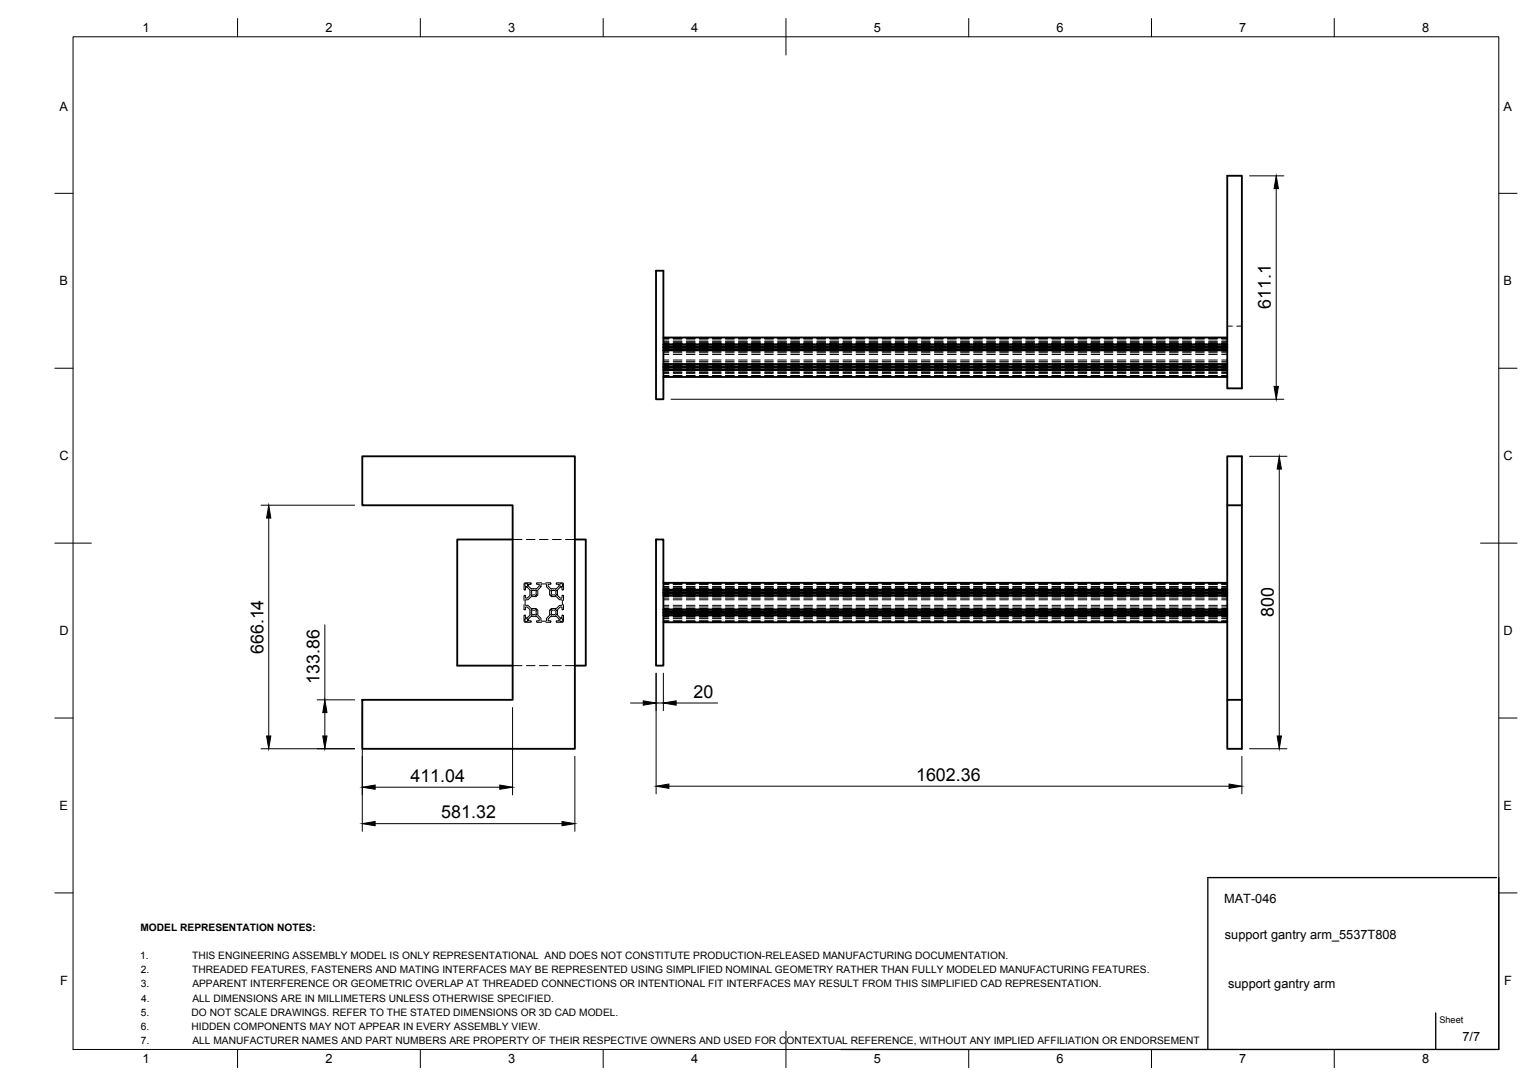
ISO-10303-21;
HEADER;
/* Generated by software containing ST-Developer
 * from STEP Tools, Inc. (www.steptools.com) 
 */

FILE_DESCRIPTION(
/* description */ ('STEP AP214'),
/* implementation_level */ '2;1');

FILE_NAME(
/* name */ 'support gantry arm.step',
/* time_stamp */ '2026-11-14T22:16:48-08:00',
/* author */ (''),
/* organization */ (''),
/* preprocessor_version */ 'ST-DEVELOPER v20.2',
/* originating_system */ 'Autodesk Translation Framework v15.17.0.0',
/* authorisation */ '');

FILE_SCHEMA (('AUTOMOTIVE_DESIGN { 1 0 10303 214 3 1 1 }'));
ENDSEC;

DATA;
#10=MECHANICAL_DESIGN_GEOMETRIC_PRESENTATION_REPRESENTATION('',(#5500),#276462);
#35=ORIENTED_CLOSED_SHELL('',*,#98725,.F.);
#36=ORIENTED_CLOSED_SHELL('',*,#98726,.F.);
#37=ORIENTED_CLOSED_SHELL('',*,#98727,.F.);
#38=ORIENTED_CLOSED_SHELL('',*,#98728,.F.);
#39=ORIENTED_CLOSED_SHELL('',*,#98729,.F.);
#40=ORIENTED_CLOSED_SHELL('',*,#98730,.F.);
#41=ORIENTED_CLOSED_SHELL('',*,#98731,.F.);
#42=ORIENTED_CLOSED_SHELL('',*,#98732,.F.);
#43=ORIENTED_CLOSED_SHELL('',*,#98733,.F.);
#44=BREP_WITH_VOIDS('Body1',#98734,(#35,#36,#37,#38,#39,#40,#41,#42,#43));
#5465=SHAPE_REPRESENTATION_RELATIONSHIP('SRR','None',#276493,#5471);
#5471=ADVANCED_BREP_SHAPE_REPRESENTATION('',(#44),#276461);
#5500=STYLED_ITEM('',(#276527),#44);
#6444=FACE_BOUND('',#19950,.T.);
#6445=FACE_BOUND('',#19956,.T.);
#7354=PLANE('',#110990);
#7355=PLANE('',#110998);
#7356=PLANE('',#110999);
#7357=PLANE('',#111002);
#7358=PLANE('',#111005);
#7359=PLANE('',#111008);
#7360=PLANE('',#111011);
#7361=PLANE('',#111014);
#7362=PLANE('',#111017);
#7363=PLANE('',#111020);
#7364=PLANE('',#111021);
#7365=PLANE('',#111026);
#7366=PLANE('',#111029);
#7367=PLANE('',#111032);
#7368=PLANE('',#111035);
#7369=PLANE('',#111038);
#7370=PLANE('',#111039);
#7371=PLANE('',#111064);
#7372=PLANE('',#111090);
#7373=PLANE('',#111092);
#7374=PLANE('',#111094);
#7375=PLANE('',#111095);
#7376=PLANE('',#111096);
#7377=PLANE('',#111098);
#7378=PLANE('',#111100);
#7379=PLANE('',#111102);
#7380=PLANE('',#111104);
#7381=PLANE('',#111106);
#7382=PLANE('',#111108);
#7383=PLANE('',#111109);
#7384=PLANE('',#111110);
#7385=PLANE('',#111112);
#7386=PLANE('',#111114);
#7387=PLANE('',#111116);
#7388=PLANE('',#111118);
#7389=PLANE('',#111120);
#7390=PLANE('',#111122);
#7391=PLANE('',#111123);
#7392=PLANE('',#111124);
#7393=PLANE('',#111126);
#7394=PLANE('',#111128);
#7395=PLANE('',#111130);
#7396=PLANE('',#111132);
#7397=PLANE('',#111134);
#7398=PLANE('',#111136);
#7399=PLANE('',#111137);
#7400=PLANE('',#111138);
#7401=PLANE('',#111140);
#7402=PLANE('',#111142);
#7403=PLANE('',#111144);
#7404=PLANE('',#111148);
#7405=PLANE('',#111156);
#7406=PLANE('',#111159);
#7407=PLANE('',#111162);
#7408=PLANE('',#111165);
#7409=PLANE('',#111168);
#7410=PLANE('',#111169);
#7411=PLANE('',#111172);
#7412=PLANE('',#111175);
#7413=PLANE('',#111178);
#7414=PLANE('',#111179);
#7415=PLANE('',#111184);
#7416=PLANE('',#111187);
#7417=PLANE('',#111190);
#7418=PLANE('',#111193);
#7419=PLANE('',#111196);
#7420=PLANE('',#111200);
#7421=PLANE('',#111208);
#7422=PLANE('',#111211);
#7423=PLANE('',#111214);
#7424=PLANE('',#111217);
#7425=PLANE('',#111220);
#7426=PLANE('',#111223);
#7427=PLANE('',#111226);
#7428=PLANE('',#111227);
#7429=PLANE('',#111230);
#7430=PLANE('',#111231);
#7431=PLANE('',#111236);
#7432=PLANE('',#111239);
#7433=PLANE('',#111242);
#7434=PLANE('',#111245);
#7435=PLANE('',#111248);
#7436=PLANE('',#111252);
#7437=PLANE('',#111260);
#7438=PLANE('',#111263);
#7439=PLANE('',#111266);
#7440=PLANE('',#111269);
#7441=PLANE('',#111272);
#7442=PLANE('',#111275);
#7443=PLANE('',#111278);
#7444=PLANE('',#111279);
#7445=PLANE('',#111282);
#7446=PLANE('',#111283);
#7447=PLANE('',#111288);
#7448=PLANE('',#111291);
#7449=PLANE('',#111294);
#7450=PLANE('',#111297);
#7451=PLANE('',#111300);
#7452=PLANE('',#111301);
#7453=PLANE('',#111302);
#7454=PLANE('',#111303);
#7455=PLANE('',#111304);
#7456=PLANE('',#111305);
#7457=PLANE('',#111309);
#7458=PLANE('',#111313);
#7459=PLANE('',#111317);
#7460=PLANE('',#111321);
#7461=PLANE('',#111322);
#7462=PLANE('',#111323);
#7463=PLANE('',#111324);
#7464=PLANE('',#111325);
#7465=PLANE('',#111326);
#7466=PLANE('',#111327);
#7467=PLANE('',#111328);
#7468=PLANE('',#111332);
#7469=PLANE('',#111336);
#7470=PLANE('',#111340);
#7471=PLANE('',#111344);
#7472=PLANE('',#111345);
#7473=PLANE('',#111346);
#7474=PLANE('',#111347);
#7475=PLANE('',#111351);
#7476=PLANE('',#111355);
#7477=PLANE('',#111359);
#7478=PLANE('',#111363);
#7479=PLANE('',#111364);
#7480=PLANE('',#111365);
#7481=PLANE('',#111366);
#7482=PLANE('',#111370);
#7483=PLANE('',#111371);
#7484=PLANE('',#111372);
#7485=PLANE('',#111373);
#7486=PLANE('',#111377);
#7487=PLANE('',#111381);
#7488=PLANE('',#111385);
#7489=PLANE('',#111389);
#7490=PLANE('',#111390);
#7491=PLANE('',#111391);
#7492=PLANE('',#111392);
#7493=PLANE('',#111396);
#7494=PLANE('',#111400);
#7495=PLANE('',#111404);
#7496=PLANE('',#111408);
#7497=PLANE('',#111409);
#7498=PLANE('',#111410);
#7499=PLANE('',#111411);
#7500=PLANE('',#111412);
#7501=PLANE('',#111413);
#7502=PLANE('',#111414);
#7503=PLANE('',#111418);
#7504=PLANE('',#111422);
#7505=PLANE('',#111426);
#7506=PLANE('',#111430);
#7507=PLANE('',#111431);
#7508=PLANE('',#111432);
#7509=PLANE('',#111433);
#7510=PLANE('',#111437);
#7511=PLANE('',#111441);
#7512=PLANE('',#111445);
#7513=PLANE('',#111449);
#7514=PLANE('',#111450);
#7515=PLANE('',#111451);
#7516=PLANE('',#111452);
#7517=PLANE('',#111456);
#7518=PLANE('',#111457);
#7519=PLANE('',#111458);
#7520=PLANE('',#111459);
#7521=PLANE('',#111463);
#7522=PLANE('',#111467);
#7523=PLANE('',#111471);
#7524=PLANE('',#111475);
#7525=PLANE('',#111476);
#7526=PLANE('',#111477);
#7527=PLANE('',#111478);
#7528=PLANE('',#111482);
#7529=PLANE('',#111486);
#7530=PLANE('',#111490);
#7531=PLANE('',#111494);
#7532=PLANE('',#111495);
#7533=PLANE('',#111496);
#7534=PLANE('',#111497);
#7535=PLANE('',#111498);
#7536=PLANE('',#111499);
#7537=PLANE('',#111500);
#7538=PLANE('',#111504);
#7539=PLANE('',#111508);
#7540=PLANE('',#111512);
#7541=PLANE('',#111516);
#7542=PLANE('',#111517);
#7543=PLANE('',#111518);
#7544=PLANE('',#111519);
#7545=PLANE('',#111523);
#7546=PLANE('',#111527);
#7547=PLANE('',#111531);
#7548=PLANE('',#111535);
#7549=PLANE('',#111536);
#7550=PLANE('',#111537);
#7551=PLANE('',#111538);
#7552=PLANE('',#111542);
#7553=PLANE('',#111543);
#7554=PLANE('',#111544);
#7555=PLANE('',#111545);
#7556=PLANE('',#111549);
#7557=PLANE('',#111553);
#7558=PLANE('',#111557);
#7559=PLANE('',#111561);
#7560=PLANE('',#111562);
#7561=PLANE('',#111563);
#7562=PLANE('',#111564);
#7563=PLANE('',#111568);
#7564=PLANE('',#111572);
#7565=PLANE('',#111576);
#7566=PLANE('',#111580);
#7567=PLANE('',#111581);
#7568=PLANE('',#111582);
#7569=PLANE('',#111583);
#7570=PLANE('',#111584);
#7571=PLANE('',#111585);
#7572=PLANE('',#111589);
#7573=PLANE('',#111593);
#7574=PLANE('',#111597);
#7575=PLANE('',#111601);
#7576=PLANE('',#111602);
#7577=PLANE('',#111603);
#7578=PLANE('',#111604);
#7579=PLANE('',#111608);
#7580=PLANE('',#111612);
#7581=PLANE('',#111616);
#7582=PLANE('',#111620);
#7583=PLANE('',#111621);
#7584=PLANE('',#111622);
#7585=PLANE('',#111623);
#7586=PLANE('',#111627);
#7587=PLANE('',#111628);
#7588=PLANE('',#111629);
#7589=PLANE('',#111630);
#7590=PLANE('',#111634);
#7591=PLANE('',#111638);
#7592=PLANE('',#111642);
#7593=PLANE('',#111646);
#7594=PLANE('',#111647);
#7595=PLANE('',#111648);
#7596=PLANE('',#111649);
#7597=PLANE('',#111650);
#7598=PLANE('',#111651);
#7599=PLANE('',#111652);
#7600=PLANE('',#111653);
#7601=PLANE('',#111654);
#7602=PLANE('',#111655);
#7603=PLANE('',#111656);
#7604=PLANE('',#111657);
#7605=PLANE('',#111658);
#7606=PLANE('',#111659);
#7607=PLANE('',#111660);
#7608=PLANE('',#111661);
#7609=PLANE('',#111662);
#7610=PLANE('',#111663);
#7611=PLANE('',#111664);
#7612=PLANE('',#111665);
#7613=PLANE('',#111666);
#13324=FACE_OUTER_BOUND('',#19556,.T.);
#13325=FACE_OUTER_BOUND('',#19557,.T.);
#13326=FACE_OUTER_BOUND('',#19558,.T.);
#13327=FACE_OUTER_BOUND('',#19559,.T.);
#13328=FACE_OUTER_BOUND('',#19560,.T.);
#13329=FACE_OUTER_BOUND('',#19561,.T.);
#13330=FACE_OUTER_BOUND('',#19562,.T.);
#13331=FACE_OUTER_BOUND('',#19563,.T.);
#13332=FACE_OUTER_BOUND('',#19564,.T.);
#13333=FACE_OUTER_BOUND('',#19565,.T.);
#13334=FACE_OUTER_BOUND('',#19566,.T.);
#13335=FACE_OUTER_BOUND('',#19567,.T.);
#13336=FACE_OUTER_BOUND('',#19568,.T.);
#13337=FACE_OUTER_BOUND('',#19569,.T.);
#13338=FACE_OUTER_BOUND('',#19570,.T.);
#13339=FACE_OUTER_BOUND('',#19571,.T.);
#13340=FACE_OUTER_BOUND('',#19572,.T.);
#13341=FACE_OUTER_BOUND('',#19573,.T.);
#13342=FACE_OUTER_BOUND('',#19574,.T.);
#13343=FACE_OUTER_BOUND('',#19575,.T.);
#13344=FACE_OUTER_BOUND('',#19576,.T.);
#13345=FACE_OUTER_BOUND('',#19577,.T.);
#13346=FACE_OUTER_BOUND('',#19578,.T.);
#13347=FACE_OUTER_BOUND('',#19579,.T.);
#13348=FACE_OUTER_BOUND('',#19580,.T.);
#13349=FACE_OUTER_BOUND('',#19581,.T.);
#13350=FACE_OUTER_BOUND('',#19582,.T.);
#13351=FACE_OUTER_BOUND('',#19583,.T.);
#13352=FACE_OUTER_BOUND('',#19584,.T.);
#13353=FACE_OUTER_BOUND('',#19585,.T.);
#13354=FACE_OUTER_BOUND('',#19586,.T.);
#13355=FACE_OUTER_BOUND('',#19587,.T.);
#13356=FACE_OUTER_BOUND('',#19588,.T.);
#13357=FACE_OUTER_BOUND('',#19589,.T.);
#13358=FACE_OUTER_BOUND('',#19590,.T.);
#13359=FACE_OUTER_BOUND('',#19591,.T.);
#13360=FACE_OUTER_BOUND('',#19592,.T.);
#13361=FACE_OUTER_BOUND('',#19593,.T.);
#13362=FACE_OUTER_BOUND('',#19594,.T.);
#13363=FACE_OUTER_BOUND('',#19595,.T.);
#13364=FACE_OUTER_BOUND('',#19596,.T.);
#13365=FACE_OUTER_BOUND('',#19597,.T.);
#13366=FACE_OUTER_BOUND('',#19598,.T.);
#13367=FACE_OUTER_BOUND('',#19599,.T.);
#13368=FACE_OUTER_BOUND('',#19600,.T.);
#13369=FACE_OUTER_BOUND('',#19601,.T.);
#13370=FACE_OUTER_BOUND('',#19602,.T.);
#13371=FACE_OUTER_BOUND('',#19603,.T.);
#13372=FACE_OUTER_BOUND('',#19604,.T.);
#13373=FACE_OUTER_BOUND('',#19605,.T.);
#13374=FACE_OUTER_BOUND('',#19606,.T.);
#13375=FACE_OUTER_BOUND('',#19607,.T.);
#13376=FACE_OUTER_BOUND('',#19608,.T.);
#13377=FACE_OUTER_BOUND('',#19609,.T.);
#13378=FACE_OUTER_BOUND('',#19610,.T.);
#13379=FACE_OUTER_BOUND('',#19611,.T.);
#13380=FACE_OUTER_BOUND('',#19612,.T.);
#13381=FACE_OUTER_BOUND('',#19613,.T.);
#13382=FACE_OUTER_BOUND('',#19614,.T.);
#13383=FACE_OUTER_BOUND('',#19615,.T.);
#13384=FACE_OUTER_BOUND('',#19616,.T.);
#13385=FACE_OUTER_BOUND('',#19617,.T.);
#13386=FACE_OUTER_BOUND('',#19618,.T.);
#13387=FACE_OUTER_BOUND('',#19619,.T.);
#13388=FACE_OUTER_BOUND('',#19620,.T.);
#13389=FACE_OUTER_BOUND('',#19621,.T.);
#13390=FACE_OUTER_BOUND('',#19622,.T.);
#13391=FACE_OUTER_BOUND('',#19623,.T.);
#13392=FACE_OUTER_BOUND('',#19624,.T.);
#13393=FACE_OUTER_BOUND('',#19625,.T.);
#13394=FACE_OUTER_BOUND('',#19626,.T.);
#13395=FACE_OUTER_BOUND('',#19627,.T.);
#13396=FACE_OUTER_BOUND('',#19628,.T.);
#13397=FACE_OUTER_BOUND('',#19629,.T.);
#13398=FACE_OUTER_BOUND('',#19630,.T.);
#13399=FACE_OUTER_BOUND('',#19631,.T.);
#13400=FACE_OUTER_BOUND('',#19632,.T.);
#13401=FACE_OUTER_BOUND('',#19633,.T.);
#13402=FACE_OUTER_BOUND('',#19634,.T.);
#13403=FACE_OUTER_BOUND('',#19635,.T.);
#13404=FACE_OUTER_BOUND('',#19636,.T.);
#13405=FACE_OUTER_BOUND('',#19637,.T.);
#13406=FACE_OUTER_BOUND('',#19638,.T.);
#13407=FACE_OUTER_BOUND('',#19639,.T.);
#13408=FACE_OUTER_BOUND('',#19640,.T.);
#13409=FACE_OUTER_BOUND('',#19641,.T.);
#13410=FACE_OUTER_BOUND('',#19642,.T.);
#13411=FACE_OUTER_BOUND('',#19643,.T.);
#13412=FACE_OUTER_BOUND('',#19644,.T.);
#13413=FACE_OUTER_BOUND('',#19645,.T.);
#13414=FACE_OUTER_BOUND('',#19646,.T.);
#13415=FACE_OUTER_BOUND('',#19647,.T.);
#13416=FACE_OUTER_BOUND('',#19648,.T.);
#13417=FACE_OUTER_BOUND('',#19649,.T.);
#13418=FACE_OUTER_BOUND('',#19650,.T.);
#13419=FACE_OUTER_BOUND('',#19651,.T.);
#13420=FACE_OUTER_BOUND('',#19652,.T.);
#13421=FACE_OUTER_BOUND('',#19653,.T.);
#13422=FACE_OUTER_BOUND('',#19654,.T.);
#13423=FACE_OUTER_BOUND('',#19655,.T.);
#13424=FACE_OUTER_BOUND('',#19656,.T.);
#13425=FACE_OUTER_BOUND('',#19657,.T.);
#13426=FACE_OUTER_BOUND('',#19658,.T.);
#13427=FACE_OUTER_BOUND('',#19659,.T.);
#13428=FACE_OUTER_BOUND('',#19660,.T.);
#13429=FACE_OUTER_BOUND('',#19661,.T.);
#13430=FACE_OUTER_BOUND('',#19662,.T.);
#13431=FACE_OUTER_BOUND('',#19663,.T.);
#13432=FACE_OUTER_BOUND('',#19664,.T.);
#13433=FACE_OUTER_BOUND('',#19665,.T.);
#13434=FACE_OUTER_BOUND('',#19666,.T.);
#13435=FACE_OUTER_BOUND('',#19667,.T.);
#13436=FACE_OUTER_BOUND('',#19668,.T.);
#13437=FACE_OUTER_BOUND('',#19669,.T.);
#13438=FACE_OUTER_BOUND('',#19670,.T.);
#13439=FACE_OUTER_BOUND('',#19671,.T.);
#13440=FACE_OUTER_BOUND('',#19672,.T.);
#13441=FACE_OUTER_BOUND('',#19673,.T.);
#13442=FACE_OUTER_BOUND('',#19674,.T.);
#13443=FACE_OUTER_BOUND('',#19675,.T.);
#13444=FACE_OUTER_BOUND('',#19676,.T.);
#13445=FACE_OUTER_BOUND('',#19677,.T.);
#13446=FACE_OUTER_BOUND('',#19678,.T.);
#13447=FACE_OUTER_BOUND('',#19679,.T.);
#13448=FACE_OUTER_BOUND('',#19680,.T.);
#13449=FACE_OUTER_BOUND('',#19681,.T.);
#13450=FACE_OUTER_BOUND('',#19682,.T.);
#13451=FACE_OUTER_BOUND('',#19683,.T.);
#13452=FACE_OUTER_BOUND('',#19684,.T.);
#13453=FACE_OUTER_BOUND('',#19685,.T.);
#13454=FACE_OUTER_BOUND('',#19686,.T.);
#13455=FACE_OUTER_BOUND('',#19687,.T.);
#13456=FACE_OUTER_BOUND('',#19688,.T.);
#13457=FACE_OUTER_BOUND('',#19689,.T.);
#13458=FACE_OUTER_BOUND('',#19690,.T.);
#13459=FACE_OUTER_BOUND('',#19691,.T.);
#13460=FACE_OUTER_BOUND('',#19692,.T.);
#13461=FACE_OUTER_BOUND('',#19693,.T.);
#13462=FACE_OUTER_BOUND('',#19694,.T.);
#13463=FACE_OUTER_BOUND('',#19695,.T.);
#13464=FACE_OUTER_BOUND('',#19696,.T.);
#13465=FACE_OUTER_BOUND('',#19697,.T.);
#13466=FACE_OUTER_BOUND('',#19698,.T.);
#13467=FACE_OUTER_BOUND('',#19699,.T.);
#13468=FACE_OUTER_BOUND('',#19700,.T.);
#13469=FACE_OUTER_BOUND('',#19701,.T.);
#13470=FACE_OUTER_BOUND('',#19702,.T.);
#13471=FACE_OUTER_BOUND('',#19703,.T.);
#13472=FACE_OUTER_BOUND('',#19704,.T.);
#13473=FACE_OUTER_BOUND('',#19705,.T.);
#13474=FACE_OUTER_BOUND('',#19706,.T.);
#13475=FACE_OUTER_BOUND('',#19707,.T.);
#13476=FACE_OUTER_BOUND('',#19708,.T.);
#13477=FACE_OUTER_BOUND('',#19709,.T.);
#13478=FACE_OUTER_BOUND('',#19710,.T.);
#13479=FACE_OUTER_BOUND('',#19711,.T.);
#13480=FACE_OUTER_BOUND('',#19712,.T.);
#13481=FACE_OUTER_BOUND('',#19713,.T.);
#13482=FACE_OUTER_BOUND('',#19714,.T.);
#13483=FACE_OUTER_BOUND('',#19715,.T.);
#13484=FACE_OUTER_BOUND('',#19716,.T.);
#13485=FACE_OUTER_BOUND('',#19717,.T.);
#13486=FACE_OUTER_BOUND('',#19718,.T.);
#13487=FACE_OUTER_BOUND('',#19719,.T.);
#13488=FACE_OUTER_BOUND('',#19720,.T.);
#13489=FACE_OUTER_BOUND('',#19721,.T.);
#13490=FACE_OUTER_BOUND('',#19722,.T.);
#13491=FACE_OUTER_BOUND('',#19723,.T.);
#13492=FACE_OUTER_BOUND('',#19724,.T.);
#13493=FACE_OUTER_BOUND('',#19725,.T.);
#13494=FACE_OUTER_BOUND('',#19726,.T.);
#13495=FACE_OUTER_BOUND('',#19727,.T.);
#13496=FACE_OUTER_BOUND('',#19728,.T.);
#13497=FACE_OUTER_BOUND('',#19729,.T.);
#13498=FACE_OUTER_BOUND('',#19730,.T.);
#13499=FACE_OUTER_BOUND('',#19731,.T.);
#13500=FACE_OUTER_BOUND('',#19732,.T.);
#13501=FACE_OUTER_BOUND('',#19733,.T.);
#13502=FACE_OUTER_BOUND('',#19734,.T.);
#13503=FACE_OUTER_BOUND('',#19735,.T.);
#13504=FACE_OUTER_BOUND('',#19736,.T.);
#13505=FACE_OUTER_BOUND('',#19737,.T.);
#13506=FACE_OUTER_BOUND('',#19738,.T.);
#13507=FACE_OUTER_BOUND('',#19739,.T.);
#13508=FACE_OUTER_BOUND('',#19740,.T.);
#13509=FACE_OUTER_BOUND('',#19741,.T.);
#13510=FACE_OUTER_BOUND('',#19742,.T.);
#13511=FACE_OUTER_BOUND('',#19743,.T.);
#13512=FACE_OUTER_BOUND('',#19744,.T.);
#13513=FACE_OUTER_BOUND('',#19745,.T.);
#13514=FACE_OUTER_BOUND('',#19746,.T.);
#13515=FACE_OUTER_BOUND('',#19747,.T.);
#13516=FACE_OUTER_BOUND('',#19748,.T.);
#13517=FACE_OUTER_BOUND('',#19749,.T.);
#13518=FACE_OUTER_BOUND('',#19750,.T.);
#13519=FACE_OUTER_BOUND('',#19751,.T.);
#13520=FACE_OUTER_BOUND('',#19752,.T.);
#13521=FACE_OUTER_BOUND('',#19753,.T.);
#13522=FACE_OUTER_BOUND('',#19754,.T.);
#13523=FACE_OUTER_BOUND('',#19755,.T.);
#13524=FACE_OUTER_BOUND('',#19756,.T.);
#13525=FACE_OUTER_BOUND('',#19757,.T.);
#13526=FACE_OUTER_BOUND('',#19758,.T.);
#13527=FACE_OUTER_BOUND('',#19759,.T.);
#13528=FACE_OUTER_BOUND('',#19760,.T.);
#13529=FACE_OUTER_BOUND('',#19761,.T.);
#13530=FACE_OUTER_BOUND('',#19762,.T.);
#13531=FACE_OUTER_BOUND('',#19763,.T.);
#13532=FACE_OUTER_BOUND('',#19764,.T.);
#13533=FACE_OUTER_BOUND('',#19765,.T.);
#13534=FACE_OUTER_BOUND('',#19766,.T.);
#13535=FACE_OUTER_BOUND('',#19767,.T.);
#13536=FACE_OUTER_BOUND('',#19768,.T.);
#13537=FACE_OUTER_BOUND('',#19769,.T.);
#13538=FACE_OUTER_BOUND('',#19770,.T.);
#13539=FACE_OUTER_BOUND('',#19771,.T.);
#13540=FACE_OUTER_BOUND('',#19772,.T.);
#13541=FACE_OUTER_BOUND('',#19773,.T.);
#13542=FACE_OUTER_BOUND('',#19774,.T.);
#13543=FACE_OUTER_BOUND('',#19775,.T.);
#13544=FACE_OUTER_BOUND('',#19776,.T.);
#13545=FACE_OUTER_BOUND('',#19777,.T.);
#13546=FACE_OUTER_BOUND('',#19778,.T.);
#13547=FACE_OUTER_BOUND('',#19779,.T.);
#13548=FACE_OUTER_BOUND('',#19780,.T.);
#13549=FACE_OUTER_BOUND('',#19781,.T.);
#13550=FACE_OUTER_BOUND('',#19782,.T.);
#13551=FACE_OUTER_BOUND('',#19783,.T.);
#13552=FACE_OUTER_BOUND('',#19784,.T.);
#13553=FACE_OUTER_BOUND('',#19785,.T.);
#13554=FACE_OUTER_BOUND('',#19786,.T.);
#13555=FACE_OUTER_BOUND('',#19787,.T.);
#13556=FACE_OUTER_BOUND('',#19788,.T.);
#13557=FACE_OUTER_BOUND('',#19789,.T.);
#13558=FACE_OUTER_BOUND('',#19790,.T.);
#13559=FACE_OUTER_BOUND('',#19791,.T.);
#13560=FACE_OUTER_BOUND('',#19792,.T.);
#13561=FACE_OUTER_BOUND('',#19793,.T.);
#13562=FACE_OUTER_BOUND('',#19794,.T.);
#13563=FACE_OUTER_BOUND('',#19795,.T.);
#13564=FACE_OUTER_BOUND('',#19796,.T.);
#13565=FACE_OUTER_BOUND('',#19797,.T.);
#13566=FACE_OUTER_BOUND('',#19798,.T.);
#13567=FACE_OUTER_BOUND('',#19799,.T.);
#13568=FACE_OUTER_BOUND('',#19800,.T.);
#13569=FACE_OUTER_BOUND('',#19801,.T.);
#13570=FACE_OUTER_BOUND('',#19802,.T.);
#13571=FACE_OUTER_BOUND('',#19803,.T.);
#13572=FACE_OUTER_BOUND('',#19804,.T.);
#13573=FACE_OUTER_BOUND('',#19805,.T.);
#13574=FACE_OUTER_BOUND('',#19806,.T.);
#13575=FACE_OUTER_BOUND('',#19807,.T.);
#13576=FACE_OUTER_BOUND('',#19808,.T.);
#13577=FACE_OUTER_BOUND('',#19809,.T.);
#13578=FACE_OUTER_BOUND('',#19810,.T.);
#13579=FACE_OUTER_BOUND('',#19811,.T.);
#13580=FACE_OUTER_BOUND('',#19812,.T.);
#13581=FACE_OUTER_BOUND('',#19813,.T.);
#13582=FACE_OUTER_BOUND('',#19814,.T.);
#13583=FACE_OUTER_BOUND('',#19815,.T.);
#13584=FACE_OUTER_BOUND('',#19816,.T.);
#13585=FACE_OUTER_BOUND('',#19817,.T.);
#13586=FACE_OUTER_BOUND('',#19818,.T.);
#13587=FACE_OUTER_BOUND('',#19819,.T.);
#13588=FACE_OUTER_BOUND('',#19820,.T.);
#13589=FACE_OUTER_BOUND('',#19821,.T.);
#13590=FACE_OUTER_BOUND('',#19822,.T.);
#13591=FACE_OUTER_BOUND('',#19823,.T.);
#13592=FACE_OUTER_BOUND('',#19824,.T.);
#13593=FACE_OUTER_BOUND('',#19825,.T.);
#13594=FACE_OUTER_BOUND('',#19826,.T.);
#13595=FACE_OUTER_BOUND('',#19827,.T.);
#13596=FACE_OUTER_BOUND('',#19828,.T.);
#13597=FACE_OUTER_BOUND('',#19829,.T.);
#13598=FACE_OUTER_BOUND('',#19830,.T.);
#13599=FACE_OUTER_BOUND('',#19831,.T.);
#13600=FACE_OUTER_BOUND('',#19832,.T.);
#13601=FACE_OUTER_BOUND('',#19833,.T.);
#13602=FACE_OUTER_BOUND('',#19834,.T.);
#13603=FACE_OUTER_BOUND('',#19835,.T.);
#13604=FACE_OUTER_BOUND('',#19836,.T.);
#13605=FACE_OUTER_BOUND('',#19837,.T.);
#13606=FACE_OUTER_BOUND('',#19838,.T.);
#13607=FACE_OUTER_BOUND('',#19839,.T.);
#13608=FACE_OUTER_BOUND('',#19840,.T.);
#13609=FACE_OUTER_BOUND('',#19841,.T.);
#13610=FACE_OUTER_BOUND('',#19842,.T.);
#13611=FACE_OUTER_BOUND('',#19843,.T.);
#13612=FACE_OUTER_BOUND('',#19844,.T.);
#13613=FACE_OUTER_BOUND('',#19845,.T.);
#13614=FACE_OUTER_BOUND('',#19846,.T.);
#13615=FACE_OUTER_BOUND('',#19847,.T.);
#13616=FACE_OUTER_BOUND('',#19848,.T.);
#13617=FACE_OUTER_BOUND('',#19849,.T.);
#13618=FACE_OUTER_BOUND('',#19850,.T.);
#13619=FACE_OUTER_BOUND('',#19851,.T.);
#13620=FACE_OUTER_BOUND('',#19852,.T.);
#13621=FACE_OUTER_BOUND('',#19853,.T.);
#13622=FACE_OUTER_BOUND('',#19854,.T.);
#13623=FACE_OUTER_BOUND('',#19855,.T.);
#13624=FACE_OUTER_BOUND('',#19856,.T.);
#13625=FACE_OUTER_BOUND('',#19857,.T.);
#13626=FACE_OUTER_BOUND('',#19858,.T.);
#13627=FACE_OUTER_BOUND('',#19859,.T.);
#13628=FACE_OUTER_BOUND('',#19860,.T.);
#13629=FACE_OUTER_BOUND('',#19861,.T.);
#13630=FACE_OUTER_BOUND('',#19862,.T.);
#13631=FACE_OUTER_BOUND('',#19863,.T.);
#13632=FACE_OUTER_BOUND('',#19864,.T.);
#13633=FACE_OUTER_BOUND('',#19865,.T.);
#13634=FACE_OUTER_BOUND('',#19866,.T.);
#13635=FACE_OUTER_BOUND('',#19867,.T.);
#13636=FACE_OUTER_BOUND('',#19868,.T.);
#13637=FACE_OUTER_BOUND('',#19869,.T.);
#13638=FACE_OUTER_BOUND('',#19870,.T.);
#13639=FACE_OUTER_BOUND('',#19871,.T.);
#13640=FACE_OUTER_BOUND('',#19872,.T.);
#13641=FACE_OUTER_BOUND('',#19873,.T.);
#13642=FACE_OUTER_BOUND('',#19874,.T.);
#13643=FACE_OUTER_BOUND('',#19875,.T.);
#13644=FACE_OUTER_BOUND('',#19876,.T.);
#13645=FACE_OUTER_BOUND('',#19877,.T.);
#13646=FACE_OUTER_BOUND('',#19878,.T.);
#13647=FACE_OUTER_BOUND('',#19879,.T.);
#13648=FACE_OUTER_BOUND('',#19880,.T.);
#13649=FACE_OUTER_BOUND('',#19881,.T.);
#13650=FACE_OUTER_BOUND('',#19882,.T.);
#13651=FACE_OUTER_BOUND('',#19883,.T.);
#13652=FACE_OUTER_BOUND('',#19884,.T.);
#13653=FACE_OUTER_BOUND('',#19885,.T.);
#13654=FACE_OUTER_BOUND('',#19886,.T.);
#13655=FACE_OUTER_BOUND('',#19887,.T.);
#13656=FACE_OUTER_BOUND('',#19888,.T.);
#13657=FACE_OUTER_BOUND('',#19889,.T.);
#13658=FACE_OUTER_BOUND('',#19890,.T.);
#13659=FACE_OUTER_BOUND('',#19891,.T.);
#13660=FACE_OUTER_BOUND('',#19892,.T.);
#13661=FACE_OUTER_BOUND('',#19893,.T.);
#13662=FACE_OUTER_BOUND('',#19894,.T.);
#13663=FACE_OUTER_BOUND('',#19895,.T.);
#13664=FACE_OUTER_BOUND('',#19896,.T.);
#13665=FACE_OUTER_BOUND('',#19897,.T.);
#13666=FACE_OUTER_BOUND('',#19898,.T.);
#13667=FACE_OUTER_BOUND('',#19899,.T.);
#13668=FACE_OUTER_BOUND('',#19900,.T.);
#13669=FACE_OUTER_BOUND('',#19901,.T.);
#13670=FACE_OUTER_BOUND('',#19902,.T.);
#13671=FACE_OUTER_BOUND('',#19903,.T.);
#13672=FACE_OUTER_BOUND('',#19904,.T.);
#13673=FACE_OUTER_BOUND('',#19905,.T.);
#13674=FACE_OUTER_BOUND('',#19906,.T.);
#13675=FACE_OUTER_BOUND('',#19907,.T.);
#13676=FACE_OUTER_BOUND('',#19908,.T.);
#13677=FACE_OUTER_BOUND('',#19909,.T.);
#13678=FACE_OUTER_BOUND('',#19910,.T.);
#13679=FACE_OUTER_BOUND('',#19911,.T.);
#13680=FACE_OUTER_BOUND('',#19912,.T.);
#13681=FACE_OUTER_BOUND('',#19913,.T.);
#13682=FACE_OUTER_BOUND('',#19914,.T.);
#13683=FACE_OUTER_BOUND('',#19915,.T.);
#13684=FACE_OUTER_BOUND('',#19916,.T.);
#13685=FACE_OUTER_BOUND('',#19917,.T.);
#13686=FACE_OUTER_BOUND('',#19918,.T.);
#13687=FACE_OUTER_BOUND('',#19919,.T.);
#13688=FACE_OUTER_BOUND('',#19920,.T.);
#13689=FACE_OUTER_BOUND('',#19921,.T.);
#13690=FACE_OUTER_BOUND('',#19922,.T.);
#13691=FACE_OUTER_BOUND('',#19923,.T.);
#13692=FACE_OUTER_BOUND('',#19924,.T.);
#13693=FACE_OUTER_BOUND('',#19925,.T.);
#13694=FACE_OUTER_BOUND('',#19926,.T.);
#13695=FACE_OUTER_BOUND('',#19927,.T.);
#13696=FACE_OUTER_BOUND('',#19928,.T.);
#13697=FACE_OUTER_BOUND('',#19929,.T.);
#13698=FACE_OUTER_BOUND('',#19930,.T.);
#13699=FACE_OUTER_BOUND('',#19931,.T.);
#13700=FACE_OUTER_BOUND('',#19932,.T.);
#13701=FACE_OUTER_BOUND('',#19933,.T.);
#13702=FACE_OUTER_BOUND('',#19934,.T.);
#13703=FACE_OUTER_BOUND('',#19935,.T.);
#13704=FACE_OUTER_BOUND('',#19936,.T.);
#13705=FACE_OUTER_BOUND('',#19937,.T.);
#13706=FACE_OUTER_BOUND('',#19938,.T.);
#13707=FACE_OUTER_BOUND('',#19939,.T.);
#13708=FACE_OUTER_BOUND('',#19940,.T.);
#13709=FACE_OUTER_BOUND('',#19941,.T.);
#13710=FACE_OUTER_BOUND('',#19942,.T.);
#13711=FACE_OUTER_BOUND('',#19943,.T.);
#13712=FACE_OUTER_BOUND('',#19944,.T.);
#13713=FACE_OUTER_BOUND('',#19945,.T.);
#13714=FACE_OUTER_BOUND('',#19946,.T.);
#13715=FACE_OUTER_BOUND('',#19947,.T.);
#13716=FACE_OUTER_BOUND('',#19948,.T.);
#13717=FACE_OUTER_BOUND('',#19949,.T.);
#13718=FACE_OUTER_BOUND('',#19951,.T.);
#13719=FACE_OUTER_BOUND('',#19952,.T.);
#13720=FACE_OUTER_BOUND('',#19953,.T.);
#13721=FACE_OUTER_BOUND('',#19954,.T.);
#13722=FACE_OUTER_BOUND('',#19955,.T.);
#13723=FACE_OUTER_BOUND('',#19957,.T.);
#19556=EDGE_LOOP('',(#88025,#88026,#88027,#88028));
#19557=EDGE_LOOP('',(#88029,#88030,#88031,#88032,#88033,#88034,#88035,#88036,
#88037,#88038,#88039,#88040,#88041,#88042,#88043,#88044));
#19558=EDGE_LOOP('',(#88045,#88046,#88047,#88048));
#19559=EDGE_LOOP('',(#88049,#88050,#88051,#88052));
#19560=EDGE_LOOP('',(#88053,#88054,#88055,#88056));
#19561=EDGE_LOOP('',(#88057,#88058,#88059,#88060));
#19562=EDGE_LOOP('',(#88061,#88062,#88063,#88064));
#19563=EDGE_LOOP('',(#88065,#88066,#88067,#88068));
#19564=EDGE_LOOP('',(#88069,#88070,#88071,#88072));
#19565=EDGE_LOOP('',(#88073,#88074,#88075,#88076));
#19566=EDGE_LOOP('',(#88077,#88078,#88079,#88080));
#19567=EDGE_LOOP('',(#88081,#88082,#88083,#88084));
#19568=EDGE_LOOP('',(#88085,#88086,#88087,#88088));
#19569=EDGE_LOOP('',(#88089,#88090,#88091,#88092));
#19570=EDGE_LOOP('',(#88093,#88094,#88095,#88096));
#19571=EDGE_LOOP('',(#88097,#88098,#88099,#88100));
#19572=EDGE_LOOP('',(#88101,#88102,#88103,#88104));
#19573=EDGE_LOOP('',(#88105,#88106,#88107,#88108,#88109,#88110,#88111,#88112,
#88113,#88114,#88115,#88116,#88117,#88118,#88119,#88120));
#19574=EDGE_LOOP('',(#88121,#88122,#88123,#88124,#88125,#88126,#88127,#88128));
#19575=EDGE_LOOP('',(#88129,#88130,#88131,#88132));
#19576=EDGE_LOOP('',(#88133,#88134,#88135,#88136));
#19577=EDGE_LOOP('',(#88137,#88138,#88139,#88140));
#19578=EDGE_LOOP('',(#88141,#88142,#88143,#88144));
#19579=EDGE_LOOP('',(#88145,#88146,#88147,#88148));
#19580=EDGE_LOOP('',(#88149,#88150,#88151,#88152));
#19581=EDGE_LOOP('',(#88153,#88154,#88155,#88156));
#19582=EDGE_LOOP('',(#88157,#88158,#88159,#88160));
#19583=EDGE_LOOP('',(#88161,#88162,#88163,#88164,#88165,#88166,#88167,#88168));
#19584=EDGE_LOOP('',(#88169,#88170,#88171,#88172,#88173,#88174,#88175,#88176,
#88177,#88178,#88179,#88180,#88181,#88182,#88183,#88184,#88185,#88186,#88187,
#88188,#88189,#88190,#88191,#88192,#88193,#88194,#88195,#88196,#88197,#88198,
#88199,#88200,#88201,#88202,#88203,#88204,#88205,#88206,#88207,#88208,#88209,
#88210,#88211,#88212,#88213,#88214,#88215,#88216,#88217,#88218,#88219,#88220,
#88221,#88222,#88223,#88224));
#19585=EDGE_LOOP('',(#88225,#88226,#88227,#88228,#88229,#88230,#88231,#88232,
#88233,#88234,#88235,#88236,#88237,#88238,#88239,#88240,#88241,#88242,#88243,
#88244,#88245,#88246,#88247,#88248,#88249,#88250,#88251,#88252,#88253,#88254,
#88255,#88256,#88257,#88258,#88259,#88260,#88261,#88262,#88263,#88264,#88265,
#88266,#88267,#88268,#88269,#88270,#88271,#88272,#88273,#88274,#88275,#88276,
#88277,#88278,#88279,#88280));
#19586=EDGE_LOOP('',(#88281,#88282,#88283,#88284));
#19587=EDGE_LOOP('',(#88285,#88286,#88287,#88288));
#19588=EDGE_LOOP('',(#88289,#88290,#88291,#88292));
#19589=EDGE_LOOP('',(#88293,#88294,#88295,#88296));
#19590=EDGE_LOOP('',(#88297,#88298,#88299,#88300));
#19591=EDGE_LOOP('',(#88301,#88302,#88303,#88304));
#19592=EDGE_LOOP('',(#88305,#88306,#88307,#88308));
#19593=EDGE_LOOP('',(#88309,#88310,#88311,#88312));
#19594=EDGE_LOOP('',(#88313,#88314,#88315,#88316));
#19595=EDGE_LOOP('',(#88317,#88318,#88319,#88320));
#19596=EDGE_LOOP('',(#88321,#88322,#88323,#88324));
#19597=EDGE_LOOP('',(#88325,#88326,#88327,#88328));
#19598=EDGE_LOOP('',(#88329,#88330,#88331,#88332));
#19599=EDGE_LOOP('',(#88333,#88334,#88335,#88336));
#19600=EDGE_LOOP('',(#88337,#88338,#88339,#88340));
#19601=EDGE_LOOP('',(#88341,#88342,#88343,#88344));
#19602=EDGE_LOOP('',(#88345,#88346,#88347,#88348));
#19603=EDGE_LOOP('',(#88349,#88350,#88351,#88352));
#19604=EDGE_LOOP('',(#88353,#88354,#88355,#88356));
#19605=EDGE_LOOP('',(#88357,#88358,#88359,#88360));
#19606=EDGE_LOOP('',(#88361,#88362,#88363,#88364));
#19607=EDGE_LOOP('',(#88365,#88366,#88367,#88368));
#19608=EDGE_LOOP('',(#88369,#88370,#88371,#88372));
#19609=EDGE_LOOP('',(#88373,#88374,#88375,#88376));
#19610=EDGE_LOOP('',(#88377,#88378,#88379,#88380));
#19611=EDGE_LOOP('',(#88381,#88382,#88383,#88384));
#19612=EDGE_LOOP('',(#88385,#88386,#88387,#88388));
#19613=EDGE_LOOP('',(#88389,#88390,#88391,#88392));
#19614=EDGE_LOOP('',(#88393,#88394,#88395,#88396));
#19615=EDGE_LOOP('',(#88397,#88398,#88399,#88400));
#19616=EDGE_LOOP('',(#88401,#88402,#88403,#88404));
#19617=EDGE_LOOP('',(#88405,#88406,#88407,#88408));
#19618=EDGE_LOOP('',(#88409,#88410,#88411,#88412));
#19619=EDGE_LOOP('',(#88413,#88414,#88415,#88416));
#19620=EDGE_LOOP('',(#88417,#88418,#88419,#88420));
#19621=EDGE_LOOP('',(#88421,#88422,#88423,#88424));
#19622=EDGE_LOOP('',(#88425,#88426,#88427,#88428));
#19623=EDGE_LOOP('',(#88429,#88430,#88431,#88432));
#19624=EDGE_LOOP('',(#88433,#88434,#88435,#88436));
#19625=EDGE_LOOP('',(#88437,#88438,#88439,#88440));
#19626=EDGE_LOOP('',(#88441,#88442,#88443,#88444));
#19627=EDGE_LOOP('',(#88445,#88446,#88447,#88448));
#19628=EDGE_LOOP('',(#88449,#88450,#88451,#88452));
#19629=EDGE_LOOP('',(#88453,#88454,#88455,#88456));
#19630=EDGE_LOOP('',(#88457,#88458,#88459,#88460));
#19631=EDGE_LOOP('',(#88461,#88462,#88463,#88464));
#19632=EDGE_LOOP('',(#88465,#88466,#88467,#88468));
#19633=EDGE_LOOP('',(#88469,#88470,#88471,#88472));
#19634=EDGE_LOOP('',(#88473,#88474,#88475,#88476));
#19635=EDGE_LOOP('',(#88477,#88478,#88479,#88480));
#19636=EDGE_LOOP('',(#88481,#88482,#88483,#88484));
#19637=EDGE_LOOP('',(#88485,#88486,#88487,#88488));
#19638=EDGE_LOOP('',(#88489,#88490,#88491,#88492));
#19639=EDGE_LOOP('',(#88493,#88494,#88495,#88496));
#19640=EDGE_LOOP('',(#88497,#88498,#88499,#88500));
#19641=EDGE_LOOP('',(#88501,#88502,#88503,#88504));
#19642=EDGE_LOOP('',(#88505,#88506,#88507,#88508));
#19643=EDGE_LOOP('',(#88509,#88510,#88511,#88512,#88513,#88514,#88515,#88516,
#88517,#88518,#88519,#88520,#88521,#88522,#88523,#88524));
#19644=EDGE_LOOP('',(#88525,#88526,#88527,#88528));
#19645=EDGE_LOOP('',(#88529,#88530,#88531,#88532));
#19646=EDGE_LOOP('',(#88533,#88534,#88535,#88536));
#19647=EDGE_LOOP('',(#88537,#88538,#88539,#88540));
#19648=EDGE_LOOP('',(#88541,#88542,#88543,#88544));
#19649=EDGE_LOOP('',(#88545,#88546,#88547,#88548));
#19650=EDGE_LOOP('',(#88549,#88550,#88551,#88552));
#19651=EDGE_LOOP('',(#88553,#88554,#88555,#88556));
#19652=EDGE_LOOP('',(#88557,#88558,#88559,#88560));
#19653=EDGE_LOOP('',(#88561,#88562,#88563,#88564));
#19654=EDGE_LOOP('',(#88565,#88566,#88567,#88568));
#19655=EDGE_LOOP('',(#88569,#88570,#88571,#88572));
#19656=EDGE_LOOP('',(#88573,#88574,#88575,#88576));
#19657=EDGE_LOOP('',(#88577,#88578,#88579,#88580));
#19658=EDGE_LOOP('',(#88581,#88582,#88583,#88584));
#19659=EDGE_LOOP('',(#88585,#88586,#88587,#88588,#88589,#88590,#88591,#88592,
#88593,#88594,#88595,#88596,#88597,#88598,#88599,#88600));
#19660=EDGE_LOOP('',(#88601,#88602,#88603,#88604,#88605,#88606,#88607,#88608));
#19661=EDGE_LOOP('',(#88609,#88610,#88611,#88612));
#19662=EDGE_LOOP('',(#88613,#88614,#88615,#88616));
#19663=EDGE_LOOP('',(#88617,#88618,#88619,#88620));
#19664=EDGE_LOOP('',(#88621,#88622,#88623,#88624));
#19665=EDGE_LOOP('',(#88625,#88626,#88627,#88628));
#19666=EDGE_LOOP('',(#88629,#88630,#88631,#88632));
#19667=EDGE_LOOP('',(#88633,#88634,#88635,#88636));
#19668=EDGE_LOOP('',(#88637,#88638,#88639,#88640));
#19669=EDGE_LOOP('',(#88641,#88642,#88643,#88644,#88645,#88646,#88647,#88648));
#19670=EDGE_LOOP('',(#88649,#88650,#88651,#88652));
#19671=EDGE_LOOP('',(#88653,#88654,#88655,#88656,#88657,#88658,#88659,#88660,
#88661,#88662,#88663,#88664,#88665,#88666,#88667,#88668));
#19672=EDGE_LOOP('',(#88669,#88670,#88671,#88672));
#19673=EDGE_LOOP('',(#88673,#88674,#88675,#88676));
#19674=EDGE_LOOP('',(#88677,#88678,#88679,#88680));
#19675=EDGE_LOOP('',(#88681,#88682,#88683,#88684));
#19676=EDGE_LOOP('',(#88685,#88686,#88687,#88688));
#19677=EDGE_LOOP('',(#88689,#88690,#88691,#88692));
#19678=EDGE_LOOP('',(#88693,#88694,#88695,#88696));
#19679=EDGE_LOOP('',(#88697,#88698,#88699,#88700));
#19680=EDGE_LOOP('',(#88701,#88702,#88703,#88704));
#19681=EDGE_LOOP('',(#88705,#88706,#88707,#88708));
#19682=EDGE_LOOP('',(#88709,#88710,#88711,#88712));
#19683=EDGE_LOOP('',(#88713,#88714,#88715,#88716));
#19684=EDGE_LOOP('',(#88717,#88718,#88719,#88720));
#19685=EDGE_LOOP('',(#88721,#88722,#88723,#88724));
#19686=EDGE_LOOP('',(#88725,#88726,#88727,#88728));
#19687=EDGE_LOOP('',(#88729,#88730,#88731,#88732,#88733,#88734,#88735,#88736,
#88737,#88738,#88739,#88740,#88741,#88742,#88743,#88744));
#19688=EDGE_LOOP('',(#88745,#88746,#88747,#88748,#88749,#88750,#88751,#88752));
#19689=EDGE_LOOP('',(#88753,#88754,#88755,#88756));
#19690=EDGE_LOOP('',(#88757,#88758,#88759,#88760));
#19691=EDGE_LOOP('',(#88761,#88762,#88763,#88764));
#19692=EDGE_LOOP('',(#88765,#88766,#88767,#88768));
#19693=EDGE_LOOP('',(#88769,#88770,#88771,#88772));
#19694=EDGE_LOOP('',(#88773,#88774,#88775,#88776));
#19695=EDGE_LOOP('',(#88777,#88778,#88779,#88780));
#19696=EDGE_LOOP('',(#88781,#88782,#88783,#88784));
#19697=EDGE_LOOP('',(#88785,#88786,#88787,#88788,#88789,#88790,#88791,#88792));
#19698=EDGE_LOOP('',(#88793,#88794,#88795,#88796));
#19699=EDGE_LOOP('',(#88797,#88798,#88799,#88800,#88801,#88802,#88803,#88804,
#88805,#88806,#88807,#88808,#88809,#88810,#88811,#88812));
#19700=EDGE_LOOP('',(#88813,#88814,#88815,#88816));
#19701=EDGE_LOOP('',(#88817,#88818,#88819,#88820));
#19702=EDGE_LOOP('',(#88821,#88822,#88823,#88824));
#19703=EDGE_LOOP('',(#88825,#88826,#88827,#88828));
#19704=EDGE_LOOP('',(#88829,#88830,#88831,#88832));
#19705=EDGE_LOOP('',(#88833,#88834,#88835,#88836));
#19706=EDGE_LOOP('',(#88837,#88838,#88839,#88840));
#19707=EDGE_LOOP('',(#88841,#88842,#88843,#88844));
#19708=EDGE_LOOP('',(#88845,#88846,#88847,#88848));
#19709=EDGE_LOOP('',(#88849,#88850,#88851,#88852));
#19710=EDGE_LOOP('',(#88853,#88854,#88855,#88856));
#19711=EDGE_LOOP('',(#88857,#88858,#88859,#88860));
#19712=EDGE_LOOP('',(#88861,#88862,#88863,#88864));
#19713=EDGE_LOOP('',(#88865,#88866,#88867,#88868));
#19714=EDGE_LOOP('',(#88869,#88870,#88871,#88872));
#19715=EDGE_LOOP('',(#88873,#88874,#88875,#88876,#88877,#88878,#88879,#88880,
#88881,#88882,#88883,#88884,#88885,#88886,#88887,#88888));
#19716=EDGE_LOOP('',(#88889,#88890,#88891,#88892,#88893,#88894,#88895,#88896));
#19717=EDGE_LOOP('',(#88897,#88898,#88899,#88900));
#19718=EDGE_LOOP('',(#88901,#88902,#88903,#88904));
#19719=EDGE_LOOP('',(#88905,#88906,#88907,#88908));
#19720=EDGE_LOOP('',(#88909,#88910,#88911,#88912));
#19721=EDGE_LOOP('',(#88913,#88914,#88915,#88916));
#19722=EDGE_LOOP('',(#88917,#88918,#88919,#88920));
#19723=EDGE_LOOP('',(#88921,#88922,#88923,#88924));
#19724=EDGE_LOOP('',(#88925,#88926,#88927,#88928));
#19725=EDGE_LOOP('',(#88929,#88930,#88931,#88932,#88933,#88934,#88935,#88936));
#19726=EDGE_LOOP('',(#88937,#88938,#88939,#88940));
#19727=EDGE_LOOP('',(#88941,#88942,#88943,#88944));
#19728=EDGE_LOOP('',(#88945,#88946,#88947,#88948));
#19729=EDGE_LOOP('',(#88949,#88950,#88951,#88952));
#19730=EDGE_LOOP('',(#88953,#88954,#88955,#88956));
#19731=EDGE_LOOP('',(#88957,#88958,#88959,#88960));
#19732=EDGE_LOOP('',(#88961,#88962,#88963,#88964));
#19733=EDGE_LOOP('',(#88965,#88966,#88967,#88968));
#19734=EDGE_LOOP('',(#88969,#88970,#88971,#88972));
#19735=EDGE_LOOP('',(#88973,#88974,#88975,#88976));
#19736=EDGE_LOOP('',(#88977,#88978,#88979,#88980));
#19737=EDGE_LOOP('',(#88981,#88982,#88983,#88984));
#19738=EDGE_LOOP('',(#88985,#88986,#88987,#88988));
#19739=EDGE_LOOP('',(#88989,#88990,#88991,#88992));
#19740=EDGE_LOOP('',(#88993,#88994,#88995,#88996));
#19741=EDGE_LOOP('',(#88997,#88998,#88999,#89000));
#19742=EDGE_LOOP('',(#89001,#89002,#89003,#89004));
#19743=EDGE_LOOP('',(#89005,#89006,#89007,#89008));
#19744=EDGE_LOOP('',(#89009,#89010,#89011,#89012));
#19745=EDGE_LOOP('',(#89013,#89014,#89015,#89016));
#19746=EDGE_LOOP('',(#89017,#89018,#89019,#89020));
#19747=EDGE_LOOP('',(#89021,#89022,#89023,#89024));
#19748=EDGE_LOOP('',(#89025,#89026,#89027,#89028));
#19749=EDGE_LOOP('',(#89029,#89030,#89031,#89032));
#19750=EDGE_LOOP('',(#89033,#89034,#89035,#89036));
#19751=EDGE_LOOP('',(#89037,#89038,#89039,#89040));
#19752=EDGE_LOOP('',(#89041,#89042,#89043,#89044));
#19753=EDGE_LOOP('',(#89045,#89046,#89047,#89048));
#19754=EDGE_LOOP('',(#89049,#89050,#89051,#89052));
#19755=EDGE_LOOP('',(#89053,#89054,#89055,#89056));
#19756=EDGE_LOOP('',(#89057,#89058,#89059,#89060));
#19757=EDGE_LOOP('',(#89061,#89062,#89063,#89064));
#19758=EDGE_LOOP('',(#89065,#89066,#89067,#89068));
#19759=EDGE_LOOP('',(#89069,#89070,#89071,#89072));
#19760=EDGE_LOOP('',(#89073,#89074,#89075,#89076));
#19761=EDGE_LOOP('',(#89077,#89078,#89079,#89080));
#19762=EDGE_LOOP('',(#89081,#89082,#89083,#89084));
#19763=EDGE_LOOP('',(#89085,#89086,#89087,#89088));
#19764=EDGE_LOOP('',(#89089,#89090,#89091,#89092));
#19765=EDGE_LOOP('',(#89093,#89094,#89095,#89096));
#19766=EDGE_LOOP('',(#89097,#89098,#89099,#89100));
#19767=EDGE_LOOP('',(#89101,#89102,#89103,#89104));
#19768=EDGE_LOOP('',(#89105,#89106,#89107,#89108));
#19769=EDGE_LOOP('',(#89109,#89110,#89111,#89112));
#19770=EDGE_LOOP('',(#89113,#89114,#89115,#89116));
#19771=EDGE_LOOP('',(#89117,#89118,#89119,#89120));
#19772=EDGE_LOOP('',(#89121,#89122,#89123,#89124));
#19773=EDGE_LOOP('',(#89125,#89126,#89127,#89128));
#19774=EDGE_LOOP('',(#89129,#89130,#89131,#89132));
#19775=EDGE_LOOP('',(#89133,#89134,#89135,#89136));
#19776=EDGE_LOOP('',(#89137,#89138,#89139,#89140));
#19777=EDGE_LOOP('',(#89141,#89142,#89143,#89144));
#19778=EDGE_LOOP('',(#89145,#89146,#89147,#89148));
#19779=EDGE_LOOP('',(#89149,#89150,#89151,#89152));
#19780=EDGE_LOOP('',(#89153,#89154,#89155,#89156));
#19781=EDGE_LOOP('',(#89157,#89158,#89159,#89160));
#19782=EDGE_LOOP('',(#89161,#89162,#89163,#89164));
#19783=EDGE_LOOP('',(#89165,#89166,#89167,#89168));
#19784=EDGE_LOOP('',(#89169,#89170,#89171,#89172));
#19785=EDGE_LOOP('',(#89173,#89174,#89175,#89176));
#19786=EDGE_LOOP('',(#89177,#89178,#89179,#89180));
#19787=EDGE_LOOP('',(#89181,#89182,#89183,#89184));
#19788=EDGE_LOOP('',(#89185,#89186,#89187,#89188));
#19789=EDGE_LOOP('',(#89189,#89190,#89191,#89192));
#19790=EDGE_LOOP('',(#89193,#89194,#89195,#89196));
#19791=EDGE_LOOP('',(#89197,#89198,#89199,#89200));
#19792=EDGE_LOOP('',(#89201,#89202,#89203,#89204));
#19793=EDGE_LOOP('',(#89205,#89206,#89207,#89208));
#19794=EDGE_LOOP('',(#89209,#89210,#89211,#89212));
#19795=EDGE_LOOP('',(#89213,#89214,#89215,#89216));
#19796=EDGE_LOOP('',(#89217,#89218,#89219,#89220));
#19797=EDGE_LOOP('',(#89221,#89222,#89223,#89224));
#19798=EDGE_LOOP('',(#89225,#89226,#89227,#89228));
#19799=EDGE_LOOP('',(#89229,#89230,#89231,#89232));
#19800=EDGE_LOOP('',(#89233,#89234,#89235,#89236));
#19801=EDGE_LOOP('',(#89237,#89238,#89239,#89240));
#19802=EDGE_LOOP('',(#89241,#89242,#89243,#89244));
#19803=EDGE_LOOP('',(#89245,#89246,#89247,#89248));
#19804=EDGE_LOOP('',(#89249,#89250,#89251,#89252));
#19805=EDGE_LOOP('',(#89253,#89254,#89255,#89256));
#19806=EDGE_LOOP('',(#89257,#89258,#89259,#89260));
#19807=EDGE_LOOP('',(#89261,#89262,#89263,#89264));
#19808=EDGE_LOOP('',(#89265,#89266,#89267,#89268));
#19809=EDGE_LOOP('',(#89269,#89270,#89271,#89272));
#19810=EDGE_LOOP('',(#89273,#89274,#89275,#89276));
#19811=EDGE_LOOP('',(#89277,#89278,#89279,#89280));
#19812=EDGE_LOOP('',(#89281,#89282,#89283,#89284));
#19813=EDGE_LOOP('',(#89285,#89286,#89287,#89288));
#19814=EDGE_LOOP('',(#89289,#89290,#89291,#89292));
#19815=EDGE_LOOP('',(#89293,#89294,#89295,#89296));
#19816=EDGE_LOOP('',(#89297,#89298,#89299,#89300));
#19817=EDGE_LOOP('',(#89301,#89302,#89303,#89304));
#19818=EDGE_LOOP('',(#89305,#89306,#89307,#89308));
#19819=EDGE_LOOP('',(#89309,#89310,#89311,#89312));
#19820=EDGE_LOOP('',(#89313,#89314,#89315,#89316));
#19821=EDGE_LOOP('',(#89317,#89318,#89319,#89320));
#19822=EDGE_LOOP('',(#89321,#89322,#89323,#89324));
#19823=EDGE_LOOP('',(#89325,#89326,#89327,#89328));
#19824=EDGE_LOOP('',(#89329,#89330,#89331,#89332));
#19825=EDGE_LOOP('',(#89333,#89334,#89335,#89336));
#19826=EDGE_LOOP('',(#89337,#89338,#89339,#89340));
#19827=EDGE_LOOP('',(#89341,#89342,#89343,#89344));
#19828=EDGE_LOOP('',(#89345,#89346,#89347,#89348));
#19829=EDGE_LOOP('',(#89349,#89350,#89351,#89352));
#19830=EDGE_LOOP('',(#89353,#89354,#89355,#89356));
#19831=EDGE_LOOP('',(#89357,#89358,#89359,#89360));
#19832=EDGE_LOOP('',(#89361,#89362,#89363,#89364));
#19833=EDGE_LOOP('',(#89365,#89366,#89367,#89368));
#19834=EDGE_LOOP('',(#89369,#89370,#89371,#89372));
#19835=EDGE_LOOP('',(#89373,#89374,#89375,#89376));
#19836=EDGE_LOOP('',(#89377,#89378,#89379,#89380));
#19837=EDGE_LOOP('',(#89381,#89382,#89383,#89384));
#19838=EDGE_LOOP('',(#89385,#89386,#89387,#89388));
#19839=EDGE_LOOP('',(#89389,#89390,#89391,#89392));
#19840=EDGE_LOOP('',(#89393,#89394,#89395,#89396));
#19841=EDGE_LOOP('',(#89397,#89398,#89399,#89400));
#19842=EDGE_LOOP('',(#89401,#89402,#89403,#89404));
#19843=EDGE_LOOP('',(#89405,#89406,#89407,#89408));
#19844=EDGE_LOOP('',(#89409,#89410,#89411,#89412));
#19845=EDGE_LOOP('',(#89413,#89414,#89415,#89416));
#19846=EDGE_LOOP('',(#89417,#89418,#89419,#89420));
#19847=EDGE_LOOP('',(#89421,#89422,#89423,#89424));
#19848=EDGE_LOOP('',(#89425,#89426,#89427,#89428));
#19849=EDGE_LOOP('',(#89429,#89430,#89431,#89432));
#19850=EDGE_LOOP('',(#89433,#89434,#89435,#89436));
#19851=EDGE_LOOP('',(#89437,#89438,#89439,#89440));
#19852=EDGE_LOOP('',(#89441,#89442,#89443,#89444));
#19853=EDGE_LOOP('',(#89445,#89446,#89447,#89448));
#19854=EDGE_LOOP('',(#89449,#89450,#89451,#89452));
#19855=EDGE_LOOP('',(#89453,#89454,#89455,#89456));
#19856=EDGE_LOOP('',(#89457,#89458,#89459,#89460));
#19857=EDGE_LOOP('',(#89461,#89462,#89463,#89464));
#19858=EDGE_LOOP('',(#89465,#89466,#89467,#89468));
#19859=EDGE_LOOP('',(#89469,#89470,#89471,#89472));
#19860=EDGE_LOOP('',(#89473,#89474,#89475,#89476));
#19861=EDGE_LOOP('',(#89477,#89478,#89479,#89480));
#19862=EDGE_LOOP('',(#89481,#89482,#89483,#89484));
#19863=EDGE_LOOP('',(#89485,#89486,#89487,#89488));
#19864=EDGE_LOOP('',(#89489,#89490,#89491,#89492));
#19865=EDGE_LOOP('',(#89493,#89494,#89495,#89496));
#19866=EDGE_LOOP('',(#89497,#89498,#89499,#89500));
#19867=EDGE_LOOP('',(#89501,#89502,#89503,#89504));
#19868=EDGE_LOOP('',(#89505,#89506,#89507,#89508));
#19869=EDGE_LOOP('',(#89509,#89510,#89511,#89512));
#19870=EDGE_LOOP('',(#89513,#89514,#89515,#89516));
#19871=EDGE_LOOP('',(#89517,#89518,#89519,#89520));
#19872=EDGE_LOOP('',(#89521,#89522,#89523,#89524));
#19873=EDGE_LOOP('',(#89525,#89526,#89527,#89528));
#19874=EDGE_LOOP('',(#89529,#89530,#89531,#89532));
#19875=EDGE_LOOP('',(#89533,#89534,#89535,#89536));
#19876=EDGE_LOOP('',(#89537,#89538,#89539,#89540));
#19877=EDGE_LOOP('',(#89541,#89542,#89543,#89544));
#19878=EDGE_LOOP('',(#89545,#89546,#89547,#89548));
#19879=EDGE_LOOP('',(#89549,#89550,#89551,#89552));
#19880=EDGE_LOOP('',(#89553,#89554,#89555,#89556));
#19881=EDGE_LOOP('',(#89557,#89558,#89559,#89560));
#19882=EDGE_LOOP('',(#89561,#89562,#89563,#89564));
#19883=EDGE_LOOP('',(#89565,#89566,#89567,#89568));
#19884=EDGE_LOOP('',(#89569,#89570,#89571,#89572));
#19885=EDGE_LOOP('',(#89573,#89574,#89575,#89576));
#19886=EDGE_LOOP('',(#89577,#89578,#89579,#89580));
#19887=EDGE_LOOP('',(#89581,#89582,#89583,#89584));
#19888=EDGE_LOOP('',(#89585,#89586,#89587,#89588));
#19889=EDGE_LOOP('',(#89589,#89590,#89591,#89592));
#19890=EDGE_LOOP('',(#89593,#89594,#89595,#89596));
#19891=EDGE_LOOP('',(#89597,#89598,#89599,#89600));
#19892=EDGE_LOOP('',(#89601,#89602,#89603,#89604));
#19893=EDGE_LOOP('',(#89605,#89606,#89607,#89608));
#19894=EDGE_LOOP('',(#89609,#89610,#89611,#89612));
#19895=EDGE_LOOP('',(#89613,#89614,#89615,#89616));
#19896=EDGE_LOOP('',(#89617,#89618,#89619,#89620));
#19897=EDGE_LOOP('',(#89621,#89622,#89623,#89624));
#19898=EDGE_LOOP('',(#89625,#89626,#89627,#89628));
#19899=EDGE_LOOP('',(#89629,#89630,#89631,#89632));
#19900=EDGE_LOOP('',(#89633,#89634,#89635,#89636));
#19901=EDGE_LOOP('',(#89637,#89638,#89639,#89640));
#19902=EDGE_LOOP('',(#89641,#89642,#89643,#89644));
#19903=EDGE_LOOP('',(#89645,#89646,#89647,#89648));
#19904=EDGE_LOOP('',(#89649,#89650,#89651,#89652));
#19905=EDGE_LOOP('',(#89653,#89654,#89655,#89656));
#19906=EDGE_LOOP('',(#89657,#89658,#89659,#89660));
#19907=EDGE_LOOP('',(#89661,#89662,#89663,#89664));
#19908=EDGE_LOOP('',(#89665,#89666,#89667,#89668));
#19909=EDGE_LOOP('',(#89669,#89670,#89671,#89672));
#19910=EDGE_LOOP('',(#89673,#89674,#89675,#89676));
#19911=EDGE_LOOP('',(#89677,#89678,#89679,#89680));
#19912=EDGE_LOOP('',(#89681,#89682,#89683,#89684));
#19913=EDGE_LOOP('',(#89685,#89686,#89687,#89688));
#19914=EDGE_LOOP('',(#89689,#89690,#89691,#89692));
#19915=EDGE_LOOP('',(#89693,#89694,#89695,#89696));
#19916=EDGE_LOOP('',(#89697,#89698,#89699,#89700));
#19917=EDGE_LOOP('',(#89701,#89702,#89703,#89704));
#19918=EDGE_LOOP('',(#89705,#89706,#89707,#89708));
#19919=EDGE_LOOP('',(#89709,#89710,#89711,#89712));
#19920=EDGE_LOOP('',(#89713,#89714,#89715,#89716));
#19921=EDGE_LOOP('',(#89717,#89718,#89719,#89720));
#19922=EDGE_LOOP('',(#89721,#89722,#89723,#89724));
#19923=EDGE_LOOP('',(#89725,#89726,#89727,#89728));
#19924=EDGE_LOOP('',(#89729,#89730,#89731,#89732));
#19925=EDGE_LOOP('',(#89733,#89734,#89735,#89736));
#19926=EDGE_LOOP('',(#89737,#89738,#89739,#89740));
#19927=EDGE_LOOP('',(#89741,#89742,#89743,#89744));
#19928=EDGE_LOOP('',(#89745,#89746,#89747,#89748));
#19929=EDGE_LOOP('',(#89749,#89750,#89751,#89752));
#19930=EDGE_LOOP('',(#89753,#89754,#89755,#89756));
#19931=EDGE_LOOP('',(#89757,#89758,#89759,#89760));
#19932=EDGE_LOOP('',(#89761,#89762,#89763,#89764));
#19933=EDGE_LOOP('',(#89765,#89766,#89767,#89768));
#19934=EDGE_LOOP('',(#89769,#89770,#89771,#89772));
#19935=EDGE_LOOP('',(#89773,#89774,#89775,#89776));
#19936=EDGE_LOOP('',(#89777,#89778,#89779,#89780));
#19937=EDGE_LOOP('',(#89781,#89782,#89783,#89784));
#19938=EDGE_LOOP('',(#89785,#89786,#89787,#89788));
#19939=EDGE_LOOP('',(#89789,#89790,#89791,#89792));
#19940=EDGE_LOOP('',(#89793,#89794,#89795,#89796,#89797,#89798,#89799,#89800));
#19941=EDGE_LOOP('',(#89801,#89802,#89803,#89804));
#19942=EDGE_LOOP('',(#89805,#89806,#89807,#89808));
#19943=EDGE_LOOP('',(#89809,#89810,#89811,#89812));
#19944=EDGE_LOOP('',(#89813,#89814,#89815,#89816));
#19945=EDGE_LOOP('',(#89817,#89818,#89819,#89820));
#19946=EDGE_LOOP('',(#89821,#89822,#89823,#89824));
#19947=EDGE_LOOP('',(#89825,#89826,#89827,#89828));
#19948=EDGE_LOOP('',(#89829,#89830,#89831,#89832));
#19949=EDGE_LOOP('',(#89833,#89834,#89835,#89836,#89837,#89838,#89839,#89840));
#19950=EDGE_LOOP('',(#89841,#89842,#89843,#89844,#89845,#89846,#89847,#89848,
#89849,#89850,#89851,#89852,#89853,#89854,#89855,#89856,#89857,#89858,#89859,
#89860,#89861,#89862,#89863,#89864,#89865,#89866,#89867,#89868,#89869,#89870,
#89871,#89872,#89873,#89874,#89875,#89876,#89877,#89878,#89879,#89880,#89881,
#89882,#89883,#89884,#89885,#89886,#89887,#89888,#89889,#89890,#89891,#89892,
#89893,#89894,#89895,#89896,#89897,#89898,#89899,#89900,#89901,#89902,#89903,
#89904,#89905,#89906,#89907,#89908,#89909,#89910,#89911,#89912,#89913,#89914,
#89915,#89916,#89917,#89918,#89919,#89920,#89921,#89922,#89923,#89924,#89925,
#89926,#89927,#89928,#89929,#89930,#89931,#89932,#89933,#89934,#89935,#89936,
#89937,#89938,#89939,#89940,#89941,#89942,#89943,#89944,#89945,#89946,#89947,
#89948,#89949,#89950,#89951,#89952,#89953,#89954,#89955,#89956,#89957,#89958,
#89959,#89960,#89961,#89962,#89963,#89964,#89965,#89966,#89967,#89968,#89969,
#89970,#89971,#89972,#89973,#89974,#89975,#89976,#89977,#89978,#89979,#89980,
#89981,#89982,#89983,#89984,#89985,#89986,#89987,#89988,#89989,#89990,#89991,
#89992,#89993,#89994,#89995,#89996,#89997,#89998,#89999,#90000,#90001,#90002,
#90003,#90004,#90005,#90006,#90007,#90008,#90009,#90010,#90011,#90012,#90013,
#90014,#90015,#90016,#90017,#90018,#90019,#90020,#90021,#90022,#90023,#90024,
#90025,#90026,#90027,#90028,#90029,#90030,#90031,#90032,#90033,#90034,#90035,
#90036,#90037,#90038,#90039,#90040,#90041,#90042,#90043,#90044,#90045,#90046,
#90047,#90048,#90049,#90050,#90051,#90052,#90053,#90054));
#19951=EDGE_LOOP('',(#90055,#90056,#90057,#90058));
#19952=EDGE_LOOP('',(#90059,#90060,#90061,#90062));
#19953=EDGE_LOOP('',(#90063,#90064,#90065,#90066));
#19954=EDGE_LOOP('',(#90067,#90068,#90069,#90070));
#19955=EDGE_LOOP('',(#90071,#90072,#90073,#90074));
#19956=EDGE_LOOP('',(#90075,#90076,#90077,#90078,#90079,#90080,#90081,#90082,
#90083,#90084,#90085,#90086,#90087,#90088,#90089,#90090,#90091,#90092,#90093,
#90094,#90095,#90096,#90097,#90098,#90099,#90100,#90101,#90102,#90103,#90104,
#90105,#90106,#90107,#90108,#90109,#90110,#90111,#90112,#90113,#90114,#90115,
#90116,#90117,#90118,#90119,#90120,#90121,#90122,#90123,#90124,#90125,#90126,
#90127,#90128,#90129,#90130,#90131,#90132,#90133,#90134,#90135,#90136,#90137,
#90138,#90139,#90140,#90141,#90142,#90143,#90144,#90145,#90146,#90147,#90148,
#90149,#90150,#90151,#90152,#90153,#90154,#90155,#90156,#90157,#90158,#90159,
#90160,#90161,#90162,#90163,#90164,#90165,#90166,#90167,#90168,#90169,#90170,
#90171,#90172,#90173,#90174,#90175,#90176,#90177,#90178,#90179,#90180,#90181,
#90182,#90183,#90184,#90185,#90186,#90187,#90188,#90189,#90190,#90191,#90192,
#90193,#90194,#90195,#90196,#90197,#90198,#90199,#90200,#90201,#90202,#90203,
#90204,#90205,#90206,#90207,#90208,#90209,#90210,#90211,#90212,#90213,#90214,
#90215,#90216,#90217,#90218,#90219,#90220,#90221,#90222,#90223,#90224,#90225,
#90226,#90227,#90228,#90229,#90230,#90231,#90232,#90233,#90234,#90235,#90236,
#90237,#90238,#90239,#90240,#90241,#90242,#90243,#90244,#90245,#90246,#90247,
#90248,#90249,#90250,#90251,#90252,#90253,#90254,#90255,#90256,#90257,#90258,
#90259,#90260,#90261,#90262,#90263,#90264,#90265,#90266,#90267,#90268,#90269,
#90270,#90271,#90272,#90273,#90274,#90275,#90276,#90277,#90278,#90279,#90280,
#90281,#90282,#90283,#90284,#90285,#90286,#90287,#90288));
#19957=EDGE_LOOP('',(#90289,#90290,#90291,#90292));
#24331=LINE('',#274156,#29558);
#24332=LINE('',#274159,#29559);
#24333=LINE('',#274165,#29560);
#24334=LINE('',#274169,#29561);
#24335=LINE('',#274173,#29562);
#24336=LINE('',#274177,#29563);
#24337=LINE('',#274181,#29564);
#24338=LINE('',#274185,#29565);
#24339=LINE('',#274188,#29566);
#24340=LINE('',#274189,#29567);
#24341=LINE('',#274192,#29568);
#24342=LINE('',#274193,#29569);
#24343=LINE('',#274196,#29570);
#24344=LINE('',#274197,#29571);
#24345=LINE('',#274200,#29572);
#24346=LINE('',#274204,#29573);
#24347=LINE('',#274205,#29574);
#24348=LINE('',#274208,#29575);
#24349=LINE('',#274212,#29576);
#24350=LINE('',#274213,#29577);
#24351=LINE('',#274216,#29578);
#24352=LINE('',#274220,#29579);
#24353=LINE('',#274221,#29580);
#24354=LINE('',#274224,#29581);
#24355=LINE('',#274228,#29582);
#24356=LINE('',#274229,#29583);
#24357=LINE('',#274232,#29584);
#24358=LINE('',#274236,#29585);
#24359=LINE('',#274237,#29586);
#24360=LINE('',#274240,#29587);
#24361=LINE('',#274244,#29588);
#24362=LINE('',#274245,#29589);
#24363=LINE('',#274254,#29590);
#24364=LINE('',#274258,#29591);
#24365=LINE('',#274262,#29592);
#24366=LINE('',#274265,#29593);
#24367=LINE('',#274268,#29594);
#24368=LINE('',#274270,#29595);
#24369=LINE('',#274271,#29596);
#24370=LINE('',#274274,#29597);
#24371=LINE('',#274278,#29598);
#24372=LINE('',#274279,#29599);
#24373=LINE('',#274282,#29600);
#24374=LINE('',#274286,#29601);
#24375=LINE('',#274287,#29602);
#24376=LINE('',#274290,#29603);
#24377=LINE('',#274294,#29604);
#24378=LINE('',#274295,#29605);
#24379=LINE('',#274304,#29606);
#24380=LINE('',#274308,#29607);
#24381=LINE('',#274312,#29608);
#24382=LINE('',#274316,#29609);
#24383=LINE('',#274318,#29610);
#24384=LINE('',#274320,#29611);
#24385=LINE('',#274324,#29612);
#24386=LINE('',#274328,#29613);
#24387=LINE('',#274332,#29614);
#24388=LINE('',#274336,#29615);
#24389=LINE('',#274340,#29616);
#24390=LINE('',#274344,#29617);
#24391=LINE('',#274346,#29618);
#24392=LINE('',#274348,#29619);
#24393=LINE('',#274352,#29620);
#24394=LINE('',#274356,#29621);
#24395=LINE('',#274360,#29622);
#24396=LINE('',#274364,#29623);
#24397=LINE('',#274368,#29624);
#24398=LINE('',#274372,#29625);
#24399=LINE('',#274374,#29626);
#24400=LINE('',#274376,#29627);
#24401=LINE('',#274380,#29628);
#24402=LINE('',#274384,#29629);
#24403=LINE('',#274388,#29630);
#24404=LINE('',#274392,#29631);
#24405=LINE('',#274396,#29632);
#24406=LINE('',#274400,#29633);
#24407=LINE('',#274402,#29634);
#24408=LINE('',#274404,#29635);
#24409=LINE('',#274408,#29636);
#24410=LINE('',#274411,#29637);
#24411=LINE('',#274417,#29638);
#24412=LINE('',#274421,#29639);
#24413=LINE('',#274425,#29640);
#24414=LINE('',#274429,#29641);
#24415=LINE('',#274431,#29642);
#24416=LINE('',#274433,#29643);
#24417=LINE('',#274437,#29644);
#24418=LINE('',#274441,#29645);
#24419=LINE('',#274445,#29646);
#24420=LINE('',#274449,#29647);
#24421=LINE('',#274453,#29648);
#24422=LINE('',#274457,#29649);
#24423=LINE('',#274459,#29650);
#24424=LINE('',#274461,#29651);
#24425=LINE('',#274465,#29652);
#24426=LINE('',#274469,#29653);
#24427=LINE('',#274473,#29654);
#24428=LINE('',#274477,#29655);
#24429=LINE('',#274481,#29656);
#24430=LINE('',#274485,#29657);
#24431=LINE('',#274487,#29658);
#24432=LINE('',#274489,#29659);
#24433=LINE('',#274493,#29660);
#24434=LINE('',#274497,#29661);
#24435=LINE('',#274501,#29662);
#24436=LINE('',#274505,#29663);
#24437=LINE('',#274509,#29664);
#24438=LINE('',#274513,#29665);
#24439=LINE('',#274515,#29666);
#24440=LINE('',#274517,#29667);
#24441=LINE('',#274521,#29668);
#24442=LINE('',#274524,#29669);
#24443=LINE('',#274526,#29670);
#24444=LINE('',#274527,#29671);
#24445=LINE('',#274529,#29672);
#24446=LINE('',#274531,#29673);
#24447=LINE('',#274533,#29674);
#24448=LINE('',#274535,#29675);
#24449=LINE('',#274537,#29676);
#24450=LINE('',#274539,#29677);
#24451=LINE('',#274541,#29678);
#24452=LINE('',#274543,#29679);
#24453=LINE('',#274545,#29680);
#24454=LINE('',#274547,#29681);
#24455=LINE('',#274549,#29682);
#24456=LINE('',#274551,#29683);
#24457=LINE('',#274553,#29684);
#24458=LINE('',#274555,#29685);
#24459=LINE('',#274557,#29686);
#24460=LINE('',#274559,#29687);
#24461=LINE('',#274561,#29688);
#24462=LINE('',#274563,#29689);
#24463=LINE('',#274565,#29690);
#24464=LINE('',#274567,#29691);
#24465=LINE('',#274569,#29692);
#24466=LINE('',#274571,#29693);
#24467=LINE('',#274573,#29694);
#24468=LINE('',#274575,#29695);
#24469=LINE('',#274577,#29696);
#24470=LINE('',#274579,#29697);
#24471=LINE('',#274581,#29698);
#24472=LINE('',#274583,#29699);
#24473=LINE('',#274585,#29700);
#24474=LINE('',#274587,#29701);
#24475=LINE('',#274589,#29702);
#24476=LINE('',#274591,#29703);
#24477=LINE('',#274593,#29704);
#24478=LINE('',#274595,#29705);
#24479=LINE('',#274597,#29706);
#24480=LINE('',#274599,#29707);
#24481=LINE('',#274601,#29708);
#24482=LINE('',#274603,#29709);
#24483=LINE('',#274605,#29710);
#24484=LINE('',#274607,#29711);
#24485=LINE('',#274609,#29712);
#24486=LINE('',#274611,#29713);
#24487=LINE('',#274613,#29714);
#24488=LINE('',#274615,#29715);
#24489=LINE('',#274617,#29716);
#24490=LINE('',#274619,#29717);
#24491=LINE('',#274621,#29718);
#24492=LINE('',#274623,#29719);
#24493=LINE('',#274625,#29720);
#24494=LINE('',#274627,#29721);
#24495=LINE('',#274629,#29722);
#24496=LINE('',#274631,#29723);
#24497=LINE('',#274633,#29724);
#24498=LINE('',#274635,#29725);
#24499=LINE('',#274642,#29726);
#24500=LINE('',#274645,#29727);
#24501=LINE('',#274651,#29728);
#24502=LINE('',#274655,#29729);
#24503=LINE('',#274658,#29730);
#24504=LINE('',#274660,#29731);
#24505=LINE('',#274664,#29732);
#24506=LINE('',#274668,#29733);
#24507=LINE('',#274672,#29734);
#24508=LINE('',#274675,#29735);
#24509=LINE('',#274678,#29736);
#24510=LINE('',#274680,#29737);
#24511=LINE('',#274681,#29738);
#24512=LINE('',#274684,#29739);
#24513=LINE('',#274688,#29740);
#24514=LINE('',#274689,#29741);
#24515=LINE('',#274692,#29742);
#24516=LINE('',#274696,#29743);
#24517=LINE('',#274697,#29744);
#24518=LINE('',#274700,#29745);
#24519=LINE('',#274704,#29746);
#24520=LINE('',#274705,#29747);
#24521=LINE('',#274708,#29748);
#24522=LINE('',#274711,#29749);
#24523=LINE('',#274714,#29750);
#24524=LINE('',#274715,#29751);
#24525=LINE('',#274718,#29752);
#24526=LINE('',#274722,#29753);
#24527=LINE('',#274723,#29754);
#24528=LINE('',#274726,#29755);
#24529=LINE('',#274730,#29756);
#24530=LINE('',#274731,#29757);
#24531=LINE('',#274740,#29758);
#24532=LINE('',#274744,#29759);
#24533=LINE('',#274748,#29760);
#24534=LINE('',#274751,#29761);
#24535=LINE('',#274754,#29762);
#24536=LINE('',#274756,#29763);
#24537=LINE('',#274757,#29764);
#24538=LINE('',#274760,#29765);
#24539=LINE('',#274764,#29766);
#24540=LINE('',#274765,#29767);
#24541=LINE('',#274768,#29768);
#24542=LINE('',#274772,#29769);
#24543=LINE('',#274773,#29770);
#24544=LINE('',#274776,#29771);
#24545=LINE('',#274780,#29772);
#24546=LINE('',#274781,#29773);
#24547=LINE('',#274790,#29774);
#24548=LINE('',#274793,#29775);
#24549=LINE('',#274798,#29776);
#24550=LINE('',#274800,#29777);
#24551=LINE('',#274804,#29778);
#24552=LINE('',#274808,#29779);
#24553=LINE('',#274812,#29780);
#24554=LINE('',#274816,#29781);
#24555=LINE('',#274820,#29782);
#24556=LINE('',#274823,#29783);
#24557=LINE('',#274826,#29784);
#24558=LINE('',#274828,#29785);
#24559=LINE('',#274829,#29786);
#24560=LINE('',#274832,#29787);
#24561=LINE('',#274836,#29788);
#24562=LINE('',#274837,#29789);
#24563=LINE('',#274840,#29790);
#24564=LINE('',#274844,#29791);
#24565=LINE('',#274845,#29792);
#24566=LINE('',#274848,#29793);
#24567=LINE('',#274852,#29794);
#24568=LINE('',#274853,#29795);
#24569=LINE('',#274856,#29796);
#24570=LINE('',#274860,#29797);
#24571=LINE('',#274861,#29798);
#24572=LINE('',#274864,#29799);
#24573=LINE('',#274868,#29800);
#24574=LINE('',#274869,#29801);
#24575=LINE('',#274872,#29802);
#24576=LINE('',#274875,#29803);
#24577=LINE('',#274878,#29804);
#24578=LINE('',#274879,#29805);
#24579=LINE('',#274888,#29806);
#24580=LINE('',#274892,#29807);
#24581=LINE('',#274896,#29808);
#24582=LINE('',#274899,#29809);
#24583=LINE('',#274902,#29810);
#24584=LINE('',#274904,#29811);
#24585=LINE('',#274905,#29812);
#24586=LINE('',#274908,#29813);
#24587=LINE('',#274912,#29814);
#24588=LINE('',#274913,#29815);
#24589=LINE('',#274916,#29816);
#24590=LINE('',#274920,#29817);
#24591=LINE('',#274921,#29818);
#24592=LINE('',#274924,#29819);
#24593=LINE('',#274928,#29820);
#24594=LINE('',#274929,#29821);
#24595=LINE('',#274938,#29822);
#24596=LINE('',#274941,#29823);
#24597=LINE('',#274946,#29824);
#24598=LINE('',#274948,#29825);
#24599=LINE('',#274952,#29826);
#24600=LINE('',#274956,#29827);
#24601=LINE('',#274960,#29828);
#24602=LINE('',#274964,#29829);
#24603=LINE('',#274968,#29830);
#24604=LINE('',#274971,#29831);
#24605=LINE('',#274974,#29832);
#24606=LINE('',#274976,#29833);
#24607=LINE('',#274977,#29834);
#24608=LINE('',#274980,#29835);
#24609=LINE('',#274984,#29836);
#24610=LINE('',#274985,#29837);
#24611=LINE('',#274988,#29838);
#24612=LINE('',#274992,#29839);
#24613=LINE('',#274993,#29840);
#24614=LINE('',#274996,#29841);
#24615=LINE('',#275000,#29842);
#24616=LINE('',#275001,#29843);
#24617=LINE('',#275004,#29844);
#24618=LINE('',#275008,#29845);
#24619=LINE('',#275009,#29846);
#24620=LINE('',#275012,#29847);
#24621=LINE('',#275016,#29848);
#24622=LINE('',#275017,#29849);
#24623=LINE('',#275020,#29850);
#24624=LINE('',#275023,#29851);
#24625=LINE('',#275026,#29852);
#24626=LINE('',#275027,#29853);
#24627=LINE('',#275036,#29854);
#24628=LINE('',#275040,#29855);
#24629=LINE('',#275044,#29856);
#24630=LINE('',#275047,#29857);
#24631=LINE('',#275050,#29858);
#24632=LINE('',#275052,#29859);
#24633=LINE('',#275053,#29860);
#24634=LINE('',#275056,#29861);
#24635=LINE('',#275060,#29862);
#24636=LINE('',#275061,#29863);
#24637=LINE('',#275064,#29864);
#24638=LINE('',#275068,#29865);
#24639=LINE('',#275069,#29866);
#24640=LINE('',#275072,#29867);
#24641=LINE('',#275076,#29868);
#24642=LINE('',#275077,#29869);
#24643=LINE('',#275084,#29870);
#24644=LINE('',#275086,#29871);
#24645=LINE('',#275088,#29872);
#24646=LINE('',#275089,#29873);
#24647=LINE('',#275093,#29874);
#24648=LINE('',#275095,#29875);
#24649=LINE('',#275097,#29876);
#24650=LINE('',#275098,#29877);
#24651=LINE('',#275102,#29878);
#24652=LINE('',#275104,#29879);
#24653=LINE('',#275106,#29880);
#24654=LINE('',#275107,#29881);
#24655=LINE('',#275110,#29882);
#24656=LINE('',#275112,#29883);
#24657=LINE('',#275113,#29884);
#24658=LINE('',#275116,#29885);
#24659=LINE('',#275118,#29886);
#24660=LINE('',#275119,#29887);
#24661=LINE('',#275125,#29888);
#24662=LINE('',#275128,#29889);
#24663=LINE('',#275130,#29890);
#24664=LINE('',#275131,#29891);
#24665=LINE('',#275137,#29892);
#24666=LINE('',#275140,#29893);
#24667=LINE('',#275142,#29894);
#24668=LINE('',#275143,#29895);
#24669=LINE('',#275149,#29896);
#24670=LINE('',#275152,#29897);
#24671=LINE('',#275154,#29898);
#24672=LINE('',#275155,#29899);
#24673=LINE('',#275161,#29900);
#24674=LINE('',#275164,#29901);
#24675=LINE('',#275166,#29902);
#24676=LINE('',#275167,#29903);
#24677=LINE('',#275170,#29904);
#24678=LINE('',#275172,#29905);
#24679=LINE('',#275173,#29906);
#24680=LINE('',#275176,#29907);
#24681=LINE('',#275178,#29908);
#24682=LINE('',#275179,#29909);
#24683=LINE('',#275182,#29910);
#24684=LINE('',#275184,#29911);
#24685=LINE('',#275185,#29912);
#24686=LINE('',#275189,#29913);
#24687=LINE('',#275191,#29914);
#24688=LINE('',#275193,#29915);
#24689=LINE('',#275194,#29916);
#24690=LINE('',#275197,#29917);
#24691=LINE('',#275199,#29918);
#24692=LINE('',#275200,#29919);
#24693=LINE('',#275203,#29920);
#24694=LINE('',#275205,#29921);
#24695=LINE('',#275206,#29922);
#24696=LINE('',#275209,#29923);
#24697=LINE('',#275211,#29924);
#24698=LINE('',#275212,#29925);
#24699=LINE('',#275218,#29926);
#24700=LINE('',#275221,#29927);
#24701=LINE('',#275223,#29928);
#24702=LINE('',#275224,#29929);
#24703=LINE('',#275230,#29930);
#24704=LINE('',#275233,#29931);
#24705=LINE('',#275235,#29932);
#24706=LINE('',#275236,#29933);
#24707=LINE('',#275242,#29934);
#24708=LINE('',#275245,#29935);
#24709=LINE('',#275247,#29936);
#24710=LINE('',#275248,#29937);
#24711=LINE('',#275254,#29938);
#24712=LINE('',#275257,#29939);
#24713=LINE('',#275259,#29940);
#24714=LINE('',#275260,#29941);
#24715=LINE('',#275263,#29942);
#24716=LINE('',#275265,#29943);
#24717=LINE('',#275266,#29944);
#24718=LINE('',#275269,#29945);
#24719=LINE('',#275271,#29946);
#24720=LINE('',#275272,#29947);
#24721=LINE('',#275275,#29948);
#24722=LINE('',#275277,#29949);
#24723=LINE('',#275278,#29950);
#24724=LINE('',#275284,#29951);
#24725=LINE('',#275287,#29952);
#24726=LINE('',#275289,#29953);
#24727=LINE('',#275290,#29954);
#24728=LINE('',#275296,#29955);
#24729=LINE('',#275299,#29956);
#24730=LINE('',#275301,#29957);
#24731=LINE('',#275302,#29958);
#24732=LINE('',#275309,#29959);
#24733=LINE('',#275311,#29960);
#24734=LINE('',#275313,#29961);
#24735=LINE('',#275314,#29962);
#24736=LINE('',#275320,#29963);
#24737=LINE('',#275323,#29964);
#24738=LINE('',#275325,#29965);
#24739=LINE('',#275326,#29966);
#24740=LINE('',#275329,#29967);
#24741=LINE('',#275331,#29968);
#24742=LINE('',#275332,#29969);
#24743=LINE('',#275335,#29970);
#24744=LINE('',#275337,#29971);
#24745=LINE('',#275338,#29972);
#24746=LINE('',#275341,#29973);
#24747=LINE('',#275343,#29974);
#24748=LINE('',#275344,#29975);
#24749=LINE('',#275350,#29976);
#24750=LINE('',#275353,#29977);
#24751=LINE('',#275355,#29978);
#24752=LINE('',#275356,#29979);
#24753=LINE('',#275359,#29980);
#24754=LINE('',#275361,#29981);
#24755=LINE('',#275362,#29982);
#24756=LINE('',#275365,#29983);
#24757=LINE('',#275367,#29984);
#24758=LINE('',#275368,#29985);
#24759=LINE('',#275371,#29986);
#24760=LINE('',#275373,#29987);
#24761=LINE('',#275374,#29988);
#24762=LINE('',#275380,#29989);
#24763=LINE('',#275383,#29990);
#24764=LINE('',#275385,#29991);
#24765=LINE('',#275386,#29992);
#24766=LINE('',#275392,#29993);
#24767=LINE('',#275395,#29994);
#24768=LINE('',#275397,#29995);
#24769=LINE('',#275398,#29996);
#24770=LINE('',#275404,#29997);
#24771=LINE('',#275407,#29998);
#24772=LINE('',#275409,#29999);
#24773=LINE('',#275410,#30000);
#24774=LINE('',#275416,#30001);
#24775=LINE('',#275418,#30002);
#24776=LINE('',#275419,#30003);
#24777=LINE('',#275423,#30004);
#24778=LINE('',#275425,#30005);
#24779=LINE('',#275427,#30006);
#24780=LINE('',#275428,#30007);
#24781=LINE('',#275431,#30008);
#24782=LINE('',#275433,#30009);
#24783=LINE('',#275434,#30010);
#24784=LINE('',#275437,#30011);
#24785=LINE('',#275439,#30012);
#24786=LINE('',#275440,#30013);
#24787=LINE('',#275446,#30014);
#24788=LINE('',#275449,#30015);
#24789=LINE('',#275451,#30016);
#24790=LINE('',#275452,#30017);
#24791=LINE('',#275458,#30018);
#24792=LINE('',#275461,#30019);
#24793=LINE('',#275463,#30020);
#24794=LINE('',#275464,#30021);
#24795=LINE('',#275470,#30022);
#24796=LINE('',#275473,#30023);
#24797=LINE('',#275475,#30024);
#24798=LINE('',#275476,#30025);
#24799=LINE('',#275482,#30026);
#24800=LINE('',#275485,#30027);
#24801=LINE('',#275487,#30028);
#24802=LINE('',#275488,#30029);
#24803=LINE('',#275491,#30030);
#24804=LINE('',#275493,#30031);
#24805=LINE('',#275494,#30032);
#24806=LINE('',#275496,#30033);
#24807=LINE('',#275497,#30034);
#24808=LINE('',#275501,#30035);
#24809=LINE('',#275503,#30036);
#24810=LINE('',#275505,#30037);
#24811=LINE('',#275506,#30038);
#24812=LINE('',#275509,#30039);
#24813=LINE('',#275511,#30040);
#24814=LINE('',#275512,#30041);
#24815=LINE('',#275515,#30042);
#24816=LINE('',#275517,#30043);
#24817=LINE('',#275518,#30044);
#24818=LINE('',#275521,#30045);
#24819=LINE('',#275523,#30046);
#24820=LINE('',#275524,#30047);
#24821=LINE('',#275530,#30048);
#24822=LINE('',#275533,#30049);
#24823=LINE('',#275535,#30050);
#24824=LINE('',#275536,#30051);
#24825=LINE('',#275542,#30052);
#24826=LINE('',#275545,#30053);
#24827=LINE('',#275547,#30054);
#24828=LINE('',#275548,#30055);
#24829=LINE('',#275554,#30056);
#24830=LINE('',#275557,#30057);
#24831=LINE('',#275559,#30058);
#24832=LINE('',#275560,#30059);
#24833=LINE('',#275566,#30060);
#24834=LINE('',#275569,#30061);
#24835=LINE('',#275571,#30062);
#24836=LINE('',#275572,#30063);
#24837=LINE('',#275575,#30064);
#24838=LINE('',#275577,#30065);
#24839=LINE('',#275578,#30066);
#24840=LINE('',#275581,#30067);
#24841=LINE('',#275583,#30068);
#24842=LINE('',#275584,#30069);
#24843=LINE('',#275587,#30070);
#24844=LINE('',#275589,#30071);
#24845=LINE('',#275590,#30072);
#24846=LINE('',#275596,#30073);
#24847=LINE('',#275599,#30074);
#24848=LINE('',#275601,#30075);
#24849=LINE('',#275602,#30076);
#24850=LINE('',#275608,#30077);
#24851=LINE('',#275611,#30078);
#24852=LINE('',#275613,#30079);
#24853=LINE('',#275614,#30080);
#24854=LINE('',#275620,#30081);
#24855=LINE('',#275623,#30082);
#24856=LINE('',#275625,#30083);
#24857=LINE('',#275626,#30084);
#24858=LINE('',#275632,#30085);
#24859=LINE('',#275635,#30086);
#24860=LINE('',#275637,#30087);
#24861=LINE('',#275638,#30088);
#24862=LINE('',#275641,#30089);
#24863=LINE('',#275643,#30090);
#24864=LINE('',#275644,#30091);
#24865=LINE('',#275647,#30092);
#24866=LINE('',#275649,#30093);
#24867=LINE('',#275650,#30094);
#24868=LINE('',#275653,#30095);
#24869=LINE('',#275655,#30096);
#24870=LINE('',#275656,#30097);
#24871=LINE('',#275662,#30098);
#24872=LINE('',#275665,#30099);
#24873=LINE('',#275667,#30100);
#24874=LINE('',#275668,#30101);
#24875=LINE('',#275671,#30102);
#24876=LINE('',#275673,#30103);
#24877=LINE('',#275674,#30104);
#24878=LINE('',#275677,#30105);
#24879=LINE('',#275679,#30106);
#24880=LINE('',#275680,#30107);
#24881=LINE('',#275683,#30108);
#24882=LINE('',#275685,#30109);
#24883=LINE('',#275686,#30110);
#24884=LINE('',#275692,#30111);
#24885=LINE('',#275695,#30112);
#24886=LINE('',#275697,#30113);
#24887=LINE('',#275698,#30114);
#24888=LINE('',#275704,#30115);
#24889=LINE('',#275707,#30116);
#24890=LINE('',#275709,#30117);
#24891=LINE('',#275710,#30118);
#24892=LINE('',#275716,#30119);
#24893=LINE('',#275719,#30120);
#24894=LINE('',#275721,#30121);
#24895=LINE('',#275722,#30122);
#24896=LINE('',#275728,#30123);
#24897=LINE('',#275730,#30124);
#24898=LINE('',#275731,#30125);
#24899=LINE('',#275735,#30126);
#24900=LINE('',#275737,#30127);
#24901=LINE('',#275739,#30128);
#24902=LINE('',#275740,#30129);
#24903=LINE('',#275743,#30130);
#24904=LINE('',#275745,#30131);
#24905=LINE('',#275746,#30132);
#24906=LINE('',#275749,#30133);
#24907=LINE('',#275751,#30134);
#24908=LINE('',#275752,#30135);
#24909=LINE('',#275758,#30136);
#24910=LINE('',#275761,#30137);
#24911=LINE('',#275763,#30138);
#24912=LINE('',#275764,#30139);
#24913=LINE('',#275770,#30140);
#24914=LINE('',#275773,#30141);
#24915=LINE('',#275775,#30142);
#24916=LINE('',#275776,#30143);
#24917=LINE('',#275782,#30144);
#24918=LINE('',#275785,#30145);
#24919=LINE('',#275787,#30146);
#24920=LINE('',#275788,#30147);
#24921=LINE('',#275794,#30148);
#24922=LINE('',#275797,#30149);
#24923=LINE('',#275799,#30150);
#24924=LINE('',#275800,#30151);
#24925=LINE('',#275803,#30152);
#24926=LINE('',#275805,#30153);
#24927=LINE('',#275806,#30154);
#24928=LINE('',#275808,#30155);
#24929=LINE('',#275809,#30156);
#24930=LINE('',#275813,#30157);
#24931=LINE('',#275815,#30158);
#24932=LINE('',#275817,#30159);
#24933=LINE('',#275818,#30160);
#24934=LINE('',#275821,#30161);
#24935=LINE('',#275823,#30162);
#24936=LINE('',#275824,#30163);
#24937=LINE('',#275827,#30164);
#24938=LINE('',#275829,#30165);
#24939=LINE('',#275830,#30166);
#24940=LINE('',#275833,#30167);
#24941=LINE('',#275835,#30168);
#24942=LINE('',#275836,#30169);
#24943=LINE('',#275842,#30170);
#24944=LINE('',#275845,#30171);
#24945=LINE('',#275847,#30172);
#24946=LINE('',#275848,#30173);
#24947=LINE('',#275854,#30174);
#24948=LINE('',#275857,#30175);
#24949=LINE('',#275859,#30176);
#24950=LINE('',#275860,#30177);
#24951=LINE('',#275866,#30178);
#24952=LINE('',#275869,#30179);
#24953=LINE('',#275871,#30180);
#24954=LINE('',#275872,#30181);
#24955=LINE('',#275878,#30182);
#24956=LINE('',#275881,#30183);
#24957=LINE('',#275883,#30184);
#24958=LINE('',#275884,#30185);
#24959=LINE('',#275887,#30186);
#24960=LINE('',#275889,#30187);
#24961=LINE('',#275890,#30188);
#24962=LINE('',#275893,#30189);
#24963=LINE('',#275895,#30190);
#24964=LINE('',#275896,#30191);
#24965=LINE('',#275899,#30192);
#24966=LINE('',#275901,#30193);
#24967=LINE('',#275902,#30194);
#24968=LINE('',#275908,#30195);
#24969=LINE('',#275911,#30196);
#24970=LINE('',#275913,#30197);
#24971=LINE('',#275914,#30198);
#24972=LINE('',#275920,#30199);
#24973=LINE('',#275923,#30200);
#24974=LINE('',#275925,#30201);
#24975=LINE('',#275926,#30202);
#24976=LINE('',#275932,#30203);
#24977=LINE('',#275935,#30204);
#24978=LINE('',#275937,#30205);
#24979=LINE('',#275938,#30206);
#24980=LINE('',#275944,#30207);
#24981=LINE('',#275947,#30208);
#24982=LINE('',#275949,#30209);
#24983=LINE('',#275950,#30210);
#24984=LINE('',#275953,#30211);
#24985=LINE('',#275955,#30212);
#24986=LINE('',#275956,#30213);
#24987=LINE('',#275959,#30214);
#24988=LINE('',#275961,#30215);
#24989=LINE('',#275962,#30216);
#24990=LINE('',#275965,#30217);
#24991=LINE('',#275967,#30218);
#24992=LINE('',#275968,#30219);
#24993=LINE('',#275974,#30220);
#24994=LINE('',#275977,#30221);
#24995=LINE('',#275979,#30222);
#24996=LINE('',#275980,#30223);
#24997=LINE('',#275983,#30224);
#24998=LINE('',#275985,#30225);
#24999=LINE('',#275986,#30226);
#25000=LINE('',#275989,#30227);
#25001=LINE('',#275991,#30228);
#25002=LINE('',#275992,#30229);
#25003=LINE('',#275995,#30230);
#25004=LINE('',#275997,#30231);
#25005=LINE('',#275998,#30232);
#25006=LINE('',#276004,#30233);
#25007=LINE('',#276007,#30234);
#25008=LINE('',#276009,#30235);
#25009=LINE('',#276010,#30236);
#25010=LINE('',#276016,#30237);
#25011=LINE('',#276019,#30238);
#25012=LINE('',#276021,#30239);
#25013=LINE('',#276022,#30240);
#25014=LINE('',#276028,#30241);
#25015=LINE('',#276031,#30242);
#25016=LINE('',#276033,#30243);
#25017=LINE('',#276034,#30244);
#25018=LINE('',#276040,#30245);
#25019=LINE('',#276042,#30246);
#25020=LINE('',#276043,#30247);
#25021=LINE('',#276047,#30248);
#25022=LINE('',#276049,#30249);
#25023=LINE('',#276051,#30250);
#25024=LINE('',#276052,#30251);
#25025=LINE('',#276055,#30252);
#25026=LINE('',#276057,#30253);
#25027=LINE('',#276058,#30254);
#25028=LINE('',#276061,#30255);
#25029=LINE('',#276063,#30256);
#25030=LINE('',#276064,#30257);
#25031=LINE('',#276070,#30258);
#25032=LINE('',#276073,#30259);
#25033=LINE('',#276075,#30260);
#25034=LINE('',#276076,#30261);
#25035=LINE('',#276082,#30262);
#25036=LINE('',#276085,#30263);
#25037=LINE('',#276087,#30264);
#25038=LINE('',#276088,#30265);
#25039=LINE('',#276094,#30266);
#25040=LINE('',#276097,#30267);
#25041=LINE('',#276099,#30268);
#25042=LINE('',#276100,#30269);
#25043=LINE('',#276106,#30270);
#25044=LINE('',#276109,#30271);
#25045=LINE('',#276111,#30272);
#25046=LINE('',#276112,#30273);
#25047=LINE('',#276115,#30274);
#25048=LINE('',#276117,#30275);
#25049=LINE('',#276118,#30276);
#25050=LINE('',#276120,#30277);
#25051=LINE('',#276121,#30278);
#25052=LINE('',#276124,#30279);
#25053=LINE('',#276126,#30280);
#25054=LINE('',#276127,#30281);
#25055=LINE('',#276130,#30282);
#25056=LINE('',#276132,#30283);
#25057=LINE('',#276133,#30284);
#25058=LINE('',#276136,#30285);
#25059=LINE('',#276138,#30286);
#25060=LINE('',#276139,#30287);
#25061=LINE('',#276145,#30288);
#25062=LINE('',#276148,#30289);
#25063=LINE('',#276150,#30290);
#25064=LINE('',#276151,#30291);
#25065=LINE('',#276157,#30292);
#25066=LINE('',#276160,#30293);
#25067=LINE('',#276162,#30294);
#25068=LINE('',#276163,#30295);
#25069=LINE('',#276169,#30296);
#25070=LINE('',#276172,#30297);
#25071=LINE('',#276174,#30298);
#25072=LINE('',#276175,#30299);
#25073=LINE('',#276181,#30300);
#25074=LINE('',#276184,#30301);
#25075=LINE('',#276186,#30302);
#25076=LINE('',#276187,#30303);
#25077=LINE('',#276190,#30304);
#25078=LINE('',#276192,#30305);
#25079=LINE('',#276193,#30306);
#25080=LINE('',#276196,#30307);
#25081=LINE('',#276198,#30308);
#25082=LINE('',#276199,#30309);
#25083=LINE('',#276202,#30310);
#25084=LINE('',#276204,#30311);
#25085=LINE('',#276205,#30312);
#25086=LINE('',#276211,#30313);
#25087=LINE('',#276214,#30314);
#25088=LINE('',#276216,#30315);
#25089=LINE('',#276217,#30316);
#25090=LINE('',#276223,#30317);
#25091=LINE('',#276226,#30318);
#25092=LINE('',#276228,#30319);
#25093=LINE('',#276229,#30320);
#25094=LINE('',#276235,#30321);
#25095=LINE('',#276238,#30322);
#25096=LINE('',#276240,#30323);
#25097=LINE('',#276241,#30324);
#25098=LINE('',#276247,#30325);
#25099=LINE('',#276250,#30326);
#25100=LINE('',#276252,#30327);
#25101=LINE('',#276253,#30328);
#25102=LINE('',#276256,#30329);
#25103=LINE('',#276258,#30330);
#25104=LINE('',#276259,#30331);
#25105=LINE('',#276262,#30332);
#25106=LINE('',#276264,#30333);
#25107=LINE('',#276265,#30334);
#25108=LINE('',#276268,#30335);
#25109=LINE('',#276270,#30336);
#25110=LINE('',#276271,#30337);
#25111=LINE('',#276277,#30338);
#25112=LINE('',#276280,#30339);
#25113=LINE('',#276282,#30340);
#25114=LINE('',#276283,#30341);
#25115=LINE('',#276286,#30342);
#25116=LINE('',#276288,#30343);
#25117=LINE('',#276289,#30344);
#25118=LINE('',#276292,#30345);
#25119=LINE('',#276294,#30346);
#25120=LINE('',#276295,#30347);
#25121=LINE('',#276298,#30348);
#25122=LINE('',#276300,#30349);
#25123=LINE('',#276301,#30350);
#25124=LINE('',#276307,#30351);
#25125=LINE('',#276310,#30352);
#25126=LINE('',#276312,#30353);
#25127=LINE('',#276313,#30354);
#25128=LINE('',#276319,#30355);
#25129=LINE('',#276322,#30356);
#25130=LINE('',#276324,#30357);
#25131=LINE('',#276325,#30358);
#25132=LINE('',#276331,#30359);
#25133=LINE('',#276334,#30360);
#25134=LINE('',#276336,#30361);
#25135=LINE('',#276337,#30362);
#25136=LINE('',#276343,#30363);
#25137=LINE('',#276345,#30364);
#25138=LINE('',#276346,#30365);
#25139=LINE('',#276349,#30366);
#25140=LINE('',#276351,#30367);
#25141=LINE('',#276352,#30368);
#25142=LINE('',#276354,#30369);
#25143=LINE('',#276355,#30370);
#25144=LINE('',#276358,#30371);
#25145=LINE('',#276360,#30372);
#25146=LINE('',#276361,#30373);
#25147=LINE('',#276363,#30374);
#25148=LINE('',#276364,#30375);
#25149=LINE('',#276368,#30376);
#25150=LINE('',#276370,#30377);
#25151=LINE('',#276372,#30378);
#25152=LINE('',#276374,#30379);
#25153=LINE('',#276376,#30380);
#25154=LINE('',#276378,#30381);
#25155=LINE('',#276380,#30382);
#25156=LINE('',#276381,#30383);
#25157=LINE('',#276385,#30384);
#25158=LINE('',#276386,#30385);
#25159=LINE('',#276387,#30386);
#25160=LINE('',#276390,#30387);
#25161=LINE('',#276391,#30388);
#25162=LINE('',#276394,#30389);
#25163=LINE('',#276395,#30390);
#25164=LINE('',#276398,#30391);
#25165=LINE('',#276399,#30392);
#25166=LINE('',#276402,#30393);
#25167=LINE('',#276403,#30394);
#25168=LINE('',#276406,#30395);
#25169=LINE('',#276407,#30396);
#25170=LINE('',#276410,#30397);
#25171=LINE('',#276411,#30398);
#25172=LINE('',#276413,#30399);
#25173=LINE('',#276418,#30400);
#25174=LINE('',#276420,#30401);
#25175=LINE('',#276422,#30402);
#25176=LINE('',#276423,#30403);
#25177=LINE('',#276426,#30404);
#25178=LINE('',#276428,#30405);
#25179=LINE('',#276429,#30406);
#25180=LINE('',#276432,#30407);
#25181=LINE('',#276434,#30408);
#25182=LINE('',#276435,#30409);
#25183=LINE('',#276437,#30410);
#25184=LINE('',#276438,#30411);
#29558=VECTOR('',#140420,1000.);
#29559=VECTOR('',#140423,1000.);
#29560=VECTOR('',#140428,1000.);
#29561=VECTOR('',#140431,1000.);
#29562=VECTOR('',#140434,1000.);
#29563=VECTOR('',#140437,1000.);
#29564=VECTOR('',#140440,1000.);
#29565=VECTOR('',#140443,1000.);
#29566=VECTOR('',#140446,1000.);
#29567=VECTOR('',#140447,1000.);
#29568=VECTOR('',#140450,1000.);
#29569=VECTOR('',#140451,1000.);
#29570=VECTOR('',#140454,1000.);
#29571=VECTOR('',#140455,1000.);
#29572=VECTOR('',#140458,1000.);
#29573=VECTOR('',#140463,1000.);
#29574=VECTOR('',#140464,1000.);
#29575=VECTOR('',#140467,1000.);
#29576=VECTOR('',#140472,1000.);
#29577=VECTOR('',#140473,1000.);
#29578=VECTOR('',#140476,1000.);
#29579=VECTOR('',#140481,1000.);
#29580=VECTOR('',#140482,1000.);
#29581=VECTOR('',#140485,1000.);
#29582=VECTOR('',#140490,1000.);
#29583=VECTOR('',#140491,1000.);
#29584=VECTOR('',#140494,1000.);
#29585=VECTOR('',#140499,1000.);
#29586=VECTOR('',#140500,1000.);
#29587=VECTOR('',#140503,1000.);
#29588=VECTOR('',#140508,1000.);
#29589=VECTOR('',#140509,1000.);
#29590=VECTOR('',#140520,1000.);
#29591=VECTOR('',#140523,1000.);
#29592=VECTOR('',#140526,1000.);
#29593=VECTOR('',#140529,1000.);
#29594=VECTOR('',#140532,1000.);
#29595=VECTOR('',#140533,1000.);
#29596=VECTOR('',#140534,1000.);
#29597=VECTOR('',#140537,1000.);
#29598=VECTOR('',#140542,1000.);
#29599=VECTOR('',#140543,1000.);
#29600=VECTOR('',#140546,1000.);
#29601=VECTOR('',#140551,1000.);
#29602=VECTOR('',#140552,1000.);
#29603=VECTOR('',#140555,1000.);
#29604=VECTOR('',#140560,1000.);
#29605=VECTOR('',#140561,1000.);
#29606=VECTOR('',#140572,1000.);
#29607=VECTOR('',#140575,1000.);
#29608=VECTOR('',#140578,1000.);
#29609=VECTOR('',#140581,1000.);
#29610=VECTOR('',#140582,1000.);
#29611=VECTOR('',#140583,1000.);
#29612=VECTOR('',#140586,1000.);
#29613=VECTOR('',#140589,1000.);
#29614=VECTOR('',#140592,1000.);
#29615=VECTOR('',#140595,1000.);
#29616=VECTOR('',#140598,1000.);
#29617=VECTOR('',#140601,1000.);
#29618=VECTOR('',#140602,1000.);
#29619=VECTOR('',#140603,1000.);
#29620=VECTOR('',#140606,1000.);
#29621=VECTOR('',#140609,1000.);
#29622=VECTOR('',#140612,1000.);
#29623=VECTOR('',#140615,1000.);
#29624=VECTOR('',#140618,1000.);
#29625=VECTOR('',#140621,1000.);
#29626=VECTOR('',#140622,1000.);
#29627=VECTOR('',#140623,1000.);
#29628=VECTOR('',#140626,1000.);
#29629=VECTOR('',#140629,1000.);
#29630=VECTOR('',#140632,1000.);
#29631=VECTOR('',#140635,1000.);
#29632=VECTOR('',#140638,1000.);
#29633=VECTOR('',#140641,1000.);
#29634=VECTOR('',#140642,1000.);
#29635=VECTOR('',#140643,1000.);
#29636=VECTOR('',#140646,1000.);
#29637=VECTOR('',#140649,1000.);
#29638=VECTOR('',#140654,1000.);
#29639=VECTOR('',#140657,1000.);
#29640=VECTOR('',#140660,1000.);
#29641=VECTOR('',#140663,1000.);
#29642=VECTOR('',#140664,1000.);
#29643=VECTOR('',#140665,1000.);
#29644=VECTOR('',#140668,1000.);
#29645=VECTOR('',#140671,1000.);
#29646=VECTOR('',#140674,1000.);
#29647=VECTOR('',#140677,1000.);
#29648=VECTOR('',#140680,1000.);
#29649=VECTOR('',#140683,1000.);
#29650=VECTOR('',#140684,1000.);
#29651=VECTOR('',#140685,1000.);
#29652=VECTOR('',#140688,1000.);
#29653=VECTOR('',#140691,1000.);
#29654=VECTOR('',#140694,1000.);
#29655=VECTOR('',#140697,1000.);
#29656=VECTOR('',#140700,1000.);
#29657=VECTOR('',#140703,1000.);
#29658=VECTOR('',#140704,1000.);
#29659=VECTOR('',#140705,1000.);
#29660=VECTOR('',#140708,1000.);
#29661=VECTOR('',#140711,1000.);
#29662=VECTOR('',#140714,1000.);
#29663=VECTOR('',#140717,1000.);
#29664=VECTOR('',#140720,1000.);
#29665=VECTOR('',#140723,1000.);
#29666=VECTOR('',#140724,1000.);
#29667=VECTOR('',#140725,1000.);
#29668=VECTOR('',#140728,1000.);
#29669=VECTOR('',#140731,1000.);
#29670=VECTOR('',#140734,1000.);
#29671=VECTOR('',#140735,1000.);
#29672=VECTOR('',#140738,1000.);
#29673=VECTOR('',#140741,1000.);
#29674=VECTOR('',#140744,1000.);
#29675=VECTOR('',#140747,1000.);
#29676=VECTOR('',#140750,1000.);
#29677=VECTOR('',#140753,1000.);
#29678=VECTOR('',#140756,1000.);
#29679=VECTOR('',#140759,1000.);
#29680=VECTOR('',#140762,1000.);
#29681=VECTOR('',#140765,1000.);
#29682=VECTOR('',#140768,1000.);
#29683=VECTOR('',#140771,1000.);
#29684=VECTOR('',#140774,1000.);
#29685=VECTOR('',#140777,1000.);
#29686=VECTOR('',#140780,1000.);
#29687=VECTOR('',#140783,1000.);
#29688=VECTOR('',#140786,1000.);
#29689=VECTOR('',#140789,1000.);
#29690=VECTOR('',#140792,1000.);
#29691=VECTOR('',#140795,1000.);
#29692=VECTOR('',#140798,1000.);
#29693=VECTOR('',#140801,1000.);
#29694=VECTOR('',#140804,1000.);
#29695=VECTOR('',#140807,1000.);
#29696=VECTOR('',#140810,1000.);
#29697=VECTOR('',#140813,1000.);
#29698=VECTOR('',#140816,1000.);
#29699=VECTOR('',#140819,1000.);
#29700=VECTOR('',#140822,1000.);
#29701=VECTOR('',#140825,1000.);
#29702=VECTOR('',#140828,1000.);
#29703=VECTOR('',#140831,1000.);
#29704=VECTOR('',#140834,1000.);
#29705=VECTOR('',#140837,1000.);
#29706=VECTOR('',#140840,1000.);
#29707=VECTOR('',#140843,1000.);
#29708=VECTOR('',#140846,1000.);
#29709=VECTOR('',#140849,1000.);
#29710=VECTOR('',#140852,1000.);
#29711=VECTOR('',#140855,1000.);
#29712=VECTOR('',#140858,1000.);
#29713=VECTOR('',#140861,1000.);
#29714=VECTOR('',#140864,1000.);
#29715=VECTOR('',#140867,1000.);
#29716=VECTOR('',#140870,1000.);
#29717=VECTOR('',#140873,1000.);
#29718=VECTOR('',#140876,1000.);
#29719=VECTOR('',#140879,1000.);
#29720=VECTOR('',#140882,1000.);
#29721=VECTOR('',#140885,1000.);
#29722=VECTOR('',#140888,1000.);
#29723=VECTOR('',#140891,1000.);
#29724=VECTOR('',#140894,1000.);
#29725=VECTOR('',#140897,1000.);
#29726=VECTOR('',#140904,1000.);
#29727=VECTOR('',#140907,1000.);
#29728=VECTOR('',#140912,1000.);
#29729=VECTOR('',#140915,1000.);
#29730=VECTOR('',#140918,1000.);
#29731=VECTOR('',#140919,1000.);
#29732=VECTOR('',#140922,1000.);
#29733=VECTOR('',#140925,1000.);
#29734=VECTOR('',#140928,1000.);
#29735=VECTOR('',#140931,1000.);
#29736=VECTOR('',#140934,1000.);
#29737=VECTOR('',#140935,1000.);
#29738=VECTOR('',#140936,1000.);
#29739=VECTOR('',#140939,1000.);
#29740=VECTOR('',#140944,1000.);
#29741=VECTOR('',#140945,1000.);
#29742=VECTOR('',#140948,1000.);
#29743=VECTOR('',#140953,1000.);
#29744=VECTOR('',#140954,1000.);
#29745=VECTOR('',#140957,1000.);
#29746=VECTOR('',#140962,1000.);
#29747=VECTOR('',#140963,1000.);
#29748=VECTOR('',#140966,1000.);
#29749=VECTOR('',#140971,1000.);
#29750=VECTOR('',#140974,1000.);
#29751=VECTOR('',#140975,1000.);
#29752=VECTOR('',#140978,1000.);
#29753=VECTOR('',#140983,1000.);
#29754=VECTOR('',#140984,1000.);
#29755=VECTOR('',#140987,1000.);
#29756=VECTOR('',#140992,1000.);
#29757=VECTOR('',#140993,1000.);
#29758=VECTOR('',#141004,1000.);
#29759=VECTOR('',#141007,1000.);
#29760=VECTOR('',#141010,1000.);
#29761=VECTOR('',#141013,1000.);
#29762=VECTOR('',#141016,1000.);
#29763=VECTOR('',#141017,1000.);
#29764=VECTOR('',#141018,1000.);
#29765=VECTOR('',#141021,1000.);
#29766=VECTOR('',#141026,1000.);
#29767=VECTOR('',#141027,1000.);
#29768=VECTOR('',#141030,1000.);
#29769=VECTOR('',#141035,1000.);
#29770=VECTOR('',#141036,1000.);
#29771=VECTOR('',#141039,1000.);
#29772=VECTOR('',#141044,1000.);
#29773=VECTOR('',#141045,1000.);
#29774=VECTOR('',#141056,1000.);
#29775=VECTOR('',#141059,1000.);
#29776=VECTOR('',#141064,1000.);
#29777=VECTOR('',#141065,1000.);
#29778=VECTOR('',#141068,1000.);
#29779=VECTOR('',#141071,1000.);
#29780=VECTOR('',#141074,1000.);
#29781=VECTOR('',#141077,1000.);
#29782=VECTOR('',#141080,1000.);
#29783=VECTOR('',#141083,1000.);
#29784=VECTOR('',#141086,1000.);
#29785=VECTOR('',#141087,1000.);
#29786=VECTOR('',#141088,1000.);
#29787=VECTOR('',#141091,1000.);
#29788=VECTOR('',#141096,1000.);
#29789=VECTOR('',#141097,1000.);
#29790=VECTOR('',#141100,1000.);
#29791=VECTOR('',#141105,1000.);
#29792=VECTOR('',#141106,1000.);
#29793=VECTOR('',#141109,1000.);
#29794=VECTOR('',#141114,1000.);
#29795=VECTOR('',#141115,1000.);
#29796=VECTOR('',#141118,1000.);
#29797=VECTOR('',#141123,1000.);
#29798=VECTOR('',#141124,1000.);
#29799=VECTOR('',#141127,1000.);
#29800=VECTOR('',#141132,1000.);
#29801=VECTOR('',#141133,1000.);
#29802=VECTOR('',#141136,1000.);
#29803=VECTOR('',#141141,1000.);
#29804=VECTOR('',#141144,1000.);
#29805=VECTOR('',#141145,1000.);
#29806=VECTOR('',#141156,1000.);
#29807=VECTOR('',#141159,1000.);
#29808=VECTOR('',#141162,1000.);
#29809=VECTOR('',#141165,1000.);
#29810=VECTOR('',#141168,1000.);
#29811=VECTOR('',#141169,1000.);
#29812=VECTOR('',#141170,1000.);
#29813=VECTOR('',#141173,1000.);
#29814=VECTOR('',#141178,1000.);
#29815=VECTOR('',#141179,1000.);
#29816=VECTOR('',#141182,1000.);
#29817=VECTOR('',#141187,1000.);
#29818=VECTOR('',#141188,1000.);
#29819=VECTOR('',#141191,1000.);
#29820=VECTOR('',#141196,1000.);
#29821=VECTOR('',#141197,1000.);
#29822=VECTOR('',#141208,1000.);
#29823=VECTOR('',#141211,1000.);
#29824=VECTOR('',#141216,1000.);
#29825=VECTOR('',#141217,1000.);
#29826=VECTOR('',#141220,1000.);
#29827=VECTOR('',#141223,1000.);
#29828=VECTOR('',#141226,1000.);
#29829=VECTOR('',#141229,1000.);
#29830=VECTOR('',#141232,1000.);
#29831=VECTOR('',#141235,1000.);
#29832=VECTOR('',#141238,1000.);
#29833=VECTOR('',#141239,1000.);
#29834=VECTOR('',#141240,1000.);
#29835=VECTOR('',#141243,1000.);
#29836=VECTOR('',#141248,1000.);
#29837=VECTOR('',#141249,1000.);
#29838=VECTOR('',#141252,1000.);
#29839=VECTOR('',#141257,1000.);
#29840=VECTOR('',#141258,1000.);
#29841=VECTOR('',#141261,1000.);
#29842=VECTOR('',#141266,1000.);
#29843=VECTOR('',#141267,1000.);
#29844=VECTOR('',#141270,1000.);
#29845=VECTOR('',#141275,1000.);
#29846=VECTOR('',#141276,1000.);
#29847=VECTOR('',#141279,1000.);
#29848=VECTOR('',#141284,1000.);
#29849=VECTOR('',#141285,1000.);
#29850=VECTOR('',#141288,1000.);
#29851=VECTOR('',#141293,1000.);
#29852=VECTOR('',#141296,1000.);
#29853=VECTOR('',#141297,1000.);
#29854=VECTOR('',#141308,1000.);
#29855=VECTOR('',#141311,1000.);
#29856=VECTOR('',#141314,1000.);
#29857=VECTOR('',#141317,1000.);
#29858=VECTOR('',#141320,1000.);
#29859=VECTOR('',#141321,1000.);
#29860=VECTOR('',#141322,1000.);
#29861=VECTOR('',#141325,1000.);
#29862=VECTOR('',#141330,1000.);
#29863=VECTOR('',#141331,1000.);
#29864=VECTOR('',#141334,1000.);
#29865=VECTOR('',#141339,1000.);
#29866=VECTOR('',#141340,1000.);
#29867=VECTOR('',#141343,1000.);
#29868=VECTOR('',#141348,1000.);
#29869=VECTOR('',#141349,1000.);
#29870=VECTOR('',#141358,1000.);
#29871=VECTOR('',#141359,1000.);
#29872=VECTOR('',#141360,1000.);
#29873=VECTOR('',#141361,1000.);
#29874=VECTOR('',#141364,1000.);
#29875=VECTOR('',#141365,1000.);
#29876=VECTOR('',#141366,1000.);
#29877=VECTOR('',#141367,1000.);
#29878=VECTOR('',#141370,1000.);
#29879=VECTOR('',#141371,1000.);
#29880=VECTOR('',#141372,1000.);
#29881=VECTOR('',#141373,1000.);
#29882=VECTOR('',#141376,1000.);
#29883=VECTOR('',#141377,1000.);
#29884=VECTOR('',#141378,1000.);
#29885=VECTOR('',#141381,1000.);
#29886=VECTOR('',#141382,1000.);
#29887=VECTOR('',#141383,1000.);
#29888=VECTOR('',#141390,1000.);
#29889=VECTOR('',#141393,1000.);
#29890=VECTOR('',#141394,1000.);
#29891=VECTOR('',#141395,1000.);
#29892=VECTOR('',#141402,1000.);
#29893=VECTOR('',#141405,1000.);
#29894=VECTOR('',#141406,1000.);
#29895=VECTOR('',#141407,1000.);
#29896=VECTOR('',#141414,1000.);
#29897=VECTOR('',#141417,1000.);
#29898=VECTOR('',#141418,1000.);
#29899=VECTOR('',#141419,1000.);
#29900=VECTOR('',#141426,1000.);
#29901=VECTOR('',#141429,1000.);
#29902=VECTOR('',#141430,1000.);
#29903=VECTOR('',#141431,1000.);
#29904=VECTOR('',#141434,1000.);
#29905=VECTOR('',#141435,1000.);
#29906=VECTOR('',#141436,1000.);
#29907=VECTOR('',#141439,1000.);
#29908=VECTOR('',#141440,1000.);
#29909=VECTOR('',#141441,1000.);
#29910=VECTOR('',#141444,1000.);
#29911=VECTOR('',#141445,1000.);
#29912=VECTOR('',#141446,1000.);
#29913=VECTOR('',#141449,1000.);
#29914=VECTOR('',#141450,1000.);
#29915=VECTOR('',#141451,1000.);
#29916=VECTOR('',#141452,1000.);
#29917=VECTOR('',#141455,1000.);
#29918=VECTOR('',#141456,1000.);
#29919=VECTOR('',#141457,1000.);
#29920=VECTOR('',#141460,1000.);
#29921=VECTOR('',#141461,1000.);
#29922=VECTOR('',#141462,1000.);
#29923=VECTOR('',#141465,1000.);
#29924=VECTOR('',#141466,1000.);
#29925=VECTOR('',#141467,1000.);
#29926=VECTOR('',#141474,1000.);
#29927=VECTOR('',#141477,1000.);
#29928=VECTOR('',#141478,1000.);
#29929=VECTOR('',#141479,1000.);
#29930=VECTOR('',#141486,1000.);
#29931=VECTOR('',#141489,1000.);
#29932=VECTOR('',#141490,1000.);
#29933=VECTOR('',#141491,1000.);
#29934=VECTOR('',#141498,1000.);
#29935=VECTOR('',#141501,1000.);
#29936=VECTOR('',#141502,1000.);
#29937=VECTOR('',#141503,1000.);
#29938=VECTOR('',#141510,1000.);
#29939=VECTOR('',#141513,1000.);
#29940=VECTOR('',#141514,1000.);
#29941=VECTOR('',#141515,1000.);
#29942=VECTOR('',#141518,1000.);
#29943=VECTOR('',#141519,1000.);
#29944=VECTOR('',#141520,1000.);
#29945=VECTOR('',#141523,1000.);
#29946=VECTOR('',#141524,1000.);
#29947=VECTOR('',#141525,1000.);
#29948=VECTOR('',#141528,1000.);
#29949=VECTOR('',#141529,1000.);
#29950=VECTOR('',#141530,1000.);
#29951=VECTOR('',#141537,1000.);
#29952=VECTOR('',#141540,1000.);
#29953=VECTOR('',#141541,1000.);
#29954=VECTOR('',#141542,1000.);
#29955=VECTOR('',#141549,1000.);
#29956=VECTOR('',#141552,1000.);
#29957=VECTOR('',#141553,1000.);
#29958=VECTOR('',#141554,1000.);
#29959=VECTOR('',#141563,1000.);
#29960=VECTOR('',#141564,1000.);
#29961=VECTOR('',#141565,1000.);
#29962=VECTOR('',#141566,1000.);
#29963=VECTOR('',#141573,1000.);
#29964=VECTOR('',#141576,1000.);
#29965=VECTOR('',#141577,1000.);
#29966=VECTOR('',#141578,1000.);
#29967=VECTOR('',#141581,1000.);
#29968=VECTOR('',#141582,1000.);
#29969=VECTOR('',#141583,1000.);
#29970=VECTOR('',#141586,1000.);
#29971=VECTOR('',#141587,1000.);
#29972=VECTOR('',#141588,1000.);
#29973=VECTOR('',#141591,1000.);
#29974=VECTOR('',#141592,1000.);
#29975=VECTOR('',#141593,1000.);
#29976=VECTOR('',#141600,1000.);
#29977=VECTOR('',#141603,1000.);
#29978=VECTOR('',#141604,1000.);
#29979=VECTOR('',#141605,1000.);
#29980=VECTOR('',#141608,1000.);
#29981=VECTOR('',#141609,1000.);
#29982=VECTOR('',#141610,1000.);
#29983=VECTOR('',#141613,1000.);
#29984=VECTOR('',#141614,1000.);
#29985=VECTOR('',#141615,1000.);
#29986=VECTOR('',#141618,1000.);
#29987=VECTOR('',#141619,1000.);
#29988=VECTOR('',#141620,1000.);
#29989=VECTOR('',#141627,1000.);
#29990=VECTOR('',#141630,1000.);
#29991=VECTOR('',#141631,1000.);
#29992=VECTOR('',#141632,1000.);
#29993=VECTOR('',#141639,1000.);
#29994=VECTOR('',#141642,1000.);
#29995=VECTOR('',#141643,1000.);
#29996=VECTOR('',#141644,1000.);
#29997=VECTOR('',#141651,1000.);
#29998=VECTOR('',#141654,1000.);
#29999=VECTOR('',#141655,1000.);
#30000=VECTOR('',#141656,1000.);
#30001=VECTOR('',#141663,1000.);
#30002=VECTOR('',#141666,1000.);
#30003=VECTOR('',#141667,1000.);
#30004=VECTOR('',#141670,1000.);
#30005=VECTOR('',#141671,1000.);
#30006=VECTOR('',#141672,1000.);
#30007=VECTOR('',#141673,1000.);
#30008=VECTOR('',#141676,1000.);
#30009=VECTOR('',#141677,1000.);
#30010=VECTOR('',#141678,1000.);
#30011=VECTOR('',#141681,1000.);
#30012=VECTOR('',#141682,1000.);
#30013=VECTOR('',#141683,1000.);
#30014=VECTOR('',#141690,1000.);
#30015=VECTOR('',#141693,1000.);
#30016=VECTOR('',#141694,1000.);
#30017=VECTOR('',#141695,1000.);
#30018=VECTOR('',#141702,1000.);
#30019=VECTOR('',#141705,1000.);
#30020=VECTOR('',#141706,1000.);
#30021=VECTOR('',#141707,1000.);
#30022=VECTOR('',#141714,1000.);
#30023=VECTOR('',#141717,1000.);
#30024=VECTOR('',#141718,1000.);
#30025=VECTOR('',#141719,1000.);
#30026=VECTOR('',#141726,1000.);
#30027=VECTOR('',#141729,1000.);
#30028=VECTOR('',#141730,1000.);
#30029=VECTOR('',#141731,1000.);
#30030=VECTOR('',#141734,1000.);
#30031=VECTOR('',#141735,1000.);
#30032=VECTOR('',#141736,1000.);
#30033=VECTOR('',#141739,1000.);
#30034=VECTOR('',#141740,1000.);
#30035=VECTOR('',#141743,1000.);
#30036=VECTOR('',#141744,1000.);
#30037=VECTOR('',#141745,1000.);
#30038=VECTOR('',#141746,1000.);
#30039=VECTOR('',#141749,1000.);
#30040=VECTOR('',#141750,1000.);
#30041=VECTOR('',#141751,1000.);
#30042=VECTOR('',#141754,1000.);
#30043=VECTOR('',#141755,1000.);
#30044=VECTOR('',#141756,1000.);
#30045=VECTOR('',#141759,1000.);
#30046=VECTOR('',#141760,1000.);
#30047=VECTOR('',#141761,1000.);
#30048=VECTOR('',#141768,1000.);
#30049=VECTOR('',#141771,1000.);
#30050=VECTOR('',#141772,1000.);
#30051=VECTOR('',#141773,1000.);
#30052=VECTOR('',#141780,1000.);
#30053=VECTOR('',#141783,1000.);
#30054=VECTOR('',#141784,1000.);
#30055=VECTOR('',#141785,1000.);
#30056=VECTOR('',#141792,1000.);
#30057=VECTOR('',#141795,1000.);
#30058=VECTOR('',#141796,1000.);
#30059=VECTOR('',#141797,1000.);
#30060=VECTOR('',#141804,1000.);
#30061=VECTOR('',#141807,1000.);
#30062=VECTOR('',#141808,1000.);
#30063=VECTOR('',#141809,1000.);
#30064=VECTOR('',#141812,1000.);
#30065=VECTOR('',#141813,1000.);
#30066=VECTOR('',#141814,1000.);
#30067=VECTOR('',#141817,1000.);
#30068=VECTOR('',#141818,1000.);
#30069=VECTOR('',#141819,1000.);
#30070=VECTOR('',#141822,1000.);
#30071=VECTOR('',#141823,1000.);
#30072=VECTOR('',#141824,1000.);
#30073=VECTOR('',#141831,1000.);
#30074=VECTOR('',#141834,1000.);
#30075=VECTOR('',#141835,1000.);
#30076=VECTOR('',#141836,1000.);
#30077=VECTOR('',#141843,1000.);
#30078=VECTOR('',#141846,1000.);
#30079=VECTOR('',#141847,1000.);
#30080=VECTOR('',#141848,1000.);
#30081=VECTOR('',#141855,1000.);
#30082=VECTOR('',#141858,1000.);
#30083=VECTOR('',#141859,1000.);
#30084=VECTOR('',#141860,1000.);
#30085=VECTOR('',#141867,1000.);
#30086=VECTOR('',#141870,1000.);
#30087=VECTOR('',#141871,1000.);
#30088=VECTOR('',#141872,1000.);
#30089=VECTOR('',#141875,1000.);
#30090=VECTOR('',#141876,1000.);
#30091=VECTOR('',#141877,1000.);
#30092=VECTOR('',#141880,1000.);
#30093=VECTOR('',#141881,1000.);
#30094=VECTOR('',#141882,1000.);
#30095=VECTOR('',#141885,1000.);
#30096=VECTOR('',#141886,1000.);
#30097=VECTOR('',#141887,1000.);
#30098=VECTOR('',#141894,1000.);
#30099=VECTOR('',#141897,1000.);
#30100=VECTOR('',#141898,1000.);
#30101=VECTOR('',#141899,1000.);
#30102=VECTOR('',#141902,1000.);
#30103=VECTOR('',#141903,1000.);
#30104=VECTOR('',#141904,1000.);
#30105=VECTOR('',#141907,1000.);
#30106=VECTOR('',#141908,1000.);
#30107=VECTOR('',#141909,1000.);
#30108=VECTOR('',#141912,1000.);
#30109=VECTOR('',#141913,1000.);
#30110=VECTOR('',#141914,1000.);
#30111=VECTOR('',#141921,1000.);
#30112=VECTOR('',#141924,1000.);
#30113=VECTOR('',#141925,1000.);
#30114=VECTOR('',#141926,1000.);
#30115=VECTOR('',#141933,1000.);
#30116=VECTOR('',#141936,1000.);
#30117=VECTOR('',#141937,1000.);
#30118=VECTOR('',#141938,1000.);
#30119=VECTOR('',#141945,1000.);
#30120=VECTOR('',#141948,1000.);
#30121=VECTOR('',#141949,1000.);
#30122=VECTOR('',#141950,1000.);
#30123=VECTOR('',#141957,1000.);
#30124=VECTOR('',#141960,1000.);
#30125=VECTOR('',#141961,1000.);
#30126=VECTOR('',#141964,1000.);
#30127=VECTOR('',#141965,1000.);
#30128=VECTOR('',#141966,1000.);
#30129=VECTOR('',#141967,1000.);
#30130=VECTOR('',#141970,1000.);
#30131=VECTOR('',#141971,1000.);
#30132=VECTOR('',#141972,1000.);
#30133=VECTOR('',#141975,1000.);
#30134=VECTOR('',#141976,1000.);
#30135=VECTOR('',#141977,1000.);
#30136=VECTOR('',#141984,1000.);
#30137=VECTOR('',#141987,1000.);
#30138=VECTOR('',#141988,1000.);
#30139=VECTOR('',#141989,1000.);
#30140=VECTOR('',#141996,1000.);
#30141=VECTOR('',#141999,1000.);
#30142=VECTOR('',#142000,1000.);
#30143=VECTOR('',#142001,1000.);
#30144=VECTOR('',#142008,1000.);
#30145=VECTOR('',#142011,1000.);
#30146=VECTOR('',#142012,1000.);
#30147=VECTOR('',#142013,1000.);
#30148=VECTOR('',#142020,1000.);
#30149=VECTOR('',#142023,1000.);
#30150=VECTOR('',#142024,1000.);
#30151=VECTOR('',#142025,1000.);
#30152=VECTOR('',#142028,1000.);
#30153=VECTOR('',#142029,1000.);
#30154=VECTOR('',#142030,1000.);
#30155=VECTOR('',#142033,1000.);
#30156=VECTOR('',#142034,1000.);
#30157=VECTOR('',#142037,1000.);
#30158=VECTOR('',#142038,1000.);
#30159=VECTOR('',#142039,1000.);
#30160=VECTOR('',#142040,1000.);
#30161=VECTOR('',#142043,1000.);
#30162=VECTOR('',#142044,1000.);
#30163=VECTOR('',#142045,1000.);
#30164=VECTOR('',#142048,1000.);
#30165=VECTOR('',#142049,1000.);
#30166=VECTOR('',#142050,1000.);
#30167=VECTOR('',#142053,1000.);
#30168=VECTOR('',#142054,1000.);
#30169=VECTOR('',#142055,1000.);
#30170=VECTOR('',#142062,1000.);
#30171=VECTOR('',#142065,1000.);
#30172=VECTOR('',#142066,1000.);
#30173=VECTOR('',#142067,1000.);
#30174=VECTOR('',#142074,1000.);
#30175=VECTOR('',#142077,1000.);
#30176=VECTOR('',#142078,1000.);
#30177=VECTOR('',#142079,1000.);
#30178=VECTOR('',#142086,1000.);
#30179=VECTOR('',#142089,1000.);
#30180=VECTOR('',#142090,1000.);
#30181=VECTOR('',#142091,1000.);
#30182=VECTOR('',#142098,1000.);
#30183=VECTOR('',#142101,1000.);
#30184=VECTOR('',#142102,1000.);
#30185=VECTOR('',#142103,1000.);
#30186=VECTOR('',#142106,1000.);
#30187=VECTOR('',#142107,1000.);
#30188=VECTOR('',#142108,1000.);
#30189=VECTOR('',#142111,1000.);
#30190=VECTOR('',#142112,1000.);
#30191=VECTOR('',#142113,1000.);
#30192=VECTOR('',#142116,1000.);
#30193=VECTOR('',#142117,1000.);
#30194=VECTOR('',#142118,1000.);
#30195=VECTOR('',#142125,1000.);
#30196=VECTOR('',#142128,1000.);
#30197=VECTOR('',#142129,1000.);
#30198=VECTOR('',#142130,1000.);
#30199=VECTOR('',#142137,1000.);
#30200=VECTOR('',#142140,1000.);
#30201=VECTOR('',#142141,1000.);
#30202=VECTOR('',#142142,1000.);
#30203=VECTOR('',#142149,1000.);
#30204=VECTOR('',#142152,1000.);
#30205=VECTOR('',#142153,1000.);
#30206=VECTOR('',#142154,1000.);
#30207=VECTOR('',#142161,1000.);
#30208=VECTOR('',#142164,1000.);
#30209=VECTOR('',#142165,1000.);
#30210=VECTOR('',#142166,1000.);
#30211=VECTOR('',#142169,1000.);
#30212=VECTOR('',#142170,1000.);
#30213=VECTOR('',#142171,1000.);
#30214=VECTOR('',#142174,1000.);
#30215=VECTOR('',#142175,1000.);
#30216=VECTOR('',#142176,1000.);
#30217=VECTOR('',#142179,1000.);
#30218=VECTOR('',#142180,1000.);
#30219=VECTOR('',#142181,1000.);
#30220=VECTOR('',#142188,1000.);
#30221=VECTOR('',#142191,1000.);
#30222=VECTOR('',#142192,1000.);
#30223=VECTOR('',#142193,1000.);
#30224=VECTOR('',#142196,1000.);
#30225=VECTOR('',#142197,1000.);
#30226=VECTOR('',#142198,1000.);
#30227=VECTOR('',#142201,1000.);
#30228=VECTOR('',#142202,1000.);
#30229=VECTOR('',#142203,1000.);
#30230=VECTOR('',#142206,1000.);
#30231=VECTOR('',#142207,1000.);
#30232=VECTOR('',#142208,1000.);
#30233=VECTOR('',#142215,1000.);
#30234=VECTOR('',#142218,1000.);
#30235=VECTOR('',#142219,1000.);
#30236=VECTOR('',#142220,1000.);
#30237=VECTOR('',#142227,1000.);
#30238=VECTOR('',#142230,1000.);
#30239=VECTOR('',#142231,1000.);
#30240=VECTOR('',#142232,1000.);
#30241=VECTOR('',#142239,1000.);
#30242=VECTOR('',#142242,1000.);
#30243=VECTOR('',#142243,1000.);
#30244=VECTOR('',#142244,1000.);
#30245=VECTOR('',#142251,1000.);
#30246=VECTOR('',#142254,1000.);
#30247=VECTOR('',#142255,1000.);
#30248=VECTOR('',#142258,1000.);
#30249=VECTOR('',#142259,1000.);
#30250=VECTOR('',#142260,1000.);
#30251=VECTOR('',#142261,1000.);
#30252=VECTOR('',#142264,1000.);
#30253=VECTOR('',#142265,1000.);
#30254=VECTOR('',#142266,1000.);
#30255=VECTOR('',#142269,1000.);
#30256=VECTOR('',#142270,1000.);
#30257=VECTOR('',#142271,1000.);
#30258=VECTOR('',#142278,1000.);
#30259=VECTOR('',#142281,1000.);
#30260=VECTOR('',#142282,1000.);
#30261=VECTOR('',#142283,1000.);
#30262=VECTOR('',#142290,1000.);
#30263=VECTOR('',#142293,1000.);
#30264=VECTOR('',#142294,1000.);
#30265=VECTOR('',#142295,1000.);
#30266=VECTOR('',#142302,1000.);
#30267=VECTOR('',#142305,1000.);
#30268=VECTOR('',#142306,1000.);
#30269=VECTOR('',#142307,1000.);
#30270=VECTOR('',#142314,1000.);
#30271=VECTOR('',#142317,1000.);
#30272=VECTOR('',#142318,1000.);
#30273=VECTOR('',#142319,1000.);
#30274=VECTOR('',#142322,1000.);
#30275=VECTOR('',#142323,1000.);
#30276=VECTOR('',#142324,1000.);
#30277=VECTOR('',#142327,1000.);
#30278=VECTOR('',#142328,1000.);
#30279=VECTOR('',#142331,1000.);
#30280=VECTOR('',#142332,1000.);
#30281=VECTOR('',#142333,1000.);
#30282=VECTOR('',#142336,1000.);
#30283=VECTOR('',#142337,1000.);
#30284=VECTOR('',#142338,1000.);
#30285=VECTOR('',#142341,1000.);
#30286=VECTOR('',#142342,1000.);
#30287=VECTOR('',#142343,1000.);
#30288=VECTOR('',#142350,1000.);
#30289=VECTOR('',#142353,1000.);
#30290=VECTOR('',#142354,1000.);
#30291=VECTOR('',#142355,1000.);
#30292=VECTOR('',#142362,1000.);
#30293=VECTOR('',#142365,1000.);
#30294=VECTOR('',#142366,1000.);
#30295=VECTOR('',#142367,1000.);
#30296=VECTOR('',#142374,1000.);
#30297=VECTOR('',#142377,1000.);
#30298=VECTOR('',#142378,1000.);
#30299=VECTOR('',#142379,1000.);
#30300=VECTOR('',#142386,1000.);
#30301=VECTOR('',#142389,1000.);
#30302=VECTOR('',#142390,1000.);
#30303=VECTOR('',#142391,1000.);
#30304=VECTOR('',#142394,1000.);
#30305=VECTOR('',#142395,1000.);
#30306=VECTOR('',#142396,1000.);
#30307=VECTOR('',#142399,1000.);
#30308=VECTOR('',#142400,1000.);
#30309=VECTOR('',#142401,1000.);
#30310=VECTOR('',#142404,1000.);
#30311=VECTOR('',#142405,1000.);
#30312=VECTOR('',#142406,1000.);
#30313=VECTOR('',#142413,1000.);
#30314=VECTOR('',#142416,1000.);
#30315=VECTOR('',#142417,1000.);
#30316=VECTOR('',#142418,1000.);
#30317=VECTOR('',#142425,1000.);
#30318=VECTOR('',#142428,1000.);
#30319=VECTOR('',#142429,1000.);
#30320=VECTOR('',#142430,1000.);
#30321=VECTOR('',#142437,1000.);
#30322=VECTOR('',#142440,1000.);
#30323=VECTOR('',#142441,1000.);
#30324=VECTOR('',#142442,1000.);
#30325=VECTOR('',#142449,1000.);
#30326=VECTOR('',#142452,1000.);
#30327=VECTOR('',#142453,1000.);
#30328=VECTOR('',#142454,1000.);
#30329=VECTOR('',#142457,1000.);
#30330=VECTOR('',#142458,1000.);
#30331=VECTOR('',#142459,1000.);
#30332=VECTOR('',#142462,1000.);
#30333=VECTOR('',#142463,1000.);
#30334=VECTOR('',#142464,1000.);
#30335=VECTOR('',#142467,1000.);
#30336=VECTOR('',#142468,1000.);
#30337=VECTOR('',#142469,1000.);
#30338=VECTOR('',#142476,1000.);
#30339=VECTOR('',#142479,1000.);
#30340=VECTOR('',#142480,1000.);
#30341=VECTOR('',#142481,1000.);
#30342=VECTOR('',#142484,1000.);
#30343=VECTOR('',#142485,1000.);
#30344=VECTOR('',#142486,1000.);
#30345=VECTOR('',#142489,1000.);
#30346=VECTOR('',#142490,1000.);
#30347=VECTOR('',#142491,1000.);
#30348=VECTOR('',#142494,1000.);
#30349=VECTOR('',#142495,1000.);
#30350=VECTOR('',#142496,1000.);
#30351=VECTOR('',#142503,1000.);
#30352=VECTOR('',#142506,1000.);
#30353=VECTOR('',#142507,1000.);
#30354=VECTOR('',#142508,1000.);
#30355=VECTOR('',#142515,1000.);
#30356=VECTOR('',#142518,1000.);
#30357=VECTOR('',#142519,1000.);
#30358=VECTOR('',#142520,1000.);
#30359=VECTOR('',#142527,1000.);
#30360=VECTOR('',#142530,1000.);
#30361=VECTOR('',#142531,1000.);
#30362=VECTOR('',#142532,1000.);
#30363=VECTOR('',#142539,1000.);
#30364=VECTOR('',#142542,1000.);
#30365=VECTOR('',#142543,1000.);
#30366=VECTOR('',#142546,1000.);
#30367=VECTOR('',#142547,1000.);
#30368=VECTOR('',#142548,1000.);
#30369=VECTOR('',#142551,1000.);
#30370=VECTOR('',#142552,1000.);
#30371=VECTOR('',#142555,1000.);
#30372=VECTOR('',#142556,1000.);
#30373=VECTOR('',#142557,1000.);
#30374=VECTOR('',#142560,1000.);
#30375=VECTOR('',#142561,1000.);
#30376=VECTOR('',#142564,1000.);
#30377=VECTOR('',#142565,1000.);
#30378=VECTOR('',#142566,1000.);
#30379=VECTOR('',#142567,1000.);
#30380=VECTOR('',#142568,1000.);
#30381=VECTOR('',#142569,1000.);
#30382=VECTOR('',#142570,1000.);
#30383=VECTOR('',#142571,1000.);
#30384=VECTOR('',#142574,1000.);
#30385=VECTOR('',#142575,1000.);
#30386=VECTOR('',#142576,1000.);
#30387=VECTOR('',#142579,1000.);
#30388=VECTOR('',#142580,1000.);
#30389=VECTOR('',#142583,1000.);
#30390=VECTOR('',#142584,1000.);
#30391=VECTOR('',#142587,1000.);
#30392=VECTOR('',#142588,1000.);
#30393=VECTOR('',#142591,1000.);
#30394=VECTOR('',#142592,1000.);
#30395=VECTOR('',#142595,1000.);
#30396=VECTOR('',#142596,1000.);
#30397=VECTOR('',#142599,1000.);
#30398=VECTOR('',#142600,1000.);
#30399=VECTOR('',#142603,1000.);
#30400=VECTOR('',#142608,1000.);
#30401=VECTOR('',#142609,1000.);
#30402=VECTOR('',#142610,1000.);
#30403=VECTOR('',#142611,1000.);
#30404=VECTOR('',#142614,1000.);
#30405=VECTOR('',#142615,1000.);
#30406=VECTOR('',#142616,1000.);
#30407=VECTOR('',#142619,1000.);
#30408=VECTOR('',#142620,1000.);
#30409=VECTOR('',#142621,1000.);
#30410=VECTOR('',#142624,1000.);
#30411=VECTOR('',#142625,1000.);
#36279=CIRCLE('',#110988,6.3);
#36280=CIRCLE('',#110989,6.3);
#36281=CIRCLE('',#110991,9.9216);
#36282=CIRCLE('',#110992,6.29999999999999);
#36283=CIRCLE('',#110993,9.92159999999999);
#36284=CIRCLE('',#110994,6.29999999999999);
#36285=CIRCLE('',#110995,9.92159999999999);
#36286=CIRCLE('',#110996,6.3);
#36287=CIRCLE('',#110997,9.92159999999999);
#36288=CIRCLE('',#111001,9.92159999999999);
#36289=CIRCLE('',#111004,6.3);
#36290=CIRCLE('',#111007,9.92159999999999);
#36291=CIRCLE('',#111010,6.29999999999999);
#36292=CIRCLE('',#111013,9.92159999999999);
#36293=CIRCLE('',#111016,6.29999999999999);
#36294=CIRCLE('',#111019,9.9216);
#36295=CIRCLE('',#111022,1.8);
#36296=CIRCLE('',#111023,1.8);
#36297=CIRCLE('',#111024,1.8);
#36298=CIRCLE('',#111025,1.8);
#36299=CIRCLE('',#111028,1.8);
#36300=CIRCLE('',#111031,1.8);
#36301=CIRCLE('',#111034,1.8);
#36302=CIRCLE('',#111037,1.8);
#36303=CIRCLE('',#111040,2.7);
#36304=CIRCLE('',#111041,2.7);
#36305=CIRCLE('',#111042,2.7);
#36306=CIRCLE('',#111043,2.69999999999999);
#36307=CIRCLE('',#111044,2.69999999999999);
#36308=CIRCLE('',#111045,2.7);
#36309=CIRCLE('',#111046,2.7);
#36310=CIRCLE('',#111047,2.7);
#36311=CIRCLE('',#111048,2.7);
#36312=CIRCLE('',#111049,2.7);
#36313=CIRCLE('',#111050,2.69999999999999);
#36314=CIRCLE('',#111051,2.69999999999999);
#36315=CIRCLE('',#111052,2.7);
#36316=CIRCLE('',#111053,2.7);
#36317=CIRCLE('',#111054,2.7);
#36318=CIRCLE('',#111055,2.69999999999999);
#36319=CIRCLE('',#111056,2.7);
#36320=CIRCLE('',#111057,2.69999999999999);
#36321=CIRCLE('',#111058,2.7);
#36322=CIRCLE('',#111059,2.7);
#36323=CIRCLE('',#111060,2.7);
#36324=CIRCLE('',#111061,2.7);
#36325=CIRCLE('',#111062,2.69999999999999);
#36326=CIRCLE('',#111063,2.69999999999999);
#36327=CIRCLE('',#111065,2.7);
#36328=CIRCLE('',#111066,2.7);
#36329=CIRCLE('',#111067,2.69999999999999);
#36330=CIRCLE('',#111068,2.69999999999999);
#36331=CIRCLE('',#111069,2.69999999999999);
#36332=CIRCLE('',#111070,2.7);
#36333=CIRCLE('',#111071,2.7);
#36334=CIRCLE('',#111072,2.7);
#36335=CIRCLE('',#111073,2.69999999999999);
#36336=CIRCLE('',#111074,2.69999999999999);
#36337=CIRCLE('',#111075,2.69999999999999);
#36338=CIRCLE('',#111076,2.7);
#36339=CIRCLE('',#111077,2.7);
#36340=CIRCLE('',#111078,2.7);
#36341=CIRCLE('',#111079,2.7);
#36342=CIRCLE('',#111080,2.69999999999999);
#36343=CIRCLE('',#111081,2.69999999999999);
#36344=CIRCLE('',#111082,2.7);
#36345=CIRCLE('',#111083,2.7);
#36346=CIRCLE('',#111084,2.7);
#36347=CIRCLE('',#111085,2.69999999999999);
#36348=CIRCLE('',#111086,2.69999999999999);
#36349=CIRCLE('',#111087,2.69999999999999);
#36350=CIRCLE('',#111088,2.7);
#36351=CIRCLE('',#111146,6.29999999999999);
#36352=CIRCLE('',#111147,6.29999999999999);
#36353=CIRCLE('',#111149,9.9216);
#36354=CIRCLE('',#111150,6.29999999999999);
#36355=CIRCLE('',#111151,9.92159999999999);
#36356=CIRCLE('',#111152,9.92159999999998);
#36357=CIRCLE('',#111153,6.3);
#36358=CIRCLE('',#111154,9.92159999999999);
#36359=CIRCLE('',#111155,6.3);
#36360=CIRCLE('',#111158,6.29999999999999);
#36361=CIRCLE('',#111161,9.92159999999999);
#36362=CIRCLE('',#111164,6.3);
#36363=CIRCLE('',#111167,9.92159999999998);
#36364=CIRCLE('',#111171,9.92159999999999);
#36365=CIRCLE('',#111174,6.29999999999999);
#36366=CIRCLE('',#111177,9.9216);
#36367=CIRCLE('',#111180,1.8);
#36368=CIRCLE('',#111181,1.8);
#36369=CIRCLE('',#111182,1.8);
#36370=CIRCLE('',#111183,1.8);
#36371=CIRCLE('',#111186,1.8);
#36372=CIRCLE('',#111189,1.8);
#36373=CIRCLE('',#111192,1.8);
#36374=CIRCLE('',#111195,1.8);
#36375=CIRCLE('',#111198,6.29999999999999);
#36376=CIRCLE('',#111199,6.29999999999999);
#36377=CIRCLE('',#111201,9.9216);
#36378=CIRCLE('',#111202,9.92159999999999);
#36379=CIRCLE('',#111203,6.29999999999999);
#36380=CIRCLE('',#111204,9.92159999999998);
#36381=CIRCLE('',#111205,6.3);
#36382=CIRCLE('',#111206,9.92159999999999);
#36383=CIRCLE('',#111207,6.3);
#36384=CIRCLE('',#111210,6.3);
#36385=CIRCLE('',#111213,9.92159999999999);
#36386=CIRCLE('',#111216,6.3);
#36387=CIRCLE('',#111219,9.92159999999999);
#36388=CIRCLE('',#111222,6.29999999999999);
#36389=CIRCLE('',#111225,9.92159999999999);
#36390=CIRCLE('',#111229,9.92159999999999);
#36391=CIRCLE('',#111232,1.8);
#36392=CIRCLE('',#111233,1.8);
#36393=CIRCLE('',#111234,1.8);
#36394=CIRCLE('',#111235,1.8);
#36395=CIRCLE('',#111238,1.8);
#36396=CIRCLE('',#111241,1.8);
#36397=CIRCLE('',#111244,1.8);
#36398=CIRCLE('',#111247,1.8);
#36399=CIRCLE('',#111250,6.29999999999999);
#36400=CIRCLE('',#111251,6.29999999999999);
#36401=CIRCLE('',#111253,9.9216);
#36402=CIRCLE('',#111254,9.92159999999999);
#36403=CIRCLE('',#111255,6.29999999999999);
#36404=CIRCLE('',#111256,9.92159999999999);
#36405=CIRCLE('',#111257,6.3);
#36406=CIRCLE('',#111258,9.92159999999999);
#36407=CIRCLE('',#111259,6.3);
#36408=CIRCLE('',#111262,6.3);
#36409=CIRCLE('',#111265,9.92159999999999);
#36410=CIRCLE('',#111268,6.3);
#36411=CIRCLE('',#111271,9.92159999999999);
#36412=CIRCLE('',#111274,6.29999999999999);
#36413=CIRCLE('',#111277,9.92159999999999);
#36414=CIRCLE('',#111281,9.9216);
#36415=CIRCLE('',#111284,1.8);
#36416=CIRCLE('',#111285,1.8);
#36417=CIRCLE('',#111286,1.8);
#36418=CIRCLE('',#111287,1.8);
#36419=CIRCLE('',#111290,1.8);
#36420=CIRCLE('',#111293,1.8);
#36421=CIRCLE('',#111296,1.8);
#36422=CIRCLE('',#111299,1.8);
#36423=CIRCLE('',#111307,0.899999999999998);
#36424=CIRCLE('',#111308,0.899999999999998);
#36425=CIRCLE('',#111311,0.899999999999998);
#36426=CIRCLE('',#111312,0.899999999999998);
#36427=CIRCLE('',#111315,0.899999999999998);
#36428=CIRCLE('',#111316,0.899999999999998);
#36429=CIRCLE('',#111319,0.899999999999991);
#36430=CIRCLE('',#111320,0.899999999999991);
#36431=CIRCLE('',#111330,0.899999999999995);
#36432=CIRCLE('',#111331,0.899999999999995);
#36433=CIRCLE('',#111334,0.900000000000001);
#36434=CIRCLE('',#111335,0.900000000000001);
#36435=CIRCLE('',#111338,0.899999999999996);
#36436=CIRCLE('',#111339,0.899999999999996);
#36437=CIRCLE('',#111342,0.899999999999998);
#36438=CIRCLE('',#111343,0.899999999999998);
#36439=CIRCLE('',#111349,0.899999999999998);
#36440=CIRCLE('',#111350,0.899999999999998);
#36441=CIRCLE('',#111353,0.899999999999998);
#36442=CIRCLE('',#111354,0.899999999999998);
#36443=CIRCLE('',#111357,0.899999999999991);
#36444=CIRCLE('',#111358,0.899999999999991);
#36445=CIRCLE('',#111361,0.899999999999998);
#36446=CIRCLE('',#111362,0.899999999999998);
#36447=CIRCLE('',#111368,3.65760000000007);
#36448=CIRCLE('',#111369,3.65760000000007);
#36449=CIRCLE('',#111375,0.899999999999991);
#36450=CIRCLE('',#111376,0.899999999999991);
#36451=CIRCLE('',#111379,0.899999999999998);
#36452=CIRCLE('',#111380,0.899999999999998);
#36453=CIRCLE('',#111383,0.899999999999998);
#36454=CIRCLE('',#111384,0.899999999999998);
#36455=CIRCLE('',#111387,0.899999999999998);
#36456=CIRCLE('',#111388,0.899999999999998);
#36457=CIRCLE('',#111394,0.899999999999998);
#36458=CIRCLE('',#111395,0.899999999999998);
#36459=CIRCLE('',#111398,0.899999999999996);
#36460=CIRCLE('',#111399,0.899999999999998);
#36461=CIRCLE('',#111402,0.900000000000001);
#36462=CIRCLE('',#111403,0.899999999999998);
#36463=CIRCLE('',#111406,0.899999999999995);
#36464=CIRCLE('',#111407,0.899999999999991);
#36465=CIRCLE('',#111416,0.899999999999991);
#36466=CIRCLE('',#111417,0.899999999999995);
#36467=CIRCLE('',#111420,0.899999999999998);
#36468=CIRCLE('',#111421,0.900000000000001);
#36469=CIRCLE('',#111424,0.899999999999998);
#36470=CIRCLE('',#111425,0.899999999999996);
#36471=CIRCLE('',#111428,0.899999999999998);
#36472=CIRCLE('',#111429,0.899999999999998);
#36473=CIRCLE('',#111435,0.899999999999998);
#36474=CIRCLE('',#111436,0.899999999999998);
#36475=CIRCLE('',#111439,0.899999999999998);
#36476=CIRCLE('',#111440,0.899999999999998);
#36477=CIRCLE('',#111443,0.899999999999991);
#36478=CIRCLE('',#111444,0.899999999999991);
#36479=CIRCLE('',#111447,0.899999999999998);
#36480=CIRCLE('',#111448,0.899999999999998);
#36481=CIRCLE('',#111454,3.65760000000007);
#36482=CIRCLE('',#111455,3.65760000000007);
#36483=CIRCLE('',#111461,0.899999999999991);
#36484=CIRCLE('',#111462,0.899999999999991);
#36485=CIRCLE('',#111465,0.899999999999998);
#36486=CIRCLE('',#111466,0.899999999999998);
#36487=CIRCLE('',#111469,0.899999999999998);
#36488=CIRCLE('',#111470,0.899999999999998);
#36489=CIRCLE('',#111473,0.899999999999998);
#36490=CIRCLE('',#111474,0.899999999999998);
#36491=CIRCLE('',#111480,0.899999999999998);
#36492=CIRCLE('',#111481,0.899999999999998);
#36493=CIRCLE('',#111484,0.899999999999998);
#36494=CIRCLE('',#111485,0.899999999999998);
#36495=CIRCLE('',#111488,0.899999999999998);
#36496=CIRCLE('',#111489,0.899999999999998);
#36497=CIRCLE('',#111492,0.899999999999991);
#36498=CIRCLE('',#111493,0.899999999999991);
#36499=CIRCLE('',#111502,0.899999999999995);
#36500=CIRCLE('',#111503,0.899999999999995);
#36501=CIRCLE('',#111506,0.900000000000001);
#36502=CIRCLE('',#111507,0.900000000000001);
#36503=CIRCLE('',#111510,0.899999999999996);
#36504=CIRCLE('',#111511,0.899999999999996);
#36505=CIRCLE('',#111514,0.899999999999998);
#36506=CIRCLE('',#111515,0.899999999999998);
#36507=CIRCLE('',#111521,0.899999999999998);
#36508=CIRCLE('',#111522,0.899999999999998);
#36509=CIRCLE('',#111525,0.899999999999998);
#36510=CIRCLE('',#111526,0.899999999999998);
#36511=CIRCLE('',#111529,0.899999999999991);
#36512=CIRCLE('',#111530,0.899999999999991);
#36513=CIRCLE('',#111533,0.899999999999998);
#36514=CIRCLE('',#111534,0.899999999999998);
#36515=CIRCLE('',#111540,3.65760000000007);
#36516=CIRCLE('',#111541,3.65760000000007);
#36517=CIRCLE('',#111547,0.899999999999991);
#36518=CIRCLE('',#111548,0.899999999999991);
#36519=CIRCLE('',#111551,0.899999999999998);
#36520=CIRCLE('',#111552,0.899999999999998);
#36521=CIRCLE('',#111555,0.899999999999998);
#36522=CIRCLE('',#111556,0.899999999999998);
#36523=CIRCLE('',#111559,0.899999999999998);
#36524=CIRCLE('',#111560,0.899999999999998);
#36525=CIRCLE('',#111566,0.899999999999998);
#36526=CIRCLE('',#111567,0.899999999999998);
#36527=CIRCLE('',#111570,0.899999999999996);
#36528=CIRCLE('',#111571,0.899999999999998);
#36529=CIRCLE('',#111574,0.900000000000001);
#36530=CIRCLE('',#111575,0.899999999999998);
#36531=CIRCLE('',#111578,0.899999999999995);
#36532=CIRCLE('',#111579,0.899999999999991);
#36533=CIRCLE('',#111587,0.899999999999991);
#36534=CIRCLE('',#111588,0.899999999999995);
#36535=CIRCLE('',#111591,0.899999999999998);
#36536=CIRCLE('',#111592,0.900000000000001);
#36537=CIRCLE('',#111595,0.899999999999998);
#36538=CIRCLE('',#111596,0.899999999999996);
#36539=CIRCLE('',#111599,0.899999999999998);
#36540=CIRCLE('',#111600,0.899999999999998);
#36541=CIRCLE('',#111606,0.899999999999998);
#36542=CIRCLE('',#111607,0.899999999999998);
#36543=CIRCLE('',#111610,0.899999999999998);
#36544=CIRCLE('',#111611,0.899999999999998);
#36545=CIRCLE('',#111614,0.899999999999991);
#36546=CIRCLE('',#111615,0.899999999999991);
#36547=CIRCLE('',#111618,0.899999999999998);
#36548=CIRCLE('',#111619,0.899999999999998);
#36549=CIRCLE('',#111625,3.65760000000007);
#36550=CIRCLE('',#111626,3.65760000000007);
#36551=CIRCLE('',#111632,0.899999999999991);
#36552=CIRCLE('',#111633,0.899999999999991);
#36553=CIRCLE('',#111636,0.899999999999998);
#36554=CIRCLE('',#111637,0.899999999999998);
#36555=CIRCLE('',#111640,0.899999999999998);
#36556=CIRCLE('',#111641,0.899999999999998);
#36557=CIRCLE('',#111644,0.899999999999998);
#36558=CIRCLE('',#111645,0.899999999999998);
#44735=VERTEX_POINT('',#274152);
#44736=VERTEX_POINT('',#274153);
#44737=VERTEX_POINT('',#274155);
#44738=VERTEX_POINT('',#274157);
#44739=VERTEX_POINT('',#274161);
#44740=VERTEX_POINT('',#274162);
#44741=VERTEX_POINT('',#274164);
#44742=VERTEX_POINT('',#274166);
#44743=VERTEX_POINT('',#274168);
#44744=VERTEX_POINT('',#274170);
#44745=VERTEX_POINT('',#274172);
#44746=VERTEX_POINT('',#274174);
#44747=VERTEX_POINT('',#274176);
#44748=VERTEX_POINT('',#274178);
#44749=VERTEX_POINT('',#274180);
#44750=VERTEX_POINT('',#274182);
#44751=VERTEX_POINT('',#274184);
#44752=VERTEX_POINT('',#274186);
#44753=VERTEX_POINT('',#274191);
#44754=VERTEX_POINT('',#274195);
#44755=VERTEX_POINT('',#274199);
#44756=VERTEX_POINT('',#274203);
#44757=VERTEX_POINT('',#274207);
#44758=VERTEX_POINT('',#274211);
#44759=VERTEX_POINT('',#274215);
#44760=VERTEX_POINT('',#274219);
#44761=VERTEX_POINT('',#274223);
#44762=VERTEX_POINT('',#274227);
#44763=VERTEX_POINT('',#274231);
#44764=VERTEX_POINT('',#274235);
#44765=VERTEX_POINT('',#274239);
#44766=VERTEX_POINT('',#274243);
#44767=VERTEX_POINT('',#274250);
#44768=VERTEX_POINT('',#274251);
#44769=VERTEX_POINT('',#274253);
#44770=VERTEX_POINT('',#274255);
#44771=VERTEX_POINT('',#274257);
#44772=VERTEX_POINT('',#274259);
#44773=VERTEX_POINT('',#274261);
#44774=VERTEX_POINT('',#274263);
#44775=VERTEX_POINT('',#274267);
#44776=VERTEX_POINT('',#274269);
#44777=VERTEX_POINT('',#274273);
#44778=VERTEX_POINT('',#274277);
#44779=VERTEX_POINT('',#274281);
#44780=VERTEX_POINT('',#274285);
#44781=VERTEX_POINT('',#274289);
#44782=VERTEX_POINT('',#274293);
#44783=VERTEX_POINT('',#274300);
#44784=VERTEX_POINT('',#274301);
#44785=VERTEX_POINT('',#274303);
#44786=VERTEX_POINT('',#274305);
#44787=VERTEX_POINT('',#274307);
#44788=VERTEX_POINT('',#274309);
#44789=VERTEX_POINT('',#274311);
#44790=VERTEX_POINT('',#274313);
#44791=VERTEX_POINT('',#274315);
#44792=VERTEX_POINT('',#274317);
#44793=VERTEX_POINT('',#274319);
#44794=VERTEX_POINT('',#274321);
#44795=VERTEX_POINT('',#274323);
#44796=VERTEX_POINT('',#274325);
#44797=VERTEX_POINT('',#274327);
#44798=VERTEX_POINT('',#274329);
#44799=VERTEX_POINT('',#274331);
#44800=VERTEX_POINT('',#274333);
#44801=VERTEX_POINT('',#274335);
#44802=VERTEX_POINT('',#274337);
#44803=VERTEX_POINT('',#274339);
#44804=VERTEX_POINT('',#274341);
#44805=VERTEX_POINT('',#274343);
#44806=VERTEX_POINT('',#274345);
#44807=VERTEX_POINT('',#274347);
#44808=VERTEX_POINT('',#274349);
#44809=VERTEX_POINT('',#274351);
#44810=VERTEX_POINT('',#274353);
#44811=VERTEX_POINT('',#274355);
#44812=VERTEX_POINT('',#274357);
#44813=VERTEX_POINT('',#274359);
#44814=VERTEX_POINT('',#274361);
#44815=VERTEX_POINT('',#274363);
#44816=VERTEX_POINT('',#274365);
#44817=VERTEX_POINT('',#274367);
#44818=VERTEX_POINT('',#274369);
#44819=VERTEX_POINT('',#274371);
#44820=VERTEX_POINT('',#274373);
#44821=VERTEX_POINT('',#274375);
#44822=VERTEX_POINT('',#274377);
#44823=VERTEX_POINT('',#274379);
#44824=VERTEX_POINT('',#274381);
#44825=VERTEX_POINT('',#274383);
#44826=VERTEX_POINT('',#274385);
#44827=VERTEX_POINT('',#274387);
#44828=VERTEX_POINT('',#274389);
#44829=VERTEX_POINT('',#274391);
#44830=VERTEX_POINT('',#274393);
#44831=VERTEX_POINT('',#274395);
#44832=VERTEX_POINT('',#274397);
#44833=VERTEX_POINT('',#274399);
#44834=VERTEX_POINT('',#274401);
#44835=VERTEX_POINT('',#274403);
#44836=VERTEX_POINT('',#274405);
#44837=VERTEX_POINT('',#274407);
#44838=VERTEX_POINT('',#274409);
#44839=VERTEX_POINT('',#274413);
#44840=VERTEX_POINT('',#274414);
#44841=VERTEX_POINT('',#274416);
#44842=VERTEX_POINT('',#274418);
#44843=VERTEX_POINT('',#274420);
#44844=VERTEX_POINT('',#274422);
#44845=VERTEX_POINT('',#274424);
#44846=VERTEX_POINT('',#274426);
#44847=VERTEX_POINT('',#274428);
#44848=VERTEX_POINT('',#274430);
#44849=VERTEX_POINT('',#274432);
#44850=VERTEX_POINT('',#274434);
#44851=VERTEX_POINT('',#274436);
#44852=VERTEX_POINT('',#274438);
#44853=VERTEX_POINT('',#274440);
#44854=VERTEX_POINT('',#274442);
#44855=VERTEX_POINT('',#274444);
#44856=VERTEX_POINT('',#274446);
#44857=VERTEX_POINT('',#274448);
#44858=VERTEX_POINT('',#274450);
#44859=VERTEX_POINT('',#274452);
#44860=VERTEX_POINT('',#274454);
#44861=VERTEX_POINT('',#274456);
#44862=VERTEX_POINT('',#274458);
#44863=VERTEX_POINT('',#274460);
#44864=VERTEX_POINT('',#274462);
#44865=VERTEX_POINT('',#274464);
#44866=VERTEX_POINT('',#274466);
#44867=VERTEX_POINT('',#274468);
#44868=VERTEX_POINT('',#274470);
#44869=VERTEX_POINT('',#274472);
#44870=VERTEX_POINT('',#274474);
#44871=VERTEX_POINT('',#274476);
#44872=VERTEX_POINT('',#274478);
#44873=VERTEX_POINT('',#274480);
#44874=VERTEX_POINT('',#274482);
#44875=VERTEX_POINT('',#274484);
#44876=VERTEX_POINT('',#274486);
#44877=VERTEX_POINT('',#274488);
#44878=VERTEX_POINT('',#274490);
#44879=VERTEX_POINT('',#274492);
#44880=VERTEX_POINT('',#274494);
#44881=VERTEX_POINT('',#274496);
#44882=VERTEX_POINT('',#274498);
#44883=VERTEX_POINT('',#274500);
#44884=VERTEX_POINT('',#274502);
#44885=VERTEX_POINT('',#274504);
#44886=VERTEX_POINT('',#274506);
#44887=VERTEX_POINT('',#274508);
#44888=VERTEX_POINT('',#274510);
#44889=VERTEX_POINT('',#274512);
#44890=VERTEX_POINT('',#274514);
#44891=VERTEX_POINT('',#274516);
#44892=VERTEX_POINT('',#274518);
#44893=VERTEX_POINT('',#274520);
#44894=VERTEX_POINT('',#274522);
#44895=VERTEX_POINT('',#274638);
#44896=VERTEX_POINT('',#274639);
#44897=VERTEX_POINT('',#274641);
#44898=VERTEX_POINT('',#274643);
#44899=VERTEX_POINT('',#274647);
#44900=VERTEX_POINT('',#274648);
#44901=VERTEX_POINT('',#274650);
#44902=VERTEX_POINT('',#274652);
#44903=VERTEX_POINT('',#274654);
#44904=VERTEX_POINT('',#274656);
#44905=VERTEX_POINT('',#274659);
#44906=VERTEX_POINT('',#274661);
#44907=VERTEX_POINT('',#274663);
#44908=VERTEX_POINT('',#274665);
#44909=VERTEX_POINT('',#274667);
#44910=VERTEX_POINT('',#274669);
#44911=VERTEX_POINT('',#274671);
#44912=VERTEX_POINT('',#274673);
#44913=VERTEX_POINT('',#274677);
#44914=VERTEX_POINT('',#274679);
#44915=VERTEX_POINT('',#274683);
#44916=VERTEX_POINT('',#274687);
#44917=VERTEX_POINT('',#274691);
#44918=VERTEX_POINT('',#274695);
#44919=VERTEX_POINT('',#274699);
#44920=VERTEX_POINT('',#274703);
#44921=VERTEX_POINT('',#274707);
#44922=VERTEX_POINT('',#274713);
#44923=VERTEX_POINT('',#274717);
#44924=VERTEX_POINT('',#274721);
#44925=VERTEX_POINT('',#274725);
#44926=VERTEX_POINT('',#274729);
#44927=VERTEX_POINT('',#274736);
#44928=VERTEX_POINT('',#274737);
#44929=VERTEX_POINT('',#274739);
#44930=VERTEX_POINT('',#274741);
#44931=VERTEX_POINT('',#274743);
#44932=VERTEX_POINT('',#274745);
#44933=VERTEX_POINT('',#274747);
#44934=VERTEX_POINT('',#274749);
#44935=VERTEX_POINT('',#274753);
#44936=VERTEX_POINT('',#274755);
#44937=VERTEX_POINT('',#274759);
#44938=VERTEX_POINT('',#274763);
#44939=VERTEX_POINT('',#274767);
#44940=VERTEX_POINT('',#274771);
#44941=VERTEX_POINT('',#274775);
#44942=VERTEX_POINT('',#274779);
#44943=VERTEX_POINT('',#274786);
#44944=VERTEX_POINT('',#274787);
#44945=VERTEX_POINT('',#274789);
#44946=VERTEX_POINT('',#274791);
#44947=VERTEX_POINT('',#274795);
#44948=VERTEX_POINT('',#274796);
#44949=VERTEX_POINT('',#274799);
#44950=VERTEX_POINT('',#274801);
#44951=VERTEX_POINT('',#274803);
#44952=VERTEX_POINT('',#274805);
#44953=VERTEX_POINT('',#274807);
#44954=VERTEX_POINT('',#274809);
#44955=VERTEX_POINT('',#274811);
#44956=VERTEX_POINT('',#274813);
#44957=VERTEX_POINT('',#274815);
#44958=VERTEX_POINT('',#274817);
#44959=VERTEX_POINT('',#274819);
#44960=VERTEX_POINT('',#274821);
#44961=VERTEX_POINT('',#274825);
#44962=VERTEX_POINT('',#274827);
#44963=VERTEX_POINT('',#274831);
#44964=VERTEX_POINT('',#274835);
#44965=VERTEX_POINT('',#274839);
#44966=VERTEX_POINT('',#274843);
#44967=VERTEX_POINT('',#274847);
#44968=VERTEX_POINT('',#274851);
#44969=VERTEX_POINT('',#274855);
#44970=VERTEX_POINT('',#274859);
#44971=VERTEX_POINT('',#274863);
#44972=VERTEX_POINT('',#274867);
#44973=VERTEX_POINT('',#274871);
#44974=VERTEX_POINT('',#274877);
#44975=VERTEX_POINT('',#274884);
#44976=VERTEX_POINT('',#274885);
#44977=VERTEX_POINT('',#274887);
#44978=VERTEX_POINT('',#274889);
#44979=VERTEX_POINT('',#274891);
#44980=VERTEX_POINT('',#274893);
#44981=VERTEX_POINT('',#274895);
#44982=VERTEX_POINT('',#274897);
#44983=VERTEX_POINT('',#274901);
#44984=VERTEX_POINT('',#274903);
#44985=VERTEX_POINT('',#274907);
#44986=VERTEX_POINT('',#274911);
#44987=VERTEX_POINT('',#274915);
#44988=VERTEX_POINT('',#274919);
#44989=VERTEX_POINT('',#274923);
#44990=VERTEX_POINT('',#274927);
#44991=VERTEX_POINT('',#274934);
#44992=VERTEX_POINT('',#274935);
#44993=VERTEX_POINT('',#274937);
#44994=VERTEX_POINT('',#274939);
#44995=VERTEX_POINT('',#274943);
#44996=VERTEX_POINT('',#274944);
#44997=VERTEX_POINT('',#274947);
#44998=VERTEX_POINT('',#274949);
#44999=VERTEX_POINT('',#274951);
#45000=VERTEX_POINT('',#274953);
#45001=VERTEX_POINT('',#274955);
#45002=VERTEX_POINT('',#274957);
#45003=VERTEX_POINT('',#274959);
#45004=VERTEX_POINT('',#274961);
#45005=VERTEX_POINT('',#274963);
#45006=VERTEX_POINT('',#274965);
#45007=VERTEX_POINT('',#274967);
#45008=VERTEX_POINT('',#274969);
#45009=VERTEX_POINT('',#274973);
#45010=VERTEX_POINT('',#274975);
#45011=VERTEX_POINT('',#274979);
#45012=VERTEX_POINT('',#274983);
#45013=VERTEX_POINT('',#274987);
#45014=VERTEX_POINT('',#274991);
#45015=VERTEX_POINT('',#274995);
#45016=VERTEX_POINT('',#274999);
#45017=VERTEX_POINT('',#275003);
#45018=VERTEX_POINT('',#275007);
#45019=VERTEX_POINT('',#275011);
#45020=VERTEX_POINT('',#275015);
#45021=VERTEX_POINT('',#275019);
#45022=VERTEX_POINT('',#275025);
#45023=VERTEX_POINT('',#275032);
#45024=VERTEX_POINT('',#275033);
#45025=VERTEX_POINT('',#275035);
#45026=VERTEX_POINT('',#275037);
#45027=VERTEX_POINT('',#275039);
#45028=VERTEX_POINT('',#275041);
#45029=VERTEX_POINT('',#275043);
#45030=VERTEX_POINT('',#275045);
#45031=VERTEX_POINT('',#275049);
#45032=VERTEX_POINT('',#275051);
#45033=VERTEX_POINT('',#275055);
#45034=VERTEX_POINT('',#275059);
#45035=VERTEX_POINT('',#275063);
#45036=VERTEX_POINT('',#275067);
#45037=VERTEX_POINT('',#275071);
#45038=VERTEX_POINT('',#275075);
#45039=VERTEX_POINT('',#275082);
#45040=VERTEX_POINT('',#275083);
#45041=VERTEX_POINT('',#275085);
#45042=VERTEX_POINT('',#275087);
#45043=VERTEX_POINT('',#275091);
#45044=VERTEX_POINT('',#275092);
#45045=VERTEX_POINT('',#275094);
#45046=VERTEX_POINT('',#275096);
#45047=VERTEX_POINT('',#275100);
#45048=VERTEX_POINT('',#275101);
#45049=VERTEX_POINT('',#275103);
#45050=VERTEX_POINT('',#275105);
#45051=VERTEX_POINT('',#275109);
#45052=VERTEX_POINT('',#275111);
#45053=VERTEX_POINT('',#275115);
#45054=VERTEX_POINT('',#275117);
#45055=VERTEX_POINT('',#275121);
#45056=VERTEX_POINT('',#275123);
#45057=VERTEX_POINT('',#275127);
#45058=VERTEX_POINT('',#275129);
#45059=VERTEX_POINT('',#275133);
#45060=VERTEX_POINT('',#275135);
#45061=VERTEX_POINT('',#275139);
#45062=VERTEX_POINT('',#275141);
#45063=VERTEX_POINT('',#275145);
#45064=VERTEX_POINT('',#275147);
#45065=VERTEX_POINT('',#275151);
#45066=VERTEX_POINT('',#275153);
#45067=VERTEX_POINT('',#275157);
#45068=VERTEX_POINT('',#275159);
#45069=VERTEX_POINT('',#275163);
#45070=VERTEX_POINT('',#275165);
#45071=VERTEX_POINT('',#275169);
#45072=VERTEX_POINT('',#275171);
#45073=VERTEX_POINT('',#275175);
#45074=VERTEX_POINT('',#275177);
#45075=VERTEX_POINT('',#275181);
#45076=VERTEX_POINT('',#275183);
#45077=VERTEX_POINT('',#275187);
#45078=VERTEX_POINT('',#275188);
#45079=VERTEX_POINT('',#275190);
#45080=VERTEX_POINT('',#275192);
#45081=VERTEX_POINT('',#275196);
#45082=VERTEX_POINT('',#275198);
#45083=VERTEX_POINT('',#275202);
#45084=VERTEX_POINT('',#275204);
#45085=VERTEX_POINT('',#275208);
#45086=VERTEX_POINT('',#275210);
#45087=VERTEX_POINT('',#275214);
#45088=VERTEX_POINT('',#275216);
#45089=VERTEX_POINT('',#275220);
#45090=VERTEX_POINT('',#275222);
#45091=VERTEX_POINT('',#275226);
#45092=VERTEX_POINT('',#275228);
#45093=VERTEX_POINT('',#275232);
#45094=VERTEX_POINT('',#275234);
#45095=VERTEX_POINT('',#275238);
#45096=VERTEX_POINT('',#275240);
#45097=VERTEX_POINT('',#275244);
#45098=VERTEX_POINT('',#275246);
#45099=VERTEX_POINT('',#275250);
#45100=VERTEX_POINT('',#275252);
#45101=VERTEX_POINT('',#275256);
#45102=VERTEX_POINT('',#275258);
#45103=VERTEX_POINT('',#275262);
#45104=VERTEX_POINT('',#275264);
#45105=VERTEX_POINT('',#275268);
#45106=VERTEX_POINT('',#275270);
#45107=VERTEX_POINT('',#275274);
#45108=VERTEX_POINT('',#275276);
#45109=VERTEX_POINT('',#275280);
#45110=VERTEX_POINT('',#275282);
#45111=VERTEX_POINT('',#275286);
#45112=VERTEX_POINT('',#275288);
#45113=VERTEX_POINT('',#275292);
#45114=VERTEX_POINT('',#275294);
#45115=VERTEX_POINT('',#275298);
#45116=VERTEX_POINT('',#275300);
#45117=VERTEX_POINT('',#275307);
#45118=VERTEX_POINT('',#275308);
#45119=VERTEX_POINT('',#275310);
#45120=VERTEX_POINT('',#275312);
#45121=VERTEX_POINT('',#275316);
#45122=VERTEX_POINT('',#275318);
#45123=VERTEX_POINT('',#275322);
#45124=VERTEX_POINT('',#275324);
#45125=VERTEX_POINT('',#275328);
#45126=VERTEX_POINT('',#275330);
#45127=VERTEX_POINT('',#275334);
#45128=VERTEX_POINT('',#275336);
#45129=VERTEX_POINT('',#275340);
#45130=VERTEX_POINT('',#275342);
#45131=VERTEX_POINT('',#275346);
#45132=VERTEX_POINT('',#275348);
#45133=VERTEX_POINT('',#275352);
#45134=VERTEX_POINT('',#275354);
#45135=VERTEX_POINT('',#275358);
#45136=VERTEX_POINT('',#275360);
#45137=VERTEX_POINT('',#275364);
#45138=VERTEX_POINT('',#275366);
#45139=VERTEX_POINT('',#275370);
#45140=VERTEX_POINT('',#275372);
#45141=VERTEX_POINT('',#275376);
#45142=VERTEX_POINT('',#275378);
#45143=VERTEX_POINT('',#275382);
#45144=VERTEX_POINT('',#275384);
#45145=VERTEX_POINT('',#275388);
#45146=VERTEX_POINT('',#275390);
#45147=VERTEX_POINT('',#275394);
#45148=VERTEX_POINT('',#275396);
#45149=VERTEX_POINT('',#275400);
#45150=VERTEX_POINT('',#275402);
#45151=VERTEX_POINT('',#275406);
#45152=VERTEX_POINT('',#275408);
#45153=VERTEX_POINT('',#275412);
#45154=VERTEX_POINT('',#275414);
#45155=VERTEX_POINT('',#275421);
#45156=VERTEX_POINT('',#275422);
#45157=VERTEX_POINT('',#275424);
#45158=VERTEX_POINT('',#275426);
#45159=VERTEX_POINT('',#275430);
#45160=VERTEX_POINT('',#275432);
#45161=VERTEX_POINT('',#275436);
#45162=VERTEX_POINT('',#275438);
#45163=VERTEX_POINT('',#275442);
#45164=VERTEX_POINT('',#275444);
#45165=VERTEX_POINT('',#275448);
#45166=VERTEX_POINT('',#275450);
#45167=VERTEX_POINT('',#275454);
#45168=VERTEX_POINT('',#275456);
#45169=VERTEX_POINT('',#275460);
#45170=VERTEX_POINT('',#275462);
#45171=VERTEX_POINT('',#275466);
#45172=VERTEX_POINT('',#275468);
#45173=VERTEX_POINT('',#275472);
#45174=VERTEX_POINT('',#275474);
#45175=VERTEX_POINT('',#275478);
#45176=VERTEX_POINT('',#275480);
#45177=VERTEX_POINT('',#275484);
#45178=VERTEX_POINT('',#275486);
#45179=VERTEX_POINT('',#275490);
#45180=VERTEX_POINT('',#275492);
#45181=VERTEX_POINT('',#275499);
#45182=VERTEX_POINT('',#275500);
#45183=VERTEX_POINT('',#275502);
#45184=VERTEX_POINT('',#275504);
#45185=VERTEX_POINT('',#275508);
#45186=VERTEX_POINT('',#275510);
#45187=VERTEX_POINT('',#275514);
#45188=VERTEX_POINT('',#275516);
#45189=VERTEX_POINT('',#275520);
#45190=VERTEX_POINT('',#275522);
#45191=VERTEX_POINT('',#275526);
#45192=VERTEX_POINT('',#275528);
#45193=VERTEX_POINT('',#275532);
#45194=VERTEX_POINT('',#275534);
#45195=VERTEX_POINT('',#275538);
#45196=VERTEX_POINT('',#275540);
#45197=VERTEX_POINT('',#275544);
#45198=VERTEX_POINT('',#275546);
#45199=VERTEX_POINT('',#275550);
#45200=VERTEX_POINT('',#275552);
#45201=VERTEX_POINT('',#275556);
#45202=VERTEX_POINT('',#275558);
#45203=VERTEX_POINT('',#275562);
#45204=VERTEX_POINT('',#275564);
#45205=VERTEX_POINT('',#275568);
#45206=VERTEX_POINT('',#275570);
#45207=VERTEX_POINT('',#275574);
#45208=VERTEX_POINT('',#275576);
#45209=VERTEX_POINT('',#275580);
#45210=VERTEX_POINT('',#275582);
#45211=VERTEX_POINT('',#275586);
#45212=VERTEX_POINT('',#275588);
#45213=VERTEX_POINT('',#275592);
#45214=VERTEX_POINT('',#275594);
#45215=VERTEX_POINT('',#275598);
#45216=VERTEX_POINT('',#275600);
#45217=VERTEX_POINT('',#275604);
#45218=VERTEX_POINT('',#275606);
#45219=VERTEX_POINT('',#275610);
#45220=VERTEX_POINT('',#275612);
#45221=VERTEX_POINT('',#275616);
#45222=VERTEX_POINT('',#275618);
#45223=VERTEX_POINT('',#275622);
#45224=VERTEX_POINT('',#275624);
#45225=VERTEX_POINT('',#275628);
#45226=VERTEX_POINT('',#275630);
#45227=VERTEX_POINT('',#275634);
#45228=VERTEX_POINT('',#275636);
#45229=VERTEX_POINT('',#275640);
#45230=VERTEX_POINT('',#275642);
#45231=VERTEX_POINT('',#275646);
#45232=VERTEX_POINT('',#275648);
#45233=VERTEX_POINT('',#275652);
#45234=VERTEX_POINT('',#275654);
#45235=VERTEX_POINT('',#275658);
#45236=VERTEX_POINT('',#275660);
#45237=VERTEX_POINT('',#275664);
#45238=VERTEX_POINT('',#275666);
#45239=VERTEX_POINT('',#275670);
#45240=VERTEX_POINT('',#275672);
#45241=VERTEX_POINT('',#275676);
#45242=VERTEX_POINT('',#275678);
#45243=VERTEX_POINT('',#275682);
#45244=VERTEX_POINT('',#275684);
#45245=VERTEX_POINT('',#275688);
#45246=VERTEX_POINT('',#275690);
#45247=VERTEX_POINT('',#275694);
#45248=VERTEX_POINT('',#275696);
#45249=VERTEX_POINT('',#275700);
#45250=VERTEX_POINT('',#275702);
#45251=VERTEX_POINT('',#275706);
#45252=VERTEX_POINT('',#275708);
#45253=VERTEX_POINT('',#275712);
#45254=VERTEX_POINT('',#275714);
#45255=VERTEX_POINT('',#275718);
#45256=VERTEX_POINT('',#275720);
#45257=VERTEX_POINT('',#275724);
#45258=VERTEX_POINT('',#275726);
#45259=VERTEX_POINT('',#275733);
#45260=VERTEX_POINT('',#275734);
#45261=VERTEX_POINT('',#275736);
#45262=VERTEX_POINT('',#275738);
#45263=VERTEX_POINT('',#275742);
#45264=VERTEX_POINT('',#275744);
#45265=VERTEX_POINT('',#275748);
#45266=VERTEX_POINT('',#275750);
#45267=VERTEX_POINT('',#275754);
#45268=VERTEX_POINT('',#275756);
#45269=VERTEX_POINT('',#275760);
#45270=VERTEX_POINT('',#275762);
#45271=VERTEX_POINT('',#275766);
#45272=VERTEX_POINT('',#275768);
#45273=VERTEX_POINT('',#275772);
#45274=VERTEX_POINT('',#275774);
#45275=VERTEX_POINT('',#275778);
#45276=VERTEX_POINT('',#275780);
#45277=VERTEX_POINT('',#275784);
#45278=VERTEX_POINT('',#275786);
#45279=VERTEX_POINT('',#275790);
#45280=VERTEX_POINT('',#275792);
#45281=VERTEX_POINT('',#275796);
#45282=VERTEX_POINT('',#275798);
#45283=VERTEX_POINT('',#275802);
#45284=VERTEX_POINT('',#275804);
#45285=VERTEX_POINT('',#275811);
#45286=VERTEX_POINT('',#275812);
#45287=VERTEX_POINT('',#275814);
#45288=VERTEX_POINT('',#275816);
#45289=VERTEX_POINT('',#275820);
#45290=VERTEX_POINT('',#275822);
#45291=VERTEX_POINT('',#275826);
#45292=VERTEX_POINT('',#275828);
#45293=VERTEX_POINT('',#275832);
#45294=VERTEX_POINT('',#275834);
#45295=VERTEX_POINT('',#275838);
#45296=VERTEX_POINT('',#275840);
#45297=VERTEX_POINT('',#275844);
#45298=VERTEX_POINT('',#275846);
#45299=VERTEX_POINT('',#275850);
#45300=VERTEX_POINT('',#275852);
#45301=VERTEX_POINT('',#275856);
#45302=VERTEX_POINT('',#275858);
#45303=VERTEX_POINT('',#275862);
#45304=VERTEX_POINT('',#275864);
#45305=VERTEX_POINT('',#275868);
#45306=VERTEX_POINT('',#275870);
#45307=VERTEX_POINT('',#275874);
#45308=VERTEX_POINT('',#275876);
#45309=VERTEX_POINT('',#275880);
#45310=VERTEX_POINT('',#275882);
#45311=VERTEX_POINT('',#275886);
#45312=VERTEX_POINT('',#275888);
#45313=VERTEX_POINT('',#275892);
#45314=VERTEX_POINT('',#275894);
#45315=VERTEX_POINT('',#275898);
#45316=VERTEX_POINT('',#275900);
#45317=VERTEX_POINT('',#275904);
#45318=VERTEX_POINT('',#275906);
#45319=VERTEX_POINT('',#275910);
#45320=VERTEX_POINT('',#275912);
#45321=VERTEX_POINT('',#275916);
#45322=VERTEX_POINT('',#275918);
#45323=VERTEX_POINT('',#275922);
#45324=VERTEX_POINT('',#275924);
#45325=VERTEX_POINT('',#275928);
#45326=VERTEX_POINT('',#275930);
#45327=VERTEX_POINT('',#275934);
#45328=VERTEX_POINT('',#275936);
#45329=VERTEX_POINT('',#275940);
#45330=VERTEX_POINT('',#275942);
#45331=VERTEX_POINT('',#275946);
#45332=VERTEX_POINT('',#275948);
#45333=VERTEX_POINT('',#275952);
#45334=VERTEX_POINT('',#275954);
#45335=VERTEX_POINT('',#275958);
#45336=VERTEX_POINT('',#275960);
#45337=VERTEX_POINT('',#275964);
#45338=VERTEX_POINT('',#275966);
#45339=VERTEX_POINT('',#275970);
#45340=VERTEX_POINT('',#275972);
#45341=VERTEX_POINT('',#275976);
#45342=VERTEX_POINT('',#275978);
#45343=VERTEX_POINT('',#275982);
#45344=VERTEX_POINT('',#275984);
#45345=VERTEX_POINT('',#275988);
#45346=VERTEX_POINT('',#275990);
#45347=VERTEX_POINT('',#275994);
#45348=VERTEX_POINT('',#275996);
#45349=VERTEX_POINT('',#276000);
#45350=VERTEX_POINT('',#276002);
#45351=VERTEX_POINT('',#276006);
#45352=VERTEX_POINT('',#276008);
#45353=VERTEX_POINT('',#276012);
#45354=VERTEX_POINT('',#276014);
#45355=VERTEX_POINT('',#276018);
#45356=VERTEX_POINT('',#276020);
#45357=VERTEX_POINT('',#276024);
#45358=VERTEX_POINT('',#276026);
#45359=VERTEX_POINT('',#276030);
#45360=VERTEX_POINT('',#276032);
#45361=VERTEX_POINT('',#276036);
#45362=VERTEX_POINT('',#276038);
#45363=VERTEX_POINT('',#276045);
#45364=VERTEX_POINT('',#276046);
#45365=VERTEX_POINT('',#276048);
#45366=VERTEX_POINT('',#276050);
#45367=VERTEX_POINT('',#276054);
#45368=VERTEX_POINT('',#276056);
#45369=VERTEX_POINT('',#276060);
#45370=VERTEX_POINT('',#276062);
#45371=VERTEX_POINT('',#276066);
#45372=VERTEX_POINT('',#276068);
#45373=VERTEX_POINT('',#276072);
#45374=VERTEX_POINT('',#276074);
#45375=VERTEX_POINT('',#276078);
#45376=VERTEX_POINT('',#276080);
#45377=VERTEX_POINT('',#276084);
#45378=VERTEX_POINT('',#276086);
#45379=VERTEX_POINT('',#276090);
#45380=VERTEX_POINT('',#276092);
#45381=VERTEX_POINT('',#276096);
#45382=VERTEX_POINT('',#276098);
#45383=VERTEX_POINT('',#276102);
#45384=VERTEX_POINT('',#276104);
#45385=VERTEX_POINT('',#276108);
#45386=VERTEX_POINT('',#276110);
#45387=VERTEX_POINT('',#276114);
#45388=VERTEX_POINT('',#276116);
#45389=VERTEX_POINT('',#276123);
#45390=VERTEX_POINT('',#276125);
#45391=VERTEX_POINT('',#276129);
#45392=VERTEX_POINT('',#276131);
#45393=VERTEX_POINT('',#276135);
#45394=VERTEX_POINT('',#276137);
#45395=VERTEX_POINT('',#276141);
#45396=VERTEX_POINT('',#276143);
#45397=VERTEX_POINT('',#276147);
#45398=VERTEX_POINT('',#276149);
#45399=VERTEX_POINT('',#276153);
#45400=VERTEX_POINT('',#276155);
#45401=VERTEX_POINT('',#276159);
#45402=VERTEX_POINT('',#276161);
#45403=VERTEX_POINT('',#276165);
#45404=VERTEX_POINT('',#276167);
#45405=VERTEX_POINT('',#276171);
#45406=VERTEX_POINT('',#276173);
#45407=VERTEX_POINT('',#276177);
#45408=VERTEX_POINT('',#276179);
#45409=VERTEX_POINT('',#276183);
#45410=VERTEX_POINT('',#276185);
#45411=VERTEX_POINT('',#276189);
#45412=VERTEX_POINT('',#276191);
#45413=VERTEX_POINT('',#276195);
#45414=VERTEX_POINT('',#276197);
#45415=VERTEX_POINT('',#276201);
#45416=VERTEX_POINT('',#276203);
#45417=VERTEX_POINT('',#276207);
#45418=VERTEX_POINT('',#276209);
#45419=VERTEX_POINT('',#276213);
#45420=VERTEX_POINT('',#276215);
#45421=VERTEX_POINT('',#276219);
#45422=VERTEX_POINT('',#276221);
#45423=VERTEX_POINT('',#276225);
#45424=VERTEX_POINT('',#276227);
#45425=VERTEX_POINT('',#276231);
#45426=VERTEX_POINT('',#276233);
#45427=VERTEX_POINT('',#276237);
#45428=VERTEX_POINT('',#276239);
#45429=VERTEX_POINT('',#276243);
#45430=VERTEX_POINT('',#276245);
#45431=VERTEX_POINT('',#276249);
#45432=VERTEX_POINT('',#276251);
#45433=VERTEX_POINT('',#276255);
#45434=VERTEX_POINT('',#276257);
#45435=VERTEX_POINT('',#276261);
#45436=VERTEX_POINT('',#276263);
#45437=VERTEX_POINT('',#276267);
#45438=VERTEX_POINT('',#276269);
#45439=VERTEX_POINT('',#276273);
#45440=VERTEX_POINT('',#276275);
#45441=VERTEX_POINT('',#276279);
#45442=VERTEX_POINT('',#276281);
#45443=VERTEX_POINT('',#276285);
#45444=VERTEX_POINT('',#276287);
#45445=VERTEX_POINT('',#276291);
#45446=VERTEX_POINT('',#276293);
#45447=VERTEX_POINT('',#276297);
#45448=VERTEX_POINT('',#276299);
#45449=VERTEX_POINT('',#276303);
#45450=VERTEX_POINT('',#276305);
#45451=VERTEX_POINT('',#276309);
#45452=VERTEX_POINT('',#276311);
#45453=VERTEX_POINT('',#276315);
#45454=VERTEX_POINT('',#276317);
#45455=VERTEX_POINT('',#276321);
#45456=VERTEX_POINT('',#276323);
#45457=VERTEX_POINT('',#276327);
#45458=VERTEX_POINT('',#276329);
#45459=VERTEX_POINT('',#276333);
#45460=VERTEX_POINT('',#276335);
#45461=VERTEX_POINT('',#276339);
#45462=VERTEX_POINT('',#276341);
#45463=VERTEX_POINT('',#276348);
#45464=VERTEX_POINT('',#276350);
#45465=VERTEX_POINT('',#276357);
#45466=VERTEX_POINT('',#276359);
#45467=VERTEX_POINT('',#276366);
#45468=VERTEX_POINT('',#276367);
#45469=VERTEX_POINT('',#276369);
#45470=VERTEX_POINT('',#276371);
#45471=VERTEX_POINT('',#276373);
#45472=VERTEX_POINT('',#276375);
#45473=VERTEX_POINT('',#276377);
#45474=VERTEX_POINT('',#276379);
#45475=VERTEX_POINT('',#276383);
#45476=VERTEX_POINT('',#276384);
#45477=VERTEX_POINT('',#276389);
#45478=VERTEX_POINT('',#276393);
#45479=VERTEX_POINT('',#276397);
#45480=VERTEX_POINT('',#276401);
#45481=VERTEX_POINT('',#276405);
#45482=VERTEX_POINT('',#276409);
#45483=VERTEX_POINT('',#276416);
#45484=VERTEX_POINT('',#276417);
#45485=VERTEX_POINT('',#276419);
#45486=VERTEX_POINT('',#276421);
#45487=VERTEX_POINT('',#276425);
#45488=VERTEX_POINT('',#276427);
#45489=VERTEX_POINT('',#276431);
#45490=VERTEX_POINT('',#276433);
#59291=EDGE_CURVE('',#44735,#44736,#36279,.T.);
#59292=EDGE_CURVE('',#44736,#44737,#24331,.T.);
#59293=EDGE_CURVE('',#44738,#44737,#36280,.T.);
#59294=EDGE_CURVE('',#44735,#44738,#24332,.T.);
#59295=EDGE_CURVE('',#44739,#44740,#36281,.T.);
#59296=EDGE_CURVE('',#44740,#44741,#24333,.T.);
#59297=EDGE_CURVE('',#44741,#44742,#36282,.T.);
#59298=EDGE_CURVE('',#44742,#44743,#24334,.T.);
#59299=EDGE_CURVE('',#44743,#44744,#36283,.T.);
#59300=EDGE_CURVE('',#44744,#44745,#24335,.T.);
#59301=EDGE_CURVE('',#44745,#44746,#36284,.T.);
#59302=EDGE_CURVE('',#44746,#44747,#24336,.T.);
#59303=EDGE_CURVE('',#44747,#44748,#36285,.T.);
#59304=EDGE_CURVE('',#44748,#44749,#24337,.T.);
#59305=EDGE_CURVE('',#44749,#44750,#36286,.T.);
#59306=EDGE_CURVE('',#44750,#44751,#24338,.T.);
#59307=EDGE_CURVE('',#44751,#44752,#36287,.T.);
#59308=EDGE_CURVE('',#44752,#44738,#24339,.T.);
#59309=EDGE_CURVE('',#44737,#44739,#24340,.T.);
#59310=EDGE_CURVE('',#44736,#44753,#24341,.T.);
#59311=EDGE_CURVE('',#44753,#44739,#24342,.T.);
#59312=EDGE_CURVE('',#44754,#44752,#24343,.T.);
#59313=EDGE_CURVE('',#44754,#44735,#24344,.T.);
#59314=EDGE_CURVE('',#44755,#44751,#24345,.T.);
#59315=EDGE_CURVE('',#44755,#44754,#36288,.T.);
#59316=EDGE_CURVE('',#44756,#44750,#24346,.T.);
#59317=EDGE_CURVE('',#44756,#44755,#24347,.T.);
#59318=EDGE_CURVE('',#44757,#44749,#24348,.T.);
#59319=EDGE_CURVE('',#44757,#44756,#36289,.T.);
#59320=EDGE_CURVE('',#44758,#44748,#24349,.T.);
#59321=EDGE_CURVE('',#44758,#44757,#24350,.T.);
#59322=EDGE_CURVE('',#44759,#44747,#24351,.T.);
#59323=EDGE_CURVE('',#44759,#44758,#36290,.T.);
#59324=EDGE_CURVE('',#44760,#44746,#24352,.T.);
#59325=EDGE_CURVE('',#44760,#44759,#24353,.T.);
#59326=EDGE_CURVE('',#44761,#44745,#24354,.T.);
#59327=EDGE_CURVE('',#44761,#44760,#36291,.T.);
#59328=EDGE_CURVE('',#44762,#44744,#24355,.T.);
#59329=EDGE_CURVE('',#44762,#44761,#24356,.T.);
#59330=EDGE_CURVE('',#44763,#44743,#24357,.T.);
#59331=EDGE_CURVE('',#44763,#44762,#36292,.T.);
#59332=EDGE_CURVE('',#44764,#44742,#24358,.T.);
#59333=EDGE_CURVE('',#44764,#44763,#24359,.T.);
#59334=EDGE_CURVE('',#44765,#44741,#24360,.T.);
#59335=EDGE_CURVE('',#44765,#44764,#36293,.T.);
#59336=EDGE_CURVE('',#44766,#44740,#24361,.T.);
#59337=EDGE_CURVE('',#44766,#44765,#24362,.T.);
#59338=EDGE_CURVE('',#44753,#44766,#36294,.T.);
#59339=EDGE_CURVE('',#44767,#44768,#36295,.T.);
#59340=EDGE_CURVE('',#44768,#44769,#24363,.T.);
#59341=EDGE_CURVE('',#44769,#44770,#36296,.T.);
#59342=EDGE_CURVE('',#44770,#44771,#24364,.T.);
#59343=EDGE_CURVE('',#44771,#44772,#36297,.T.);
#59344=EDGE_CURVE('',#44772,#44773,#24365,.T.);
#59345=EDGE_CURVE('',#44773,#44774,#36298,.T.);
#59346=EDGE_CURVE('',#44774,#44767,#24366,.T.);
#59347=EDGE_CURVE('',#44775,#44774,#24367,.T.);
#59348=EDGE_CURVE('',#44775,#44776,#24368,.T.);
#59349=EDGE_CURVE('',#44776,#44767,#24369,.T.);
#59350=EDGE_CURVE('',#44777,#44773,#24370,.T.);
#59351=EDGE_CURVE('',#44777,#44775,#36299,.T.);
#59352=EDGE_CURVE('',#44778,#44772,#24371,.T.);
#59353=EDGE_CURVE('',#44778,#44777,#24372,.T.);
#59354=EDGE_CURVE('',#44779,#44771,#24373,.T.);
#59355=EDGE_CURVE('',#44779,#44778,#36300,.T.);
#59356=EDGE_CURVE('',#44780,#44770,#24374,.T.);
#59357=EDGE_CURVE('',#44780,#44779,#24375,.T.);
#59358=EDGE_CURVE('',#44781,#44769,#24376,.T.);
#59359=EDGE_CURVE('',#44781,#44780,#36301,.T.);
#59360=EDGE_CURVE('',#44782,#44768,#24377,.T.);
#59361=EDGE_CURVE('',#44782,#44781,#24378,.T.);
#59362=EDGE_CURVE('',#44776,#44782,#36302,.T.);
#59363=EDGE_CURVE('',#44783,#44784,#36303,.T.);
#59364=EDGE_CURVE('',#44784,#44785,#24379,.T.);
#59365=EDGE_CURVE('',#44785,#44786,#36304,.T.);
#59366=EDGE_CURVE('',#44786,#44787,#24380,.T.);
#59367=EDGE_CURVE('',#44787,#44788,#36305,.T.);
#59368=EDGE_CURVE('',#44788,#44789,#24381,.T.);
#59369=EDGE_CURVE('',#44789,#44790,#36306,.T.);
#59370=EDGE_CURVE('',#44790,#44791,#24382,.T.);
#59371=EDGE_CURVE('',#44791,#44792,#24383,.T.);
#59372=EDGE_CURVE('',#44792,#44793,#24384,.T.);
#59373=EDGE_CURVE('',#44793,#44794,#36307,.T.);
#59374=EDGE_CURVE('',#44794,#44795,#24385,.T.);
#59375=EDGE_CURVE('',#44795,#44796,#36308,.T.);
#59376=EDGE_CURVE('',#44796,#44797,#24386,.T.);
#59377=EDGE_CURVE('',#44797,#44798,#36309,.T.);
#59378=EDGE_CURVE('',#44798,#44799,#24387,.T.);
#59379=EDGE_CURVE('',#44799,#44800,#36310,.T.);
#59380=EDGE_CURVE('',#44800,#44801,#24388,.T.);
#59381=EDGE_CURVE('',#44801,#44802,#36311,.T.);
#59382=EDGE_CURVE('',#44802,#44803,#24389,.T.);
#59383=EDGE_CURVE('',#44803,#44804,#36312,.T.);
#59384=EDGE_CURVE('',#44804,#44805,#24390,.T.);
#59385=EDGE_CURVE('',#44805,#44806,#24391,.T.);
#59386=EDGE_CURVE('',#44806,#44807,#24392,.T.);
#59387=EDGE_CURVE('',#44807,#44808,#36313,.T.);
#59388=EDGE_CURVE('',#44808,#44809,#24393,.T.);
#59389=EDGE_CURVE('',#44809,#44810,#36314,.T.);
#59390=EDGE_CURVE('',#44810,#44811,#24394,.T.);
#59391=EDGE_CURVE('',#44811,#44812,#36315,.T.);
#59392=EDGE_CURVE('',#44812,#44813,#24395,.T.);
#59393=EDGE_CURVE('',#44813,#44814,#36316,.T.);
#59394=EDGE_CURVE('',#44814,#44815,#24396,.T.);
#59395=EDGE_CURVE('',#44815,#44816,#36317,.T.);
#59396=EDGE_CURVE('',#44816,#44817,#24397,.T.);
#59397=EDGE_CURVE('',#44817,#44818,#36318,.T.);
#59398=EDGE_CURVE('',#44818,#44819,#24398,.T.);
#59399=EDGE_CURVE('',#44819,#44820,#24399,.T.);
#59400=EDGE_CURVE('',#44820,#44821,#24400,.T.);
#59401=EDGE_CURVE('',#44821,#44822,#36319,.T.);
#59402=EDGE_CURVE('',#44822,#44823,#24401,.T.);
#59403=EDGE_CURVE('',#44823,#44824,#36320,.T.);
#59404=EDGE_CURVE('',#44824,#44825,#24402,.T.);
#59405=EDGE_CURVE('',#44825,#44826,#36321,.T.);
#59406=EDGE_CURVE('',#44826,#44827,#24403,.T.);
#59407=EDGE_CURVE('',#44827,#44828,#36322,.T.);
#59408=EDGE_CURVE('',#44828,#44829,#24404,.T.);
#59409=EDGE_CURVE('',#44829,#44830,#36323,.T.);
#59410=EDGE_CURVE('',#44830,#44831,#24405,.T.);
#59411=EDGE_CURVE('',#44831,#44832,#36324,.T.);
#59412=EDGE_CURVE('',#44832,#44833,#24406,.T.);
#59413=EDGE_CURVE('',#44833,#44834,#24407,.T.);
#59414=EDGE_CURVE('',#44834,#44835,#24408,.T.);
#59415=EDGE_CURVE('',#44835,#44836,#36325,.T.);
#59416=EDGE_CURVE('',#44836,#44837,#24409,.T.);
#59417=EDGE_CURVE('',#44837,#44838,#36326,.T.);
#59418=EDGE_CURVE('',#44838,#44783,#24410,.T.);
#59419=EDGE_CURVE('',#44839,#44840,#36327,.T.);
#59420=EDGE_CURVE('',#44841,#44839,#24411,.T.);
#59421=EDGE_CURVE('',#44842,#44841,#36328,.T.);
#59422=EDGE_CURVE('',#44843,#44842,#24412,.T.);
#59423=EDGE_CURVE('',#44844,#44843,#36329,.T.);
#59424=EDGE_CURVE('',#44845,#44844,#24413,.T.);
#59425=EDGE_CURVE('',#44846,#44845,#36330,.T.);
#59426=EDGE_CURVE('',#44847,#44846,#24414,.T.);
#59427=EDGE_CURVE('',#44848,#44847,#24415,.T.);
#59428=EDGE_CURVE('',#44849,#44848,#24416,.T.);
#59429=EDGE_CURVE('',#44850,#44849,#36331,.T.);
#59430=EDGE_CURVE('',#44851,#44850,#24417,.T.);
#59431=EDGE_CURVE('',#44852,#44851,#36332,.T.);
#59432=EDGE_CURVE('',#44853,#44852,#24418,.T.);
#59433=EDGE_CURVE('',#44854,#44853,#36333,.T.);
#59434=EDGE_CURVE('',#44855,#44854,#24419,.T.);
#59435=EDGE_CURVE('',#44856,#44855,#36334,.T.);
#59436=EDGE_CURVE('',#44857,#44856,#24420,.T.);
#59437=EDGE_CURVE('',#44858,#44857,#36335,.T.);
#59438=EDGE_CURVE('',#44859,#44858,#24421,.T.);
#59439=EDGE_CURVE('',#44860,#44859,#36336,.T.);
#59440=EDGE_CURVE('',#44861,#44860,#24422,.T.);
#59441=EDGE_CURVE('',#44862,#44861,#24423,.T.);
#59442=EDGE_CURVE('',#44863,#44862,#24424,.T.);
#59443=EDGE_CURVE('',#44864,#44863,#36337,.T.);
#59444=EDGE_CURVE('',#44865,#44864,#24425,.T.);
#59445=EDGE_CURVE('',#44866,#44865,#36338,.T.);
#59446=EDGE_CURVE('',#44867,#44866,#24426,.T.);
#59447=EDGE_CURVE('',#44868,#44867,#36339,.T.);
#59448=EDGE_CURVE('',#44869,#44868,#24427,.T.);
#59449=EDGE_CURVE('',#44870,#44869,#36340,.T.);
#59450=EDGE_CURVE('',#44871,#44870,#24428,.T.);
#59451=EDGE_CURVE('',#44872,#44871,#36341,.T.);
#59452=EDGE_CURVE('',#44873,#44872,#24429,.T.);
#59453=EDGE_CURVE('',#44874,#44873,#36342,.T.);
#59454=EDGE_CURVE('',#44875,#44874,#24430,.T.);
#59455=EDGE_CURVE('',#44876,#44875,#24431,.T.);
#59456=EDGE_CURVE('',#44877,#44876,#24432,.T.);
#59457=EDGE_CURVE('',#44878,#44877,#36343,.T.);
#59458=EDGE_CURVE('',#44879,#44878,#24433,.T.);
#59459=EDGE_CURVE('',#44880,#44879,#36344,.T.);
#59460=EDGE_CURVE('',#44881,#44880,#24434,.T.);
#59461=EDGE_CURVE('',#44882,#44881,#36345,.T.);
#59462=EDGE_CURVE('',#44883,#44882,#24435,.T.);
#59463=EDGE_CURVE('',#44884,#44883,#36346,.T.);
#59464=EDGE_CURVE('',#44885,#44884,#24436,.T.);
#59465=EDGE_CURVE('',#44886,#44885,#36347,.T.);
#59466=EDGE_CURVE('',#44887,#44886,#24437,.T.);
#59467=EDGE_CURVE('',#44888,#44887,#36348,.T.);
#59468=EDGE_CURVE('',#44889,#44888,#24438,.T.);
#59469=EDGE_CURVE('',#44890,#44889,#24439,.T.);
#59470=EDGE_CURVE('',#44891,#44890,#24440,.T.);
#59471=EDGE_CURVE('',#44892,#44891,#36349,.T.);
#59472=EDGE_CURVE('',#44893,#44892,#24441,.T.);
#59473=EDGE_CURVE('',#44894,#44893,#36350,.T.);
#59474=EDGE_CURVE('',#44840,#44894,#24442,.T.);
#59475=EDGE_CURVE('',#44783,#44842,#24443,.T.);
#59476=EDGE_CURVE('',#44784,#44841,#24444,.T.);
#59477=EDGE_CURVE('',#44838,#44843,#24445,.T.);
#59478=EDGE_CURVE('',#44837,#44844,#24446,.T.);
#59479=EDGE_CURVE('',#44836,#44845,#24447,.T.);
#59480=EDGE_CURVE('',#44835,#44846,#24448,.T.);
#59481=EDGE_CURVE('',#44834,#44847,#24449,.T.);
#59482=EDGE_CURVE('',#44833,#44848,#24450,.T.);
#59483=EDGE_CURVE('',#44832,#44849,#24451,.T.);
#59484=EDGE_CURVE('',#44831,#44850,#24452,.T.);
#59485=EDGE_CURVE('',#44830,#44851,#24453,.T.);
#59486=EDGE_CURVE('',#44829,#44852,#24454,.T.);
#59487=EDGE_CURVE('',#44828,#44853,#24455,.T.);
#59488=EDGE_CURVE('',#44827,#44854,#24456,.T.);
#59489=EDGE_CURVE('',#44826,#44855,#24457,.T.);
#59490=EDGE_CURVE('',#44825,#44856,#24458,.T.);
#59491=EDGE_CURVE('',#44824,#44857,#24459,.T.);
#59492=EDGE_CURVE('',#44823,#44858,#24460,.T.);
#59493=EDGE_CURVE('',#44822,#44859,#24461,.T.);
#59494=EDGE_CURVE('',#44821,#44860,#24462,.T.);
#59495=EDGE_CURVE('',#44820,#44861,#24463,.T.);
#59496=EDGE_CURVE('',#44819,#44862,#24464,.T.);
#59497=EDGE_CURVE('',#44818,#44863,#24465,.T.);
#59498=EDGE_CURVE('',#44817,#44864,#24466,.T.);
#59499=EDGE_CURVE('',#44816,#44865,#24467,.T.);
#59500=EDGE_CURVE('',#44815,#44866,#24468,.T.);
#59501=EDGE_CURVE('',#44814,#44867,#24469,.T.);
#59502=EDGE_CURVE('',#44813,#44868,#24470,.T.);
#59503=EDGE_CURVE('',#44812,#44869,#24471,.T.);
#59504=EDGE_CURVE('',#44811,#44870,#24472,.T.);
#59505=EDGE_CURVE('',#44810,#44871,#24473,.T.);
#59506=EDGE_CURVE('',#44809,#44872,#24474,.T.);
#59507=EDGE_CURVE('',#44808,#44873,#24475,.T.);
#59508=EDGE_CURVE('',#44807,#44874,#24476,.T.);
#59509=EDGE_CURVE('',#44806,#44875,#24477,.T.);
#59510=EDGE_CURVE('',#44805,#44876,#24478,.T.);
#59511=EDGE_CURVE('',#44804,#44877,#24479,.T.);
#59512=EDGE_CURVE('',#44803,#44878,#24480,.T.);
#59513=EDGE_CURVE('',#44802,#44879,#24481,.T.);
#59514=EDGE_CURVE('',#44801,#44880,#24482,.T.);
#59515=EDGE_CURVE('',#44800,#44881,#24483,.T.);
#59516=EDGE_CURVE('',#44799,#44882,#24484,.T.);
#59517=EDGE_CURVE('',#44798,#44883,#24485,.T.);
#59518=EDGE_CURVE('',#44797,#44884,#24486,.T.);
#59519=EDGE_CURVE('',#44796,#44885,#24487,.T.);
#59520=EDGE_CURVE('',#44795,#44886,#24488,.T.);
#59521=EDGE_CURVE('',#44794,#44887,#24489,.T.);
#59522=EDGE_CURVE('',#44793,#44888,#24490,.T.);
#59523=EDGE_CURVE('',#44792,#44889,#24491,.T.);
#59524=EDGE_CURVE('',#44791,#44890,#24492,.T.);
#59525=EDGE_CURVE('',#44790,#44891,#24493,.T.);
#59526=EDGE_CURVE('',#44789,#44892,#24494,.T.);
#59527=EDGE_CURVE('',#44788,#44893,#24495,.T.);
#59528=EDGE_CURVE('',#44787,#44894,#24496,.T.);
#59529=EDGE_CURVE('',#44786,#44840,#24497,.T.);
#59530=EDGE_CURVE('',#44785,#44839,#24498,.T.);
#59531=EDGE_CURVE('',#44895,#44896,#36351,.T.);
#59532=EDGE_CURVE('',#44896,#44897,#24499,.T.);
#59533=EDGE_CURVE('',#44898,#44897,#36352,.T.);
#59534=EDGE_CURVE('',#44895,#44898,#24500,.T.);
#59535=EDGE_CURVE('',#44899,#44900,#36353,.T.);
#59536=EDGE_CURVE('',#44900,#44901,#24501,.T.);
#59537=EDGE_CURVE('',#44901,#44902,#36354,.T.);
#59538=EDGE_CURVE('',#44902,#44903,#24502,.T.);
#59539=EDGE_CURVE('',#44903,#44904,#36355,.T.);
#59540=EDGE_CURVE('',#44904,#44898,#24503,.T.);
#59541=EDGE_CURVE('',#44897,#44905,#24504,.T.);
#59542=EDGE_CURVE('',#44905,#44906,#36356,.T.);
#59543=EDGE_CURVE('',#44906,#44907,#24505,.T.);
#59544=EDGE_CURVE('',#44907,#44908,#36357,.T.);
#59545=EDGE_CURVE('',#44908,#44909,#24506,.T.);
#59546=EDGE_CURVE('',#44909,#44910,#36358,.T.);
#59547=EDGE_CURVE('',#44910,#44911,#24507,.T.);
#59548=EDGE_CURVE('',#44911,#44912,#36359,.T.);
#59549=EDGE_CURVE('',#44912,#44899,#24508,.T.);
#59550=EDGE_CURVE('',#44913,#44912,#24509,.T.);
#59551=EDGE_CURVE('',#44913,#44914,#24510,.T.);
#59552=EDGE_CURVE('',#44914,#44899,#24511,.T.);
#59553=EDGE_CURVE('',#44915,#44911,#24512,.T.);
#59554=EDGE_CURVE('',#44915,#44913,#36360,.T.);
#59555=EDGE_CURVE('',#44916,#44910,#24513,.T.);
#59556=EDGE_CURVE('',#44916,#44915,#24514,.T.);
#59557=EDGE_CURVE('',#44917,#44909,#24515,.T.);
#59558=EDGE_CURVE('',#44917,#44916,#36361,.T.);
#59559=EDGE_CURVE('',#44918,#44908,#24516,.T.);
#59560=EDGE_CURVE('',#44918,#44917,#24517,.T.);
#59561=EDGE_CURVE('',#44919,#44907,#24518,.T.);
#59562=EDGE_CURVE('',#44919,#44918,#36362,.T.);
#59563=EDGE_CURVE('',#44920,#44906,#24519,.T.);
#59564=EDGE_CURVE('',#44920,#44919,#24520,.T.);
#59565=EDGE_CURVE('',#44921,#44905,#24521,.T.);
#59566=EDGE_CURVE('',#44921,#44920,#36363,.T.);
#59567=EDGE_CURVE('',#44896,#44921,#24522,.T.);
#59568=EDGE_CURVE('',#44922,#44904,#24523,.T.);
#59569=EDGE_CURVE('',#44922,#44895,#24524,.T.);
#59570=EDGE_CURVE('',#44923,#44903,#24525,.T.);
#59571=EDGE_CURVE('',#44923,#44922,#36364,.T.);
#59572=EDGE_CURVE('',#44924,#44902,#24526,.T.);
#59573=EDGE_CURVE('',#44924,#44923,#24527,.T.);
#59574=EDGE_CURVE('',#44925,#44901,#24528,.T.);
#59575=EDGE_CURVE('',#44925,#44924,#36365,.T.);
#59576=EDGE_CURVE('',#44926,#44900,#24529,.T.);
#59577=EDGE_CURVE('',#44926,#44925,#24530,.T.);
#59578=EDGE_CURVE('',#44914,#44926,#36366,.T.);
#59579=EDGE_CURVE('',#44927,#44928,#36367,.T.);
#59580=EDGE_CURVE('',#44928,#44929,#24531,.T.);
#59581=EDGE_CURVE('',#44929,#44930,#36368,.T.);
#59582=EDGE_CURVE('',#44930,#44931,#24532,.T.);
#59583=EDGE_CURVE('',#44931,#44932,#36369,.T.);
#59584=EDGE_CURVE('',#44932,#44933,#24533,.T.);
#59585=EDGE_CURVE('',#44933,#44934,#36370,.T.);
#59586=EDGE_CURVE('',#44934,#44927,#24534,.T.);
#59587=EDGE_CURVE('',#44935,#44934,#24535,.T.);
#59588=EDGE_CURVE('',#44935,#44936,#24536,.T.);
#59589=EDGE_CURVE('',#44936,#44927,#24537,.T.);
#59590=EDGE_CURVE('',#44937,#44933,#24538,.T.);
#59591=EDGE_CURVE('',#44937,#44935,#36371,.T.);
#59592=EDGE_CURVE('',#44938,#44932,#24539,.T.);
#59593=EDGE_CURVE('',#44938,#44937,#24540,.T.);
#59594=EDGE_CURVE('',#44939,#44931,#24541,.T.);
#59595=EDGE_CURVE('',#44939,#44938,#36372,.T.);
#59596=EDGE_CURVE('',#44940,#44930,#24542,.T.);
#59597=EDGE_CURVE('',#44940,#44939,#24543,.T.);
#59598=EDGE_CURVE('',#44941,#44929,#24544,.T.);
#59599=EDGE_CURVE('',#44941,#44940,#36373,.T.);
#59600=EDGE_CURVE('',#44942,#44928,#24545,.T.);
#59601=EDGE_CURVE('',#44942,#44941,#24546,.T.);
#59602=EDGE_CURVE('',#44936,#44942,#36374,.T.);
#59603=EDGE_CURVE('',#44943,#44944,#36375,.T.);
#59604=EDGE_CURVE('',#44944,#44945,#24547,.T.);
#59605=EDGE_CURVE('',#44946,#44945,#36376,.T.);
#59606=EDGE_CURVE('',#44943,#44946,#24548,.T.);
#59607=EDGE_CURVE('',#44947,#44948,#36377,.T.);
#59608=EDGE_CURVE('',#44948,#44946,#24549,.T.);
#59609=EDGE_CURVE('',#44945,#44949,#24550,.T.);
#59610=EDGE_CURVE('',#44949,#44950,#36378,.T.);
#59611=EDGE_CURVE('',#44950,#44951,#24551,.T.);
#59612=EDGE_CURVE('',#44951,#44952,#36379,.T.);
#59613=EDGE_CURVE('',#44952,#44953,#24552,.T.);
#59614=EDGE_CURVE('',#44953,#44954,#36380,.T.);
#59615=EDGE_CURVE('',#44954,#44955,#24553,.T.);
#59616=EDGE_CURVE('',#44955,#44956,#36381,.T.);
#59617=EDGE_CURVE('',#44956,#44957,#24554,.T.);
#59618=EDGE_CURVE('',#44957,#44958,#36382,.T.);
#59619=EDGE_CURVE('',#44958,#44959,#24555,.T.);
#59620=EDGE_CURVE('',#44959,#44960,#36383,.T.);
#59621=EDGE_CURVE('',#44960,#44947,#24556,.T.);
#59622=EDGE_CURVE('',#44961,#44960,#24557,.T.);
#59623=EDGE_CURVE('',#44961,#44962,#24558,.T.);
#59624=EDGE_CURVE('',#44962,#44947,#24559,.T.);
#59625=EDGE_CURVE('',#44963,#44959,#24560,.T.);
#59626=EDGE_CURVE('',#44963,#44961,#36384,.T.);
#59627=EDGE_CURVE('',#44964,#44958,#24561,.T.);
#59628=EDGE_CURVE('',#44964,#44963,#24562,.T.);
#59629=EDGE_CURVE('',#44965,#44957,#24563,.T.);
#59630=EDGE_CURVE('',#44965,#44964,#36385,.T.);
#59631=EDGE_CURVE('',#44966,#44956,#24564,.T.);
#59632=EDGE_CURVE('',#44966,#44965,#24565,.T.);
#59633=EDGE_CURVE('',#44967,#44955,#24566,.T.);
#59634=EDGE_CURVE('',#44967,#44966,#36386,.T.);
#59635=EDGE_CURVE('',#44968,#44954,#24567,.T.);
#59636=EDGE_CURVE('',#44968,#44967,#24568,.T.);
#59637=EDGE_CURVE('',#44969,#44953,#24569,.T.);
#59638=EDGE_CURVE('',#44969,#44968,#36387,.T.);
#59639=EDGE_CURVE('',#44970,#44952,#24570,.T.);
#59640=EDGE_CURVE('',#44970,#44969,#24571,.T.);
#59641=EDGE_CURVE('',#44971,#44951,#24572,.T.);
#59642=EDGE_CURVE('',#44971,#44970,#36388,.T.);
#59643=EDGE_CURVE('',#44972,#44950,#24573,.T.);
#59644=EDGE_CURVE('',#44972,#44971,#24574,.T.);
#59645=EDGE_CURVE('',#44973,#44949,#24575,.T.);
#59646=EDGE_CURVE('',#44973,#44972,#36389,.T.);
#59647=EDGE_CURVE('',#44944,#44973,#24576,.T.);
#59648=EDGE_CURVE('',#44974,#44948,#24577,.T.);
#59649=EDGE_CURVE('',#44974,#44943,#24578,.T.);
#59650=EDGE_CURVE('',#44962,#44974,#36390,.T.);
#59651=EDGE_CURVE('',#44975,#44976,#36391,.T.);
#59652=EDGE_CURVE('',#44976,#44977,#24579,.T.);
#59653=EDGE_CURVE('',#44977,#44978,#36392,.T.);
#59654=EDGE_CURVE('',#44978,#44979,#24580,.T.);
#59655=EDGE_CURVE('',#44979,#44980,#36393,.T.);
#59656=EDGE_CURVE('',#44980,#44981,#24581,.T.);
#59657=EDGE_CURVE('',#44981,#44982,#36394,.T.);
#59658=EDGE_CURVE('',#44982,#44975,#24582,.T.);
#59659=EDGE_CURVE('',#44983,#44982,#24583,.T.);
#59660=EDGE_CURVE('',#44983,#44984,#24584,.T.);
#59661=EDGE_CURVE('',#44984,#44975,#24585,.T.);
#59662=EDGE_CURVE('',#44985,#44981,#24586,.T.);
#59663=EDGE_CURVE('',#44985,#44983,#36395,.T.);
#59664=EDGE_CURVE('',#44986,#44980,#24587,.T.);
#59665=EDGE_CURVE('',#44986,#44985,#24588,.T.);
#59666=EDGE_CURVE('',#44987,#44979,#24589,.T.);
#59667=EDGE_CURVE('',#44987,#44986,#36396,.T.);
#59668=EDGE_CURVE('',#44988,#44978,#24590,.T.);
#59669=EDGE_CURVE('',#44988,#44987,#24591,.T.);
#59670=EDGE_CURVE('',#44989,#44977,#24592,.T.);
#59671=EDGE_CURVE('',#44989,#44988,#36397,.T.);
#59672=EDGE_CURVE('',#44990,#44976,#24593,.T.);
#59673=EDGE_CURVE('',#44990,#44989,#24594,.T.);
#59674=EDGE_CURVE('',#44984,#44990,#36398,.T.);
#59675=EDGE_CURVE('',#44991,#44992,#36399,.T.);
#59676=EDGE_CURVE('',#44992,#44993,#24595,.T.);
#59677=EDGE_CURVE('',#44994,#44993,#36400,.T.);
#59678=EDGE_CURVE('',#44991,#44994,#24596,.T.);
#59679=EDGE_CURVE('',#44995,#44996,#36401,.T.);
#59680=EDGE_CURVE('',#44996,#44994,#24597,.T.);
#59681=EDGE_CURVE('',#44993,#44997,#24598,.T.);
#59682=EDGE_CURVE('',#44997,#44998,#36402,.T.);
#59683=EDGE_CURVE('',#44998,#44999,#24599,.T.);
#59684=EDGE_CURVE('',#44999,#45000,#36403,.T.);
#59685=EDGE_CURVE('',#45000,#45001,#24600,.T.);
#59686=EDGE_CURVE('',#45001,#45002,#36404,.T.);
#59687=EDGE_CURVE('',#45002,#45003,#24601,.T.);
#59688=EDGE_CURVE('',#45003,#45004,#36405,.T.);
#59689=EDGE_CURVE('',#45004,#45005,#24602,.T.);
#59690=EDGE_CURVE('',#45005,#45006,#36406,.T.);
#59691=EDGE_CURVE('',#45006,#45007,#24603,.T.);
#59692=EDGE_CURVE('',#45007,#45008,#36407,.T.);
#59693=EDGE_CURVE('',#45008,#44995,#24604,.T.);
#59694=EDGE_CURVE('',#45009,#45008,#24605,.T.);
#59695=EDGE_CURVE('',#45009,#45010,#24606,.T.);
#59696=EDGE_CURVE('',#45010,#44995,#24607,.T.);
#59697=EDGE_CURVE('',#45011,#45007,#24608,.T.);
#59698=EDGE_CURVE('',#45011,#45009,#36408,.T.);
#59699=EDGE_CURVE('',#45012,#45006,#24609,.T.);
#59700=EDGE_CURVE('',#45012,#45011,#24610,.T.);
#59701=EDGE_CURVE('',#45013,#45005,#24611,.T.);
#59702=EDGE_CURVE('',#45013,#45012,#36409,.T.);
#59703=EDGE_CURVE('',#45014,#45004,#24612,.T.);
#59704=EDGE_CURVE('',#45014,#45013,#24613,.T.);
#59705=EDGE_CURVE('',#45015,#45003,#24614,.T.);
#59706=EDGE_CURVE('',#45015,#45014,#36410,.T.);
#59707=EDGE_CURVE('',#45016,#45002,#24615,.T.);
#59708=EDGE_CURVE('',#45016,#45015,#24616,.T.);
#59709=EDGE_CURVE('',#45017,#45001,#24617,.T.);
#59710=EDGE_CURVE('',#45017,#45016,#36411,.T.);
#59711=EDGE_CURVE('',#45018,#45000,#24618,.T.);
#59712=EDGE_CURVE('',#45018,#45017,#24619,.T.);
#59713=EDGE_CURVE('',#45019,#44999,#24620,.T.);
#59714=EDGE_CURVE('',#45019,#45018,#36412,.T.);
#59715=EDGE_CURVE('',#45020,#44998,#24621,.T.);
#59716=EDGE_CURVE('',#45020,#45019,#24622,.T.);
#59717=EDGE_CURVE('',#45021,#44997,#24623,.T.);
#59718=EDGE_CURVE('',#45021,#45020,#36413,.T.);
#59719=EDGE_CURVE('',#44992,#45021,#24624,.T.);
#59720=EDGE_CURVE('',#45022,#44996,#24625,.T.);
#59721=EDGE_CURVE('',#45022,#44991,#24626,.T.);
#59722=EDGE_CURVE('',#45010,#45022,#36414,.T.);
#59723=EDGE_CURVE('',#45023,#45024,#36415,.T.);
#59724=EDGE_CURVE('',#45024,#45025,#24627,.T.);
#59725=EDGE_CURVE('',#45025,#45026,#36416,.T.);
#59726=EDGE_CURVE('',#45026,#45027,#24628,.T.);
#59727=EDGE_CURVE('',#45027,#45028,#36417,.T.);
#59728=EDGE_CURVE('',#45028,#45029,#24629,.T.);
#59729=EDGE_CURVE('',#45029,#45030,#36418,.T.);
#59730=EDGE_CURVE('',#45030,#45023,#24630,.T.);
#59731=EDGE_CURVE('',#45031,#45030,#24631,.T.);
#59732=EDGE_CURVE('',#45031,#45032,#24632,.T.);
#59733=EDGE_CURVE('',#45032,#45023,#24633,.T.);
#59734=EDGE_CURVE('',#45033,#45029,#24634,.T.);
#59735=EDGE_CURVE('',#45033,#45031,#36419,.T.);
#59736=EDGE_CURVE('',#45034,#45028,#24635,.T.);
#59737=EDGE_CURVE('',#45034,#45033,#24636,.T.);
#59738=EDGE_CURVE('',#45035,#45027,#24637,.T.);
#59739=EDGE_CURVE('',#45035,#45034,#36420,.T.);
#59740=EDGE_CURVE('',#45036,#45026,#24638,.T.);
#59741=EDGE_CURVE('',#45036,#45035,#24639,.T.);
#59742=EDGE_CURVE('',#45037,#45025,#24640,.T.);
#59743=EDGE_CURVE('',#45037,#45036,#36421,.T.);
#59744=EDGE_CURVE('',#45038,#45024,#24641,.T.);
#59745=EDGE_CURVE('',#45038,#45037,#24642,.T.);
#59746=EDGE_CURVE('',#45032,#45038,#36422,.T.);
#59747=EDGE_CURVE('',#45039,#45040,#24643,.T.);
#59748=EDGE_CURVE('',#45039,#45041,#24644,.T.);
#59749=EDGE_CURVE('',#45041,#45042,#24645,.T.);
#59750=EDGE_CURVE('',#45042,#45040,#24646,.T.);
#59751=EDGE_CURVE('',#45043,#45044,#24647,.T.);
#59752=EDGE_CURVE('',#45043,#45045,#24648,.T.);
#59753=EDGE_CURVE('',#45045,#45046,#24649,.T.);
#59754=EDGE_CURVE('',#45044,#45046,#24650,.T.);
#59755=EDGE_CURVE('',#45047,#45048,#24651,.T.);
#59756=EDGE_CURVE('',#45047,#45049,#24652,.T.);
#59757=EDGE_CURVE('',#45049,#45050,#24653,.T.);
#59758=EDGE_CURVE('',#45048,#45050,#24654,.T.);
#59759=EDGE_CURVE('',#45048,#45051,#24655,.T.);
#59760=EDGE_CURVE('',#45050,#45052,#24656,.T.);
#59761=EDGE_CURVE('',#45051,#45052,#24657,.T.);
#59762=EDGE_CURVE('',#45051,#45053,#24658,.T.);
#59763=EDGE_CURVE('',#45052,#45054,#24659,.T.);
#59764=EDGE_CURVE('',#45053,#45054,#24660,.T.);
#59765=EDGE_CURVE('',#45053,#45055,#36423,.T.);
#59766=EDGE_CURVE('',#45054,#45056,#36424,.T.);
#59767=EDGE_CURVE('',#45055,#45056,#24661,.T.);
#59768=EDGE_CURVE('',#45055,#45057,#24662,.T.);
#59769=EDGE_CURVE('',#45056,#45058,#24663,.T.);
#59770=EDGE_CURVE('',#45057,#45058,#24664,.T.);
#59771=EDGE_CURVE('',#45057,#45059,#36425,.T.);
#59772=EDGE_CURVE('',#45058,#45060,#36426,.T.);
#59773=EDGE_CURVE('',#45059,#45060,#24665,.T.);
#59774=EDGE_CURVE('',#45059,#45061,#24666,.T.);
#59775=EDGE_CURVE('',#45060,#45062,#24667,.T.);
#59776=EDGE_CURVE('',#45061,#45062,#24668,.T.);
#59777=EDGE_CURVE('',#45061,#45063,#36427,.T.);
#59778=EDGE_CURVE('',#45062,#45064,#36428,.T.);
#59779=EDGE_CURVE('',#45063,#45064,#24669,.T.);
#59780=EDGE_CURVE('',#45063,#45065,#24670,.T.);
#59781=EDGE_CURVE('',#45064,#45066,#24671,.T.);
#59782=EDGE_CURVE('',#45065,#45066,#24672,.T.);
#59783=EDGE_CURVE('',#45065,#45067,#36429,.T.);
#59784=EDGE_CURVE('',#45066,#45068,#36430,.T.);
#59785=EDGE_CURVE('',#45067,#45068,#24673,.T.);
#59786=EDGE_CURVE('',#45067,#45069,#24674,.T.);
#59787=EDGE_CURVE('',#45068,#45070,#24675,.T.);
#59788=EDGE_CURVE('',#45069,#45070,#24676,.T.);
#59789=EDGE_CURVE('',#45069,#45071,#24677,.T.);
#59790=EDGE_CURVE('',#45070,#45072,#24678,.T.);
#59791=EDGE_CURVE('',#45071,#45072,#24679,.T.);
#59792=EDGE_CURVE('',#45071,#45073,#24680,.T.);
#59793=EDGE_CURVE('',#45072,#45074,#24681,.T.);
#59794=EDGE_CURVE('',#45073,#45074,#24682,.T.);
#59795=EDGE_CURVE('',#45073,#45075,#24683,.T.);
#59796=EDGE_CURVE('',#45074,#45076,#24684,.T.);
#59797=EDGE_CURVE('',#45075,#45076,#24685,.T.);
#59798=EDGE_CURVE('',#45077,#45078,#24686,.T.);
#59799=EDGE_CURVE('',#45077,#45079,#24687,.T.);
#59800=EDGE_CURVE('',#45079,#45080,#24688,.T.);
#59801=EDGE_CURVE('',#45078,#45080,#24689,.T.);
#59802=EDGE_CURVE('',#45078,#45081,#24690,.T.);
#59803=EDGE_CURVE('',#45080,#45082,#24691,.T.);
#59804=EDGE_CURVE('',#45081,#45082,#24692,.T.);
#59805=EDGE_CURVE('',#45081,#45083,#24693,.T.);
#59806=EDGE_CURVE('',#45082,#45084,#24694,.T.);
#59807=EDGE_CURVE('',#45083,#45084,#24695,.T.);
#59808=EDGE_CURVE('',#45083,#45085,#24696,.T.);
#59809=EDGE_CURVE('',#45084,#45086,#24697,.T.);
#59810=EDGE_CURVE('',#45085,#45086,#24698,.T.);
#59811=EDGE_CURVE('',#45085,#45087,#36431,.T.);
#59812=EDGE_CURVE('',#45086,#45088,#36432,.T.);
#59813=EDGE_CURVE('',#45087,#45088,#24699,.T.);
#59814=EDGE_CURVE('',#45087,#45089,#24700,.T.);
#59815=EDGE_CURVE('',#45088,#45090,#24701,.T.);
#59816=EDGE_CURVE('',#45089,#45090,#24702,.T.);
#59817=EDGE_CURVE('',#45089,#45091,#36433,.T.);
#59818=EDGE_CURVE('',#45090,#45092,#36434,.T.);
#59819=EDGE_CURVE('',#45091,#45092,#24703,.T.);
#59820=EDGE_CURVE('',#45091,#45093,#24704,.T.);
#59821=EDGE_CURVE('',#45092,#45094,#24705,.T.);
#59822=EDGE_CURVE('',#45093,#45094,#24706,.T.);
#59823=EDGE_CURVE('',#45093,#45095,#36435,.T.);
#59824=EDGE_CURVE('',#45094,#45096,#36436,.T.);
#59825=EDGE_CURVE('',#45095,#45096,#24707,.T.);
#59826=EDGE_CURVE('',#45095,#45097,#24708,.T.);
#59827=EDGE_CURVE('',#45096,#45098,#24709,.T.);
#59828=EDGE_CURVE('',#45097,#45098,#24710,.T.);
#59829=EDGE_CURVE('',#45097,#45099,#36437,.T.);
#59830=EDGE_CURVE('',#45098,#45100,#36438,.T.);
#59831=EDGE_CURVE('',#45099,#45100,#24711,.T.);
#59832=EDGE_CURVE('',#45099,#45101,#24712,.T.);
#59833=EDGE_CURVE('',#45100,#45102,#24713,.T.);
#59834=EDGE_CURVE('',#45101,#45102,#24714,.T.);
#59835=EDGE_CURVE('',#45101,#45103,#24715,.T.);
#59836=EDGE_CURVE('',#45102,#45104,#24716,.T.);
#59837=EDGE_CURVE('',#45103,#45104,#24717,.T.);
#59838=EDGE_CURVE('',#45103,#45105,#24718,.T.);
#59839=EDGE_CURVE('',#45104,#45106,#24719,.T.);
#59840=EDGE_CURVE('',#45105,#45106,#24720,.T.);
#59841=EDGE_CURVE('',#45105,#45107,#24721,.T.);
#59842=EDGE_CURVE('',#45106,#45108,#24722,.T.);
#59843=EDGE_CURVE('',#45107,#45108,#24723,.T.);
#59844=EDGE_CURVE('',#45107,#45109,#36439,.T.);
#59845=EDGE_CURVE('',#45108,#45110,#36440,.T.);
#59846=EDGE_CURVE('',#45109,#45110,#24724,.T.);
#59847=EDGE_CURVE('',#45109,#45111,#24725,.T.);
#59848=EDGE_CURVE('',#45110,#45112,#24726,.T.);
#59849=EDGE_CURVE('',#45111,#45112,#24727,.T.);
#59850=EDGE_CURVE('',#45111,#45113,#36441,.T.);
#59851=EDGE_CURVE('',#45112,#45114,#36442,.T.);
#59852=EDGE_CURVE('',#45113,#45114,#24728,.T.);
#59853=EDGE_CURVE('',#45113,#45115,#24729,.T.);
#59854=EDGE_CURVE('',#45114,#45116,#24730,.T.);
#59855=EDGE_CURVE('',#45115,#45116,#24731,.T.);
#59856=EDGE_CURVE('',#45115,#45039,#36443,.T.);
#59857=EDGE_CURVE('',#45116,#45041,#36444,.T.);
#59858=EDGE_CURVE('',#45117,#45118,#24732,.T.);
#59859=EDGE_CURVE('',#45117,#45119,#24733,.T.);
#59860=EDGE_CURVE('',#45119,#45120,#24734,.T.);
#59861=EDGE_CURVE('',#45118,#45120,#24735,.T.);
#59862=EDGE_CURVE('',#45118,#45121,#36445,.T.);
#59863=EDGE_CURVE('',#45120,#45122,#36446,.T.);
#59864=EDGE_CURVE('',#45121,#45122,#24736,.T.);
#59865=EDGE_CURVE('',#45121,#45123,#24737,.T.);
#59866=EDGE_CURVE('',#45122,#45124,#24738,.T.);
#59867=EDGE_CURVE('',#45123,#45124,#24739,.T.);
#59868=EDGE_CURVE('',#45123,#45125,#24740,.T.);
#59869=EDGE_CURVE('',#45124,#45126,#24741,.T.);
#59870=EDGE_CURVE('',#45125,#45126,#24742,.T.);
#59871=EDGE_CURVE('',#45125,#45127,#24743,.T.);
#59872=EDGE_CURVE('',#45126,#45128,#24744,.T.);
#59873=EDGE_CURVE('',#45127,#45128,#24745,.T.);
#59874=EDGE_CURVE('',#45127,#45129,#24746,.T.);
#59875=EDGE_CURVE('',#45128,#45130,#24747,.T.);
#59876=EDGE_CURVE('',#45129,#45130,#24748,.T.);
#59877=EDGE_CURVE('',#45129,#45131,#36447,.T.);
#59878=EDGE_CURVE('',#45130,#45132,#36448,.T.);
#59879=EDGE_CURVE('',#45131,#45132,#24749,.T.);
#59880=EDGE_CURVE('',#45131,#45133,#24750,.T.);
#59881=EDGE_CURVE('',#45132,#45134,#24751,.T.);
#59882=EDGE_CURVE('',#45133,#45134,#24752,.T.);
#59883=EDGE_CURVE('',#45133,#45135,#24753,.T.);
#59884=EDGE_CURVE('',#45134,#45136,#24754,.T.);
#59885=EDGE_CURVE('',#45135,#45136,#24755,.T.);
#59886=EDGE_CURVE('',#45135,#45137,#24756,.T.);
#59887=EDGE_CURVE('',#45136,#45138,#24757,.T.);
#59888=EDGE_CURVE('',#45137,#45138,#24758,.T.);
#59889=EDGE_CURVE('',#45137,#45139,#24759,.T.);
#59890=EDGE_CURVE('',#45138,#45140,#24760,.T.);
#59891=EDGE_CURVE('',#45139,#45140,#24761,.T.);
#59892=EDGE_CURVE('',#45139,#45141,#36449,.T.);
#59893=EDGE_CURVE('',#45140,#45142,#36450,.T.);
#59894=EDGE_CURVE('',#45141,#45142,#24762,.T.);
#59895=EDGE_CURVE('',#45141,#45143,#24763,.T.);
#59896=EDGE_CURVE('',#45142,#45144,#24764,.T.);
#59897=EDGE_CURVE('',#45144,#45143,#24765,.T.);
#59898=EDGE_CURVE('',#45044,#45145,#36451,.T.);
#59899=EDGE_CURVE('',#45046,#45146,#36452,.T.);
#59900=EDGE_CURVE('',#45145,#45146,#24766,.T.);
#59901=EDGE_CURVE('',#45145,#45147,#24767,.T.);
#59902=EDGE_CURVE('',#45146,#45148,#24768,.T.);
#59903=EDGE_CURVE('',#45147,#45148,#24769,.T.);
#59904=EDGE_CURVE('',#45147,#45149,#36453,.T.);
#59905=EDGE_CURVE('',#45148,#45150,#36454,.T.);
#59906=EDGE_CURVE('',#45149,#45150,#24770,.T.);
#59907=EDGE_CURVE('',#45149,#45151,#24771,.T.);
#59908=EDGE_CURVE('',#45150,#45152,#24772,.T.);
#59909=EDGE_CURVE('',#45151,#45152,#24773,.T.);
#59910=EDGE_CURVE('',#45151,#45153,#36455,.T.);
#59911=EDGE_CURVE('',#45152,#45154,#36456,.T.);
#59912=EDGE_CURVE('',#45153,#45154,#24774,.T.);
#59913=EDGE_CURVE('',#45153,#45047,#24775,.T.);
#59914=EDGE_CURVE('',#45154,#45049,#24776,.T.);
#59915=EDGE_CURVE('',#45155,#45156,#24777,.T.);
#59916=EDGE_CURVE('',#45155,#45157,#24778,.T.);
#59917=EDGE_CURVE('',#45157,#45158,#24779,.T.);
#59918=EDGE_CURVE('',#45156,#45158,#24780,.T.);
#59919=EDGE_CURVE('',#45156,#45159,#24781,.T.);
#59920=EDGE_CURVE('',#45158,#45160,#24782,.T.);
#59921=EDGE_CURVE('',#45159,#45160,#24783,.T.);
#59922=EDGE_CURVE('',#45159,#45161,#24784,.T.);
#59923=EDGE_CURVE('',#45160,#45162,#24785,.T.);
#59924=EDGE_CURVE('',#45161,#45162,#24786,.T.);
#59925=EDGE_CURVE('',#45161,#45163,#36457,.T.);
#59926=EDGE_CURVE('',#45162,#45164,#36458,.T.);
#59927=EDGE_CURVE('',#45163,#45164,#24787,.T.);
#59928=EDGE_CURVE('',#45163,#45165,#24788,.T.);
#59929=EDGE_CURVE('',#45164,#45166,#24789,.T.);
#59930=EDGE_CURVE('',#45165,#45166,#24790,.T.);
#59931=EDGE_CURVE('',#45165,#45167,#36459,.T.);
#59932=EDGE_CURVE('',#45166,#45168,#36460,.T.);
#59933=EDGE_CURVE('',#45167,#45168,#24791,.T.);
#59934=EDGE_CURVE('',#45167,#45169,#24792,.T.);
#59935=EDGE_CURVE('',#45168,#45170,#24793,.T.);
#59936=EDGE_CURVE('',#45169,#45170,#24794,.T.);
#59937=EDGE_CURVE('',#45169,#45171,#36461,.T.);
#59938=EDGE_CURVE('',#45170,#45172,#36462,.T.);
#59939=EDGE_CURVE('',#45171,#45172,#24795,.T.);
#59940=EDGE_CURVE('',#45171,#45173,#24796,.T.);
#59941=EDGE_CURVE('',#45172,#45174,#24797,.T.);
#59942=EDGE_CURVE('',#45173,#45174,#24798,.T.);
#59943=EDGE_CURVE('',#45173,#45175,#36463,.T.);
#59944=EDGE_CURVE('',#45174,#45176,#36464,.T.);
#59945=EDGE_CURVE('',#45175,#45176,#24799,.T.);
#59946=EDGE_CURVE('',#45175,#45177,#24800,.T.);
#59947=EDGE_CURVE('',#45176,#45178,#24801,.T.);
#59948=EDGE_CURVE('',#45177,#45178,#24802,.T.);
#59949=EDGE_CURVE('',#45177,#45179,#24803,.T.);
#59950=EDGE_CURVE('',#45178,#45180,#24804,.T.);
#59951=EDGE_CURVE('',#45179,#45180,#24805,.T.);
#59952=EDGE_CURVE('',#45179,#45077,#24806,.T.);
#59953=EDGE_CURVE('',#45180,#45079,#24807,.T.);
#59954=EDGE_CURVE('',#45181,#45182,#24808,.T.);
#59955=EDGE_CURVE('',#45181,#45183,#24809,.T.);
#59956=EDGE_CURVE('',#45183,#45184,#24810,.T.);
#59957=EDGE_CURVE('',#45182,#45184,#24811,.T.);
#59958=EDGE_CURVE('',#45182,#45185,#24812,.T.);
#59959=EDGE_CURVE('',#45184,#45186,#24813,.T.);
#59960=EDGE_CURVE('',#45185,#45186,#24814,.T.);
#59961=EDGE_CURVE('',#45185,#45187,#24815,.T.);
#59962=EDGE_CURVE('',#45186,#45188,#24816,.T.);
#59963=EDGE_CURVE('',#45187,#45188,#24817,.T.);
#59964=EDGE_CURVE('',#45187,#45189,#24818,.T.);
#59965=EDGE_CURVE('',#45188,#45190,#24819,.T.);
#59966=EDGE_CURVE('',#45189,#45190,#24820,.T.);
#59967=EDGE_CURVE('',#45189,#45191,#36465,.T.);
#59968=EDGE_CURVE('',#45190,#45192,#36466,.T.);
#59969=EDGE_CURVE('',#45191,#45192,#24821,.T.);
#59970=EDGE_CURVE('',#45191,#45193,#24822,.T.);
#59971=EDGE_CURVE('',#45192,#45194,#24823,.T.);
#59972=EDGE_CURVE('',#45193,#45194,#24824,.T.);
#59973=EDGE_CURVE('',#45193,#45195,#36467,.T.);
#59974=EDGE_CURVE('',#45194,#45196,#36468,.T.);
#59975=EDGE_CURVE('',#45195,#45196,#24825,.T.);
#59976=EDGE_CURVE('',#45195,#45197,#24826,.T.);
#59977=EDGE_CURVE('',#45196,#45198,#24827,.T.);
#59978=EDGE_CURVE('',#45197,#45198,#24828,.T.);
#59979=EDGE_CURVE('',#45197,#45199,#36469,.T.);
#59980=EDGE_CURVE('',#45198,#45200,#36470,.T.);
#59981=EDGE_CURVE('',#45199,#45200,#24829,.T.);
#59982=EDGE_CURVE('',#45199,#45201,#24830,.T.);
#59983=EDGE_CURVE('',#45200,#45202,#24831,.T.);
#59984=EDGE_CURVE('',#45201,#45202,#24832,.T.);
#59985=EDGE_CURVE('',#45201,#45203,#36471,.T.);
#59986=EDGE_CURVE('',#45202,#45204,#36472,.T.);
#59987=EDGE_CURVE('',#45203,#45204,#24833,.T.);
#59988=EDGE_CURVE('',#45203,#45205,#24834,.T.);
#59989=EDGE_CURVE('',#45204,#45206,#24835,.T.);
#59990=EDGE_CURVE('',#45205,#45206,#24836,.T.);
#59991=EDGE_CURVE('',#45205,#45207,#24837,.T.);
#59992=EDGE_CURVE('',#45206,#45208,#24838,.T.);
#59993=EDGE_CURVE('',#45207,#45208,#24839,.T.);
#59994=EDGE_CURVE('',#45207,#45209,#24840,.T.);
#59995=EDGE_CURVE('',#45208,#45210,#24841,.T.);
#59996=EDGE_CURVE('',#45209,#45210,#24842,.T.);
#59997=EDGE_CURVE('',#45209,#45211,#24843,.T.);
#59998=EDGE_CURVE('',#45210,#45212,#24844,.T.);
#59999=EDGE_CURVE('',#45211,#45212,#24845,.T.);
#60000=EDGE_CURVE('',#45211,#45213,#36473,.T.);
#60001=EDGE_CURVE('',#45212,#45214,#36474,.T.);
#60002=EDGE_CURVE('',#45213,#45214,#24846,.T.);
#60003=EDGE_CURVE('',#45213,#45215,#24847,.T.);
#60004=EDGE_CURVE('',#45214,#45216,#24848,.T.);
#60005=EDGE_CURVE('',#45215,#45216,#24849,.T.);
#60006=EDGE_CURVE('',#45215,#45217,#36475,.T.);
#60007=EDGE_CURVE('',#45216,#45218,#36476,.T.);
#60008=EDGE_CURVE('',#45217,#45218,#24850,.T.);
#60009=EDGE_CURVE('',#45217,#45219,#24851,.T.);
#60010=EDGE_CURVE('',#45218,#45220,#24852,.T.);
#60011=EDGE_CURVE('',#45219,#45220,#24853,.T.);
#60012=EDGE_CURVE('',#45219,#45221,#36477,.T.);
#60013=EDGE_CURVE('',#45220,#45222,#36478,.T.);
#60014=EDGE_CURVE('',#45221,#45222,#24854,.T.);
#60015=EDGE_CURVE('',#45221,#45223,#24855,.T.);
#60016=EDGE_CURVE('',#45222,#45224,#24856,.T.);
#60017=EDGE_CURVE('',#45223,#45224,#24857,.T.);
#60018=EDGE_CURVE('',#45223,#45225,#36479,.T.);
#60019=EDGE_CURVE('',#45224,#45226,#36480,.T.);
#60020=EDGE_CURVE('',#45225,#45226,#24858,.T.);
#60021=EDGE_CURVE('',#45225,#45227,#24859,.T.);
#60022=EDGE_CURVE('',#45226,#45228,#24860,.T.);
#60023=EDGE_CURVE('',#45227,#45228,#24861,.T.);
#60024=EDGE_CURVE('',#45227,#45229,#24862,.T.);
#60025=EDGE_CURVE('',#45228,#45230,#24863,.T.);
#60026=EDGE_CURVE('',#45229,#45230,#24864,.T.);
#60027=EDGE_CURVE('',#45229,#45231,#24865,.T.);
#60028=EDGE_CURVE('',#45230,#45232,#24866,.T.);
#60029=EDGE_CURVE('',#45231,#45232,#24867,.T.);
#60030=EDGE_CURVE('',#45231,#45233,#24868,.T.);
#60031=EDGE_CURVE('',#45232,#45234,#24869,.T.);
#60032=EDGE_CURVE('',#45233,#45234,#24870,.T.);
#60033=EDGE_CURVE('',#45233,#45235,#36481,.T.);
#60034=EDGE_CURVE('',#45234,#45236,#36482,.T.);
#60035=EDGE_CURVE('',#45235,#45236,#24871,.T.);
#60036=EDGE_CURVE('',#45235,#45237,#24872,.T.);
#60037=EDGE_CURVE('',#45236,#45238,#24873,.T.);
#60038=EDGE_CURVE('',#45237,#45238,#24874,.T.);
#60039=EDGE_CURVE('',#45237,#45239,#24875,.T.);
#60040=EDGE_CURVE('',#45238,#45240,#24876,.T.);
#60041=EDGE_CURVE('',#45239,#45240,#24877,.T.);
#60042=EDGE_CURVE('',#45239,#45241,#24878,.T.);
#60043=EDGE_CURVE('',#45240,#45242,#24879,.T.);
#60044=EDGE_CURVE('',#45241,#45242,#24880,.T.);
#60045=EDGE_CURVE('',#45241,#45243,#24881,.T.);
#60046=EDGE_CURVE('',#45242,#45244,#24882,.T.);
#60047=EDGE_CURVE('',#45243,#45244,#24883,.T.);
#60048=EDGE_CURVE('',#45243,#45245,#36483,.T.);
#60049=EDGE_CURVE('',#45244,#45246,#36484,.T.);
#60050=EDGE_CURVE('',#45245,#45246,#24884,.T.);
#60051=EDGE_CURVE('',#45245,#45247,#24885,.T.);
#60052=EDGE_CURVE('',#45246,#45248,#24886,.T.);
#60053=EDGE_CURVE('',#45247,#45248,#24887,.T.);
#60054=EDGE_CURVE('',#45247,#45249,#36485,.T.);
#60055=EDGE_CURVE('',#45248,#45250,#36486,.T.);
#60056=EDGE_CURVE('',#45249,#45250,#24888,.T.);
#60057=EDGE_CURVE('',#45249,#45251,#24889,.T.);
#60058=EDGE_CURVE('',#45250,#45252,#24890,.T.);
#60059=EDGE_CURVE('',#45251,#45252,#24891,.T.);
#60060=EDGE_CURVE('',#45251,#45253,#36487,.T.);
#60061=EDGE_CURVE('',#45252,#45254,#36488,.T.);
#60062=EDGE_CURVE('',#45253,#45254,#24892,.T.);
#60063=EDGE_CURVE('',#45253,#45255,#24893,.T.);
#60064=EDGE_CURVE('',#45254,#45256,#24894,.T.);
#60065=EDGE_CURVE('',#45255,#45256,#24895,.T.);
#60066=EDGE_CURVE('',#45255,#45257,#36489,.T.);
#60067=EDGE_CURVE('',#45256,#45258,#36490,.T.);
#60068=EDGE_CURVE('',#45257,#45258,#24896,.T.);
#60069=EDGE_CURVE('',#45257,#45155,#24897,.T.);
#60070=EDGE_CURVE('',#45258,#45157,#24898,.T.);
#60071=EDGE_CURVE('',#45259,#45260,#24899,.T.);
#60072=EDGE_CURVE('',#45259,#45261,#24900,.T.);
#60073=EDGE_CURVE('',#45261,#45262,#24901,.T.);
#60074=EDGE_CURVE('',#45260,#45262,#24902,.T.);
#60075=EDGE_CURVE('',#45260,#45263,#24903,.T.);
#60076=EDGE_CURVE('',#45262,#45264,#24904,.T.);
#60077=EDGE_CURVE('',#45263,#45264,#24905,.T.);
#60078=EDGE_CURVE('',#45263,#45265,#24906,.T.);
#60079=EDGE_CURVE('',#45264,#45266,#24907,.T.);
#60080=EDGE_CURVE('',#45265,#45266,#24908,.T.);
#60081=EDGE_CURVE('',#45265,#45267,#36491,.T.);
#60082=EDGE_CURVE('',#45266,#45268,#36492,.T.);
#60083=EDGE_CURVE('',#45267,#45268,#24909,.T.);
#60084=EDGE_CURVE('',#45267,#45269,#24910,.T.);
#60085=EDGE_CURVE('',#45268,#45270,#24911,.T.);
#60086=EDGE_CURVE('',#45269,#45270,#24912,.T.);
#60087=EDGE_CURVE('',#45269,#45271,#36493,.T.);
#60088=EDGE_CURVE('',#45270,#45272,#36494,.T.);
#60089=EDGE_CURVE('',#45271,#45272,#24913,.T.);
#60090=EDGE_CURVE('',#45271,#45273,#24914,.T.);
#60091=EDGE_CURVE('',#45272,#45274,#24915,.T.);
#60092=EDGE_CURVE('',#45273,#45274,#24916,.T.);
#60093=EDGE_CURVE('',#45273,#45275,#36495,.T.);
#60094=EDGE_CURVE('',#45274,#45276,#36496,.T.);
#60095=EDGE_CURVE('',#45275,#45276,#24917,.T.);
#60096=EDGE_CURVE('',#45275,#45277,#24918,.T.);
#60097=EDGE_CURVE('',#45276,#45278,#24919,.T.);
#60098=EDGE_CURVE('',#45277,#45278,#24920,.T.);
#60099=EDGE_CURVE('',#45277,#45279,#36497,.T.);
#60100=EDGE_CURVE('',#45278,#45280,#36498,.T.);
#60101=EDGE_CURVE('',#45279,#45280,#24921,.T.);
#60102=EDGE_CURVE('',#45279,#45281,#24922,.T.);
#60103=EDGE_CURVE('',#45280,#45282,#24923,.T.);
#60104=EDGE_CURVE('',#45281,#45282,#24924,.T.);
#60105=EDGE_CURVE('',#45281,#45283,#24925,.T.);
#60106=EDGE_CURVE('',#45282,#45284,#24926,.T.);
#60107=EDGE_CURVE('',#45283,#45284,#24927,.T.);
#60108=EDGE_CURVE('',#45283,#45181,#24928,.T.);
#60109=EDGE_CURVE('',#45284,#45183,#24929,.T.);
#60110=EDGE_CURVE('',#45285,#45286,#24930,.T.);
#60111=EDGE_CURVE('',#45285,#45287,#24931,.T.);
#60112=EDGE_CURVE('',#45287,#45288,#24932,.T.);
#60113=EDGE_CURVE('',#45286,#45288,#24933,.T.);
#60114=EDGE_CURVE('',#45286,#45289,#24934,.T.);
#60115=EDGE_CURVE('',#45288,#45290,#24935,.T.);
#60116=EDGE_CURVE('',#45289,#45290,#24936,.T.);
#60117=EDGE_CURVE('',#45289,#45291,#24937,.T.);
#60118=EDGE_CURVE('',#45290,#45292,#24938,.T.);
#60119=EDGE_CURVE('',#45291,#45292,#24939,.T.);
#60120=EDGE_CURVE('',#45291,#45293,#24940,.T.);
#60121=EDGE_CURVE('',#45292,#45294,#24941,.T.);
#60122=EDGE_CURVE('',#45293,#45294,#24942,.T.);
#60123=EDGE_CURVE('',#45293,#45295,#36499,.T.);
#60124=EDGE_CURVE('',#45294,#45296,#36500,.T.);
#60125=EDGE_CURVE('',#45295,#45296,#24943,.T.);
#60126=EDGE_CURVE('',#45295,#45297,#24944,.T.);
#60127=EDGE_CURVE('',#45296,#45298,#24945,.T.);
#60128=EDGE_CURVE('',#45297,#45298,#24946,.T.);
#60129=EDGE_CURVE('',#45297,#45299,#36501,.T.);
#60130=EDGE_CURVE('',#45298,#45300,#36502,.T.);
#60131=EDGE_CURVE('',#45299,#45300,#24947,.T.);
#60132=EDGE_CURVE('',#45299,#45301,#24948,.T.);
#60133=EDGE_CURVE('',#45300,#45302,#24949,.T.);
#60134=EDGE_CURVE('',#45301,#45302,#24950,.T.);
#60135=EDGE_CURVE('',#45301,#45303,#36503,.T.);
#60136=EDGE_CURVE('',#45302,#45304,#36504,.T.);
#60137=EDGE_CURVE('',#45303,#45304,#24951,.T.);
#60138=EDGE_CURVE('',#45303,#45305,#24952,.T.);
#60139=EDGE_CURVE('',#45304,#45306,#24953,.T.);
#60140=EDGE_CURVE('',#45305,#45306,#24954,.T.);
#60141=EDGE_CURVE('',#45305,#45307,#36505,.T.);
#60142=EDGE_CURVE('',#45306,#45308,#36506,.T.);
#60143=EDGE_CURVE('',#45307,#45308,#24955,.T.);
#60144=EDGE_CURVE('',#45307,#45309,#24956,.T.);
#60145=EDGE_CURVE('',#45308,#45310,#24957,.T.);
#60146=EDGE_CURVE('',#45309,#45310,#24958,.T.);
#60147=EDGE_CURVE('',#45309,#45311,#24959,.T.);
#60148=EDGE_CURVE('',#45310,#45312,#24960,.T.);
#60149=EDGE_CURVE('',#45311,#45312,#24961,.T.);
#60150=EDGE_CURVE('',#45311,#45313,#24962,.T.);
#60151=EDGE_CURVE('',#45312,#45314,#24963,.T.);
#60152=EDGE_CURVE('',#45313,#45314,#24964,.T.);
#60153=EDGE_CURVE('',#45313,#45315,#24965,.T.);
#60154=EDGE_CURVE('',#45314,#45316,#24966,.T.);
#60155=EDGE_CURVE('',#45315,#45316,#24967,.T.);
#60156=EDGE_CURVE('',#45315,#45317,#36507,.T.);
#60157=EDGE_CURVE('',#45316,#45318,#36508,.T.);
#60158=EDGE_CURVE('',#45317,#45318,#24968,.T.);
#60159=EDGE_CURVE('',#45317,#45319,#24969,.T.);
#60160=EDGE_CURVE('',#45318,#45320,#24970,.T.);
#60161=EDGE_CURVE('',#45319,#45320,#24971,.T.);
#60162=EDGE_CURVE('',#45319,#45321,#36509,.T.);
#60163=EDGE_CURVE('',#45320,#45322,#36510,.T.);
#60164=EDGE_CURVE('',#45321,#45322,#24972,.T.);
#60165=EDGE_CURVE('',#45321,#45323,#24973,.T.);
#60166=EDGE_CURVE('',#45322,#45324,#24974,.T.);
#60167=EDGE_CURVE('',#45323,#45324,#24975,.T.);
#60168=EDGE_CURVE('',#45323,#45325,#36511,.T.);
#60169=EDGE_CURVE('',#45324,#45326,#36512,.T.);
#60170=EDGE_CURVE('',#45325,#45326,#24976,.T.);
#60171=EDGE_CURVE('',#45325,#45327,#24977,.T.);
#60172=EDGE_CURVE('',#45326,#45328,#24978,.T.);
#60173=EDGE_CURVE('',#45327,#45328,#24979,.T.);
#60174=EDGE_CURVE('',#45327,#45329,#36513,.T.);
#60175=EDGE_CURVE('',#45328,#45330,#36514,.T.);
#60176=EDGE_CURVE('',#45329,#45330,#24980,.T.);
#60177=EDGE_CURVE('',#45329,#45331,#24981,.T.);
#60178=EDGE_CURVE('',#45330,#45332,#24982,.T.);
#60179=EDGE_CURVE('',#45331,#45332,#24983,.T.);
#60180=EDGE_CURVE('',#45331,#45333,#24984,.T.);
#60181=EDGE_CURVE('',#45332,#45334,#24985,.T.);
#60182=EDGE_CURVE('',#45333,#45334,#24986,.T.);
#60183=EDGE_CURVE('',#45333,#45335,#24987,.T.);
#60184=EDGE_CURVE('',#45334,#45336,#24988,.T.);
#60185=EDGE_CURVE('',#45335,#45336,#24989,.T.);
#60186=EDGE_CURVE('',#45335,#45337,#24990,.T.);
#60187=EDGE_CURVE('',#45336,#45338,#24991,.T.);
#60188=EDGE_CURVE('',#45337,#45338,#24992,.T.);
#60189=EDGE_CURVE('',#45337,#45339,#36515,.T.);
#60190=EDGE_CURVE('',#45338,#45340,#36516,.T.);
#60191=EDGE_CURVE('',#45339,#45340,#24993,.T.);
#60192=EDGE_CURVE('',#45339,#45341,#24994,.T.);
#60193=EDGE_CURVE('',#45340,#45342,#24995,.T.);
#60194=EDGE_CURVE('',#45341,#45342,#24996,.T.);
#60195=EDGE_CURVE('',#45341,#45343,#24997,.T.);
#60196=EDGE_CURVE('',#45342,#45344,#24998,.T.);
#60197=EDGE_CURVE('',#45343,#45344,#24999,.T.);
#60198=EDGE_CURVE('',#45343,#45345,#25000,.T.);
#60199=EDGE_CURVE('',#45344,#45346,#25001,.T.);
#60200=EDGE_CURVE('',#45345,#45346,#25002,.T.);
#60201=EDGE_CURVE('',#45345,#45347,#25003,.T.);
#60202=EDGE_CURVE('',#45346,#45348,#25004,.T.);
#60203=EDGE_CURVE('',#45347,#45348,#25005,.T.);
#60204=EDGE_CURVE('',#45347,#45349,#36517,.T.);
#60205=EDGE_CURVE('',#45348,#45350,#36518,.T.);
#60206=EDGE_CURVE('',#45349,#45350,#25006,.T.);
#60207=EDGE_CURVE('',#45349,#45351,#25007,.T.);
#60208=EDGE_CURVE('',#45350,#45352,#25008,.T.);
#60209=EDGE_CURVE('',#45351,#45352,#25009,.T.);
#60210=EDGE_CURVE('',#45351,#45353,#36519,.T.);
#60211=EDGE_CURVE('',#45352,#45354,#36520,.T.);
#60212=EDGE_CURVE('',#45353,#45354,#25010,.T.);
#60213=EDGE_CURVE('',#45353,#45355,#25011,.T.);
#60214=EDGE_CURVE('',#45354,#45356,#25012,.T.);
#60215=EDGE_CURVE('',#45355,#45356,#25013,.T.);
#60216=EDGE_CURVE('',#45355,#45357,#36521,.T.);
#60217=EDGE_CURVE('',#45356,#45358,#36522,.T.);
#60218=EDGE_CURVE('',#45357,#45358,#25014,.T.);
#60219=EDGE_CURVE('',#45357,#45359,#25015,.T.);
#60220=EDGE_CURVE('',#45358,#45360,#25016,.T.);
#60221=EDGE_CURVE('',#45359,#45360,#25017,.T.);
#60222=EDGE_CURVE('',#45359,#45361,#36523,.T.);
#60223=EDGE_CURVE('',#45360,#45362,#36524,.T.);
#60224=EDGE_CURVE('',#45361,#45362,#25018,.T.);
#60225=EDGE_CURVE('',#45361,#45259,#25019,.T.);
#60226=EDGE_CURVE('',#45362,#45261,#25020,.T.);
#60227=EDGE_CURVE('',#45363,#45364,#25021,.T.);
#60228=EDGE_CURVE('',#45363,#45365,#25022,.T.);
#60229=EDGE_CURVE('',#45365,#45366,#25023,.T.);
#60230=EDGE_CURVE('',#45364,#45366,#25024,.T.);
#60231=EDGE_CURVE('',#45364,#45367,#25025,.T.);
#60232=EDGE_CURVE('',#45366,#45368,#25026,.T.);
#60233=EDGE_CURVE('',#45367,#45368,#25027,.T.);
#60234=EDGE_CURVE('',#45367,#45369,#25028,.T.);
#60235=EDGE_CURVE('',#45368,#45370,#25029,.T.);
#60236=EDGE_CURVE('',#45369,#45370,#25030,.T.);
#60237=EDGE_CURVE('',#45369,#45371,#36525,.T.);
#60238=EDGE_CURVE('',#45370,#45372,#36526,.T.);
#60239=EDGE_CURVE('',#45371,#45372,#25031,.T.);
#60240=EDGE_CURVE('',#45371,#45373,#25032,.T.);
#60241=EDGE_CURVE('',#45372,#45374,#25033,.T.);
#60242=EDGE_CURVE('',#45373,#45374,#25034,.T.);
#60243=EDGE_CURVE('',#45373,#45375,#36527,.T.);
#60244=EDGE_CURVE('',#45374,#45376,#36528,.T.);
#60245=EDGE_CURVE('',#45375,#45376,#25035,.T.);
#60246=EDGE_CURVE('',#45375,#45377,#25036,.T.);
#60247=EDGE_CURVE('',#45376,#45378,#25037,.T.);
#60248=EDGE_CURVE('',#45377,#45378,#25038,.T.);
#60249=EDGE_CURVE('',#45377,#45379,#36529,.T.);
#60250=EDGE_CURVE('',#45378,#45380,#36530,.T.);
#60251=EDGE_CURVE('',#45379,#45380,#25039,.T.);
#60252=EDGE_CURVE('',#45379,#45381,#25040,.T.);
#60253=EDGE_CURVE('',#45380,#45382,#25041,.T.);
#60254=EDGE_CURVE('',#45381,#45382,#25042,.T.);
#60255=EDGE_CURVE('',#45381,#45383,#36531,.T.);
#60256=EDGE_CURVE('',#45382,#45384,#36532,.T.);
#60257=EDGE_CURVE('',#45383,#45384,#25043,.T.);
#60258=EDGE_CURVE('',#45383,#45385,#25044,.T.);
#60259=EDGE_CURVE('',#45384,#45386,#25045,.T.);
#60260=EDGE_CURVE('',#45385,#45386,#25046,.T.);
#60261=EDGE_CURVE('',#45385,#45387,#25047,.T.);
#60262=EDGE_CURVE('',#45386,#45388,#25048,.T.);
#60263=EDGE_CURVE('',#45387,#45388,#25049,.T.);
#60264=EDGE_CURVE('',#45387,#45285,#25050,.T.);
#60265=EDGE_CURVE('',#45388,#45287,#25051,.T.);
#60266=EDGE_CURVE('',#45075,#45389,#25052,.T.);
#60267=EDGE_CURVE('',#45076,#45390,#25053,.T.);
#60268=EDGE_CURVE('',#45389,#45390,#25054,.T.);
#60269=EDGE_CURVE('',#45389,#45391,#25055,.T.);
#60270=EDGE_CURVE('',#45390,#45392,#25056,.T.);
#60271=EDGE_CURVE('',#45391,#45392,#25057,.T.);
#60272=EDGE_CURVE('',#45391,#45393,#25058,.T.);
#60273=EDGE_CURVE('',#45392,#45394,#25059,.T.);
#60274=EDGE_CURVE('',#45393,#45394,#25060,.T.);
#60275=EDGE_CURVE('',#45393,#45395,#36533,.T.);
#60276=EDGE_CURVE('',#45394,#45396,#36534,.T.);
#60277=EDGE_CURVE('',#45395,#45396,#25061,.T.);
#60278=EDGE_CURVE('',#45395,#45397,#25062,.T.);
#60279=EDGE_CURVE('',#45396,#45398,#25063,.T.);
#60280=EDGE_CURVE('',#45397,#45398,#25064,.T.);
#60281=EDGE_CURVE('',#45397,#45399,#36535,.T.);
#60282=EDGE_CURVE('',#45398,#45400,#36536,.T.);
#60283=EDGE_CURVE('',#45399,#45400,#25065,.T.);
#60284=EDGE_CURVE('',#45399,#45401,#25066,.T.);
#60285=EDGE_CURVE('',#45400,#45402,#25067,.T.);
#60286=EDGE_CURVE('',#45401,#45402,#25068,.T.);
#60287=EDGE_CURVE('',#45401,#45403,#36537,.T.);
#60288=EDGE_CURVE('',#45402,#45404,#36538,.T.);
#60289=EDGE_CURVE('',#45403,#45404,#25069,.T.);
#60290=EDGE_CURVE('',#45403,#45405,#25070,.T.);
#60291=EDGE_CURVE('',#45404,#45406,#25071,.T.);
#60292=EDGE_CURVE('',#45405,#45406,#25072,.T.);
#60293=EDGE_CURVE('',#45405,#45407,#36539,.T.);
#60294=EDGE_CURVE('',#45406,#45408,#36540,.T.);
#60295=EDGE_CURVE('',#45407,#45408,#25073,.T.);
#60296=EDGE_CURVE('',#45407,#45409,#25074,.T.);
#60297=EDGE_CURVE('',#45408,#45410,#25075,.T.);
#60298=EDGE_CURVE('',#45409,#45410,#25076,.T.);
#60299=EDGE_CURVE('',#45409,#45411,#25077,.T.);
#60300=EDGE_CURVE('',#45410,#45412,#25078,.T.);
#60301=EDGE_CURVE('',#45411,#45412,#25079,.T.);
#60302=EDGE_CURVE('',#45411,#45413,#25080,.T.);
#60303=EDGE_CURVE('',#45412,#45414,#25081,.T.);
#60304=EDGE_CURVE('',#45413,#45414,#25082,.T.);
#60305=EDGE_CURVE('',#45413,#45415,#25083,.T.);
#60306=EDGE_CURVE('',#45414,#45416,#25084,.T.);
#60307=EDGE_CURVE('',#45415,#45416,#25085,.T.);
#60308=EDGE_CURVE('',#45415,#45417,#36541,.T.);
#60309=EDGE_CURVE('',#45416,#45418,#36542,.T.);
#60310=EDGE_CURVE('',#45417,#45418,#25086,.T.);
#60311=EDGE_CURVE('',#45417,#45419,#25087,.T.);
#60312=EDGE_CURVE('',#45418,#45420,#25088,.T.);
#60313=EDGE_CURVE('',#45419,#45420,#25089,.T.);
#60314=EDGE_CURVE('',#45419,#45421,#36543,.T.);
#60315=EDGE_CURVE('',#45420,#45422,#36544,.T.);
#60316=EDGE_CURVE('',#45421,#45422,#25090,.T.);
#60317=EDGE_CURVE('',#45421,#45423,#25091,.T.);
#60318=EDGE_CURVE('',#45422,#45424,#25092,.T.);
#60319=EDGE_CURVE('',#45423,#45424,#25093,.T.);
#60320=EDGE_CURVE('',#45423,#45425,#36545,.T.);
#60321=EDGE_CURVE('',#45424,#45426,#36546,.T.);
#60322=EDGE_CURVE('',#45425,#45426,#25094,.T.);
#60323=EDGE_CURVE('',#45425,#45427,#25095,.T.);
#60324=EDGE_CURVE('',#45426,#45428,#25096,.T.);
#60325=EDGE_CURVE('',#45427,#45428,#25097,.T.);
#60326=EDGE_CURVE('',#45427,#45429,#36547,.T.);
#60327=EDGE_CURVE('',#45428,#45430,#36548,.T.);
#60328=EDGE_CURVE('',#45429,#45430,#25098,.T.);
#60329=EDGE_CURVE('',#45429,#45431,#25099,.T.);
#60330=EDGE_CURVE('',#45430,#45432,#25100,.T.);
#60331=EDGE_CURVE('',#45431,#45432,#25101,.T.);
#60332=EDGE_CURVE('',#45431,#45433,#25102,.T.);
#60333=EDGE_CURVE('',#45432,#45434,#25103,.T.);
#60334=EDGE_CURVE('',#45433,#45434,#25104,.T.);
#60335=EDGE_CURVE('',#45433,#45435,#25105,.T.);
#60336=EDGE_CURVE('',#45434,#45436,#25106,.T.);
#60337=EDGE_CURVE('',#45435,#45436,#25107,.T.);
#60338=EDGE_CURVE('',#45435,#45437,#25108,.T.);
#60339=EDGE_CURVE('',#45436,#45438,#25109,.T.);
#60340=EDGE_CURVE('',#45437,#45438,#25110,.T.);
#60341=EDGE_CURVE('',#45437,#45439,#36549,.T.);
#60342=EDGE_CURVE('',#45438,#45440,#36550,.T.);
#60343=EDGE_CURVE('',#45439,#45440,#25111,.T.);
#60344=EDGE_CURVE('',#45439,#45441,#25112,.T.);
#60345=EDGE_CURVE('',#45440,#45442,#25113,.T.);
#60346=EDGE_CURVE('',#45441,#45442,#25114,.T.);
#60347=EDGE_CURVE('',#45441,#45443,#25115,.T.);
#60348=EDGE_CURVE('',#45442,#45444,#25116,.T.);
#60349=EDGE_CURVE('',#45443,#45444,#25117,.T.);
#60350=EDGE_CURVE('',#45443,#45445,#25118,.T.);
#60351=EDGE_CURVE('',#45444,#45446,#25119,.T.);
#60352=EDGE_CURVE('',#45445,#45446,#25120,.T.);
#60353=EDGE_CURVE('',#45445,#45447,#25121,.T.);
#60354=EDGE_CURVE('',#45446,#45448,#25122,.T.);
#60355=EDGE_CURVE('',#45447,#45448,#25123,.T.);
#60356=EDGE_CURVE('',#45447,#45449,#36551,.T.);
#60357=EDGE_CURVE('',#45448,#45450,#36552,.T.);
#60358=EDGE_CURVE('',#45449,#45450,#25124,.T.);
#60359=EDGE_CURVE('',#45449,#45451,#25125,.T.);
#60360=EDGE_CURVE('',#45450,#45452,#25126,.T.);
#60361=EDGE_CURVE('',#45451,#45452,#25127,.T.);
#60362=EDGE_CURVE('',#45451,#45453,#36553,.T.);
#60363=EDGE_CURVE('',#45452,#45454,#36554,.T.);
#60364=EDGE_CURVE('',#45453,#45454,#25128,.T.);
#60365=EDGE_CURVE('',#45453,#45455,#25129,.T.);
#60366=EDGE_CURVE('',#45454,#45456,#25130,.T.);
#60367=EDGE_CURVE('',#45455,#45456,#25131,.T.);
#60368=EDGE_CURVE('',#45455,#45457,#36555,.T.);
#60369=EDGE_CURVE('',#45456,#45458,#36556,.T.);
#60370=EDGE_CURVE('',#45457,#45458,#25132,.T.);
#60371=EDGE_CURVE('',#45457,#45459,#25133,.T.);
#60372=EDGE_CURVE('',#45458,#45460,#25134,.T.);
#60373=EDGE_CURVE('',#45459,#45460,#25135,.T.);
#60374=EDGE_CURVE('',#45459,#45461,#36557,.T.);
#60375=EDGE_CURVE('',#45460,#45462,#36558,.T.);
#60376=EDGE_CURVE('',#45461,#45462,#25136,.T.);
#60377=EDGE_CURVE('',#45461,#45363,#25137,.T.);
#60378=EDGE_CURVE('',#45462,#45365,#25138,.T.);
#60379=EDGE_CURVE('',#45463,#45043,#25139,.T.);
#60380=EDGE_CURVE('',#45464,#45463,#25140,.T.);
#60381=EDGE_CURVE('',#45464,#45045,#25141,.T.);
#60382=EDGE_CURVE('',#45143,#45463,#25142,.T.);
#60383=EDGE_CURVE('',#45144,#45464,#25143,.T.);
#60384=EDGE_CURVE('',#45040,#45465,#25144,.T.);
#60385=EDGE_CURVE('',#45042,#45466,#25145,.T.);
#60386=EDGE_CURVE('',#45466,#45465,#25146,.T.);
#60387=EDGE_CURVE('',#45465,#45117,#25147,.T.);
#60388=EDGE_CURVE('',#45466,#45119,#25148,.T.);
#60389=EDGE_CURVE('',#45467,#45468,#25149,.T.);
#60390=EDGE_CURVE('',#45469,#45467,#25150,.T.);
#60391=EDGE_CURVE('',#45470,#45469,#25151,.T.);
#60392=EDGE_CURVE('',#45470,#45471,#25152,.T.);
#60393=EDGE_CURVE('',#45472,#45471,#25153,.T.);
#60394=EDGE_CURVE('',#45472,#45473,#25154,.T.);
#60395=EDGE_CURVE('',#45473,#45474,#25155,.T.);
#60396=EDGE_CURVE('',#45468,#45474,#25156,.T.);
#60397=EDGE_CURVE('',#45475,#45476,#25157,.T.);
#60398=EDGE_CURVE('',#45468,#45475,#25158,.T.);
#60399=EDGE_CURVE('',#45474,#45476,#25159,.T.);
#60400=EDGE_CURVE('',#45477,#45476,#25160,.T.);
#60401=EDGE_CURVE('',#45473,#45477,#25161,.T.);
#60402=EDGE_CURVE('',#45478,#45477,#25162,.T.);
#60403=EDGE_CURVE('',#45472,#45478,#25163,.T.);
#60404=EDGE_CURVE('',#45478,#45479,#25164,.T.);
#60405=EDGE_CURVE('',#45471,#45479,#25165,.T.);
#60406=EDGE_CURVE('',#45480,#45479,#25166,.T.);
#60407=EDGE_CURVE('',#45470,#45480,#25167,.T.);
#60408=EDGE_CURVE('',#45480,#45481,#25168,.T.);
#60409=EDGE_CURVE('',#45469,#45481,#25169,.T.);
#60410=EDGE_CURVE('',#45481,#45482,#25170,.T.);
#60411=EDGE_CURVE('',#45467,#45482,#25171,.T.);
#60412=EDGE_CURVE('',#45482,#45475,#25172,.T.);
#60413=EDGE_CURVE('',#45483,#45484,#25173,.T.);
#60414=EDGE_CURVE('',#45485,#45483,#25174,.T.);
#60415=EDGE_CURVE('',#45485,#45486,#25175,.T.);
#60416=EDGE_CURVE('',#45486,#45484,#25176,.T.);
#60417=EDGE_CURVE('',#45484,#45487,#25177,.T.);
#60418=EDGE_CURVE('',#45486,#45488,#25178,.T.);
#60419=EDGE_CURVE('',#45488,#45487,#25179,.T.);
#60420=EDGE_CURVE('',#45487,#45489,#25180,.T.);
#60421=EDGE_CURVE('',#45488,#45490,#25181,.T.);
#60422=EDGE_CURVE('',#45490,#45489,#25182,.T.);
#60423=EDGE_CURVE('',#45489,#45483,#25183,.T.);
#60424=EDGE_CURVE('',#45490,#45485,#25184,.T.);
#88025=ORIENTED_EDGE('',*,*,#59291,.T.);
#88026=ORIENTED_EDGE('',*,*,#59292,.T.);
#88027=ORIENTED_EDGE('',*,*,#59293,.F.);
#88028=ORIENTED_EDGE('',*,*,#59294,.F.);
#88029=ORIENTED_EDGE('',*,*,#59295,.T.);
#88030=ORIENTED_EDGE('',*,*,#59296,.T.);
#88031=ORIENTED_EDGE('',*,*,#59297,.T.);
#88032=ORIENTED_EDGE('',*,*,#59298,.T.);
#88033=ORIENTED_EDGE('',*,*,#59299,.T.);
#88034=ORIENTED_EDGE('',*,*,#59300,.T.);
#88035=ORIENTED_EDGE('',*,*,#59301,.T.);
#88036=ORIENTED_EDGE('',*,*,#59302,.T.);
#88037=ORIENTED_EDGE('',*,*,#59303,.T.);
#88038=ORIENTED_EDGE('',*,*,#59304,.T.);
#88039=ORIENTED_EDGE('',*,*,#59305,.T.);
#88040=ORIENTED_EDGE('',*,*,#59306,.T.);
#88041=ORIENTED_EDGE('',*,*,#59307,.T.);
#88042=ORIENTED_EDGE('',*,*,#59308,.T.);
#88043=ORIENTED_EDGE('',*,*,#59293,.T.);
#88044=ORIENTED_EDGE('',*,*,#59309,.T.);
#88045=ORIENTED_EDGE('',*,*,#59292,.F.);
#88046=ORIENTED_EDGE('',*,*,#59310,.T.);
#88047=ORIENTED_EDGE('',*,*,#59311,.T.);
#88048=ORIENTED_EDGE('',*,*,#59309,.F.);
#88049=ORIENTED_EDGE('',*,*,#59312,.F.);
#88050=ORIENTED_EDGE('',*,*,#59313,.T.);
#88051=ORIENTED_EDGE('',*,*,#59294,.T.);
#88052=ORIENTED_EDGE('',*,*,#59308,.F.);
#88053=ORIENTED_EDGE('',*,*,#59314,.F.);
#88054=ORIENTED_EDGE('',*,*,#59315,.T.);
#88055=ORIENTED_EDGE('',*,*,#59312,.T.);
#88056=ORIENTED_EDGE('',*,*,#59307,.F.);
#88057=ORIENTED_EDGE('',*,*,#59316,.F.);
#88058=ORIENTED_EDGE('',*,*,#59317,.T.);
#88059=ORIENTED_EDGE('',*,*,#59314,.T.);
#88060=ORIENTED_EDGE('',*,*,#59306,.F.);
#88061=ORIENTED_EDGE('',*,*,#59318,.F.);
#88062=ORIENTED_EDGE('',*,*,#59319,.T.);
#88063=ORIENTED_EDGE('',*,*,#59316,.T.);
#88064=ORIENTED_EDGE('',*,*,#59305,.F.);
#88065=ORIENTED_EDGE('',*,*,#59320,.F.);
#88066=ORIENTED_EDGE('',*,*,#59321,.T.);
#88067=ORIENTED_EDGE('',*,*,#59318,.T.);
#88068=ORIENTED_EDGE('',*,*,#59304,.F.);
#88069=ORIENTED_EDGE('',*,*,#59322,.F.);
#88070=ORIENTED_EDGE('',*,*,#59323,.T.);
#88071=ORIENTED_EDGE('',*,*,#59320,.T.);
#88072=ORIENTED_EDGE('',*,*,#59303,.F.);
#88073=ORIENTED_EDGE('',*,*,#59324,.F.);
#88074=ORIENTED_EDGE('',*,*,#59325,.T.);
#88075=ORIENTED_EDGE('',*,*,#59322,.T.);
#88076=ORIENTED_EDGE('',*,*,#59302,.F.);
#88077=ORIENTED_EDGE('',*,*,#59326,.F.);
#88078=ORIENTED_EDGE('',*,*,#59327,.T.);
#88079=ORIENTED_EDGE('',*,*,#59324,.T.);
#88080=ORIENTED_EDGE('',*,*,#59301,.F.);
#88081=ORIENTED_EDGE('',*,*,#59328,.F.);
#88082=ORIENTED_EDGE('',*,*,#59329,.T.);
#88083=ORIENTED_EDGE('',*,*,#59326,.T.);
#88084=ORIENTED_EDGE('',*,*,#59300,.F.);
#88085=ORIENTED_EDGE('',*,*,#59330,.F.);
#88086=ORIENTED_EDGE('',*,*,#59331,.T.);
#88087=ORIENTED_EDGE('',*,*,#59328,.T.);
#88088=ORIENTED_EDGE('',*,*,#59299,.F.);
#88089=ORIENTED_EDGE('',*,*,#59332,.F.);
#88090=ORIENTED_EDGE('',*,*,#59333,.T.);
#88091=ORIENTED_EDGE('',*,*,#59330,.T.);
#88092=ORIENTED_EDGE('',*,*,#59298,.F.);
#88093=ORIENTED_EDGE('',*,*,#59334,.F.);
#88094=ORIENTED_EDGE('',*,*,#59335,.T.);
#88095=ORIENTED_EDGE('',*,*,#59332,.T.);
#88096=ORIENTED_EDGE('',*,*,#59297,.F.);
#88097=ORIENTED_EDGE('',*,*,#59336,.F.);
#88098=ORIENTED_EDGE('',*,*,#59337,.T.);
#88099=ORIENTED_EDGE('',*,*,#59334,.T.);
#88100=ORIENTED_EDGE('',*,*,#59296,.F.);
#88101=ORIENTED_EDGE('',*,*,#59311,.F.);
#88102=ORIENTED_EDGE('',*,*,#59338,.T.);
#88103=ORIENTED_EDGE('',*,*,#59336,.T.);
#88104=ORIENTED_EDGE('',*,*,#59295,.F.);
#88105=ORIENTED_EDGE('',*,*,#59338,.F.);
#88106=ORIENTED_EDGE('',*,*,#59310,.F.);
#88107=ORIENTED_EDGE('',*,*,#59291,.F.);
#88108=ORIENTED_EDGE('',*,*,#59313,.F.);
#88109=ORIENTED_EDGE('',*,*,#59315,.F.);
#88110=ORIENTED_EDGE('',*,*,#59317,.F.);
#88111=ORIENTED_EDGE('',*,*,#59319,.F.);
#88112=ORIENTED_EDGE('',*,*,#59321,.F.);
#88113=ORIENTED_EDGE('',*,*,#59323,.F.);
#88114=ORIENTED_EDGE('',*,*,#59325,.F.);
#88115=ORIENTED_EDGE('',*,*,#59327,.F.);
#88116=ORIENTED_EDGE('',*,*,#59329,.F.);
#88117=ORIENTED_EDGE('',*,*,#59331,.F.);
#88118=ORIENTED_EDGE('',*,*,#59333,.F.);
#88119=ORIENTED_EDGE('',*,*,#59335,.F.);
#88120=ORIENTED_EDGE('',*,*,#59337,.F.);
#88121=ORIENTED_EDGE('',*,*,#59339,.T.);
#88122=ORIENTED_EDGE('',*,*,#59340,.T.);
#88123=ORIENTED_EDGE('',*,*,#59341,.T.);
#88124=ORIENTED_EDGE('',*,*,#59342,.T.);
#88125=ORIENTED_EDGE('',*,*,#59343,.T.);
#88126=ORIENTED_EDGE('',*,*,#59344,.T.);
#88127=ORIENTED_EDGE('',*,*,#59345,.T.);
#88128=ORIENTED_EDGE('',*,*,#59346,.T.);
#88129=ORIENTED_EDGE('',*,*,#59347,.F.);
#88130=ORIENTED_EDGE('',*,*,#59348,.T.);
#88131=ORIENTED_EDGE('',*,*,#59349,.T.);
#88132=ORIENTED_EDGE('',*,*,#59346,.F.);
#88133=ORIENTED_EDGE('',*,*,#59350,.F.);
#88134=ORIENTED_EDGE('',*,*,#59351,.T.);
#88135=ORIENTED_EDGE('',*,*,#59347,.T.);
#88136=ORIENTED_EDGE('',*,*,#59345,.F.);
#88137=ORIENTED_EDGE('',*,*,#59352,.F.);
#88138=ORIENTED_EDGE('',*,*,#59353,.T.);
#88139=ORIENTED_EDGE('',*,*,#59350,.T.);
#88140=ORIENTED_EDGE('',*,*,#59344,.F.);
#88141=ORIENTED_EDGE('',*,*,#59354,.F.);
#88142=ORIENTED_EDGE('',*,*,#59355,.T.);
#88143=ORIENTED_EDGE('',*,*,#59352,.T.);
#88144=ORIENTED_EDGE('',*,*,#59343,.F.);
#88145=ORIENTED_EDGE('',*,*,#59356,.F.);
#88146=ORIENTED_EDGE('',*,*,#59357,.T.);
#88147=ORIENTED_EDGE('',*,*,#59354,.T.);
#88148=ORIENTED_EDGE('',*,*,#59342,.F.);
#88149=ORIENTED_EDGE('',*,*,#59358,.F.);
#88150=ORIENTED_EDGE('',*,*,#59359,.T.);
#88151=ORIENTED_EDGE('',*,*,#59356,.T.);
#88152=ORIENTED_EDGE('',*,*,#59341,.F.);
#88153=ORIENTED_EDGE('',*,*,#59360,.F.);
#88154=ORIENTED_EDGE('',*,*,#59361,.T.);
#88155=ORIENTED_EDGE('',*,*,#59358,.T.);
#88156=ORIENTED_EDGE('',*,*,#59340,.F.);
#88157=ORIENTED_EDGE('',*,*,#59349,.F.);
#88158=ORIENTED_EDGE('',*,*,#59362,.T.);
#88159=ORIENTED_EDGE('',*,*,#59360,.T.);
#88160=ORIENTED_EDGE('',*,*,#59339,.F.);
#88161=ORIENTED_EDGE('',*,*,#59362,.F.);
#88162=ORIENTED_EDGE('',*,*,#59348,.F.);
#88163=ORIENTED_EDGE('',*,*,#59351,.F.);
#88164=ORIENTED_EDGE('',*,*,#59353,.F.);
#88165=ORIENTED_EDGE('',*,*,#59355,.F.);
#88166=ORIENTED_EDGE('',*,*,#59357,.F.);
#88167=ORIENTED_EDGE('',*,*,#59359,.F.);
#88168=ORIENTED_EDGE('',*,*,#59361,.F.);
#88169=ORIENTED_EDGE('',*,*,#59363,.T.);
#88170=ORIENTED_EDGE('',*,*,#59364,.T.);
#88171=ORIENTED_EDGE('',*,*,#59365,.T.);
#88172=ORIENTED_EDGE('',*,*,#59366,.T.);
#88173=ORIENTED_EDGE('',*,*,#59367,.T.);
#88174=ORIENTED_EDGE('',*,*,#59368,.T.);
#88175=ORIENTED_EDGE('',*,*,#59369,.T.);
#88176=ORIENTED_EDGE('',*,*,#59370,.T.);
#88177=ORIENTED_EDGE('',*,*,#59371,.T.);
#88178=ORIENTED_EDGE('',*,*,#59372,.T.);
#88179=ORIENTED_EDGE('',*,*,#59373,.T.);
#88180=ORIENTED_EDGE('',*,*,#59374,.T.);
#88181=ORIENTED_EDGE('',*,*,#59375,.T.);
#88182=ORIENTED_EDGE('',*,*,#59376,.T.);
#88183=ORIENTED_EDGE('',*,*,#59377,.T.);
#88184=ORIENTED_EDGE('',*,*,#59378,.T.);
#88185=ORIENTED_EDGE('',*,*,#59379,.T.);
#88186=ORIENTED_EDGE('',*,*,#59380,.T.);
#88187=ORIENTED_EDGE('',*,*,#59381,.T.);
#88188=ORIENTED_EDGE('',*,*,#59382,.T.);
#88189=ORIENTED_EDGE('',*,*,#59383,.T.);
#88190=ORIENTED_EDGE('',*,*,#59384,.T.);
#88191=ORIENTED_EDGE('',*,*,#59385,.T.);
#88192=ORIENTED_EDGE('',*,*,#59386,.T.);
#88193=ORIENTED_EDGE('',*,*,#59387,.T.);
#88194=ORIENTED_EDGE('',*,*,#59388,.T.);
#88195=ORIENTED_EDGE('',*,*,#59389,.T.);
#88196=ORIENTED_EDGE('',*,*,#59390,.T.);
#88197=ORIENTED_EDGE('',*,*,#59391,.T.);
#88198=ORIENTED_EDGE('',*,*,#59392,.T.);
#88199=ORIENTED_EDGE('',*,*,#59393,.T.);
#88200=ORIENTED_EDGE('',*,*,#59394,.T.);
#88201=ORIENTED_EDGE('',*,*,#59395,.T.);
#88202=ORIENTED_EDGE('',*,*,#59396,.T.);
#88203=ORIENTED_EDGE('',*,*,#59397,.T.);
#88204=ORIENTED_EDGE('',*,*,#59398,.T.);
#88205=ORIENTED_EDGE('',*,*,#59399,.T.);
#88206=ORIENTED_EDGE('',*,*,#59400,.T.);
#88207=ORIENTED_EDGE('',*,*,#59401,.T.);
#88208=ORIENTED_EDGE('',*,*,#59402,.T.);
#88209=ORIENTED_EDGE('',*,*,#59403,.T.);
#88210=ORIENTED_EDGE('',*,*,#59404,.T.);
#88211=ORIENTED_EDGE('',*,*,#59405,.T.);
#88212=ORIENTED_EDGE('',*,*,#59406,.T.);
#88213=ORIENTED_EDGE('',*,*,#59407,.T.);
#88214=ORIENTED_EDGE('',*,*,#59408,.T.);
#88215=ORIENTED_EDGE('',*,*,#59409,.T.);
#88216=ORIENTED_EDGE('',*,*,#59410,.T.);
#88217=ORIENTED_EDGE('',*,*,#59411,.T.);
#88218=ORIENTED_EDGE('',*,*,#59412,.T.);
#88219=ORIENTED_EDGE('',*,*,#59413,.T.);
#88220=ORIENTED_EDGE('',*,*,#59414,.T.);
#88221=ORIENTED_EDGE('',*,*,#59415,.T.);
#88222=ORIENTED_EDGE('',*,*,#59416,.T.);
#88223=ORIENTED_EDGE('',*,*,#59417,.T.);
#88224=ORIENTED_EDGE('',*,*,#59418,.T.);
#88225=ORIENTED_EDGE('',*,*,#59419,.F.);
#88226=ORIENTED_EDGE('',*,*,#59420,.F.);
#88227=ORIENTED_EDGE('',*,*,#59421,.F.);
#88228=ORIENTED_EDGE('',*,*,#59422,.F.);
#88229=ORIENTED_EDGE('',*,*,#59423,.F.);
#88230=ORIENTED_EDGE('',*,*,#59424,.F.);
#88231=ORIENTED_EDGE('',*,*,#59425,.F.);
#88232=ORIENTED_EDGE('',*,*,#59426,.F.);
#88233=ORIENTED_EDGE('',*,*,#59427,.F.);
#88234=ORIENTED_EDGE('',*,*,#59428,.F.);
#88235=ORIENTED_EDGE('',*,*,#59429,.F.);
#88236=ORIENTED_EDGE('',*,*,#59430,.F.);
#88237=ORIENTED_EDGE('',*,*,#59431,.F.);
#88238=ORIENTED_EDGE('',*,*,#59432,.F.);
#88239=ORIENTED_EDGE('',*,*,#59433,.F.);
#88240=ORIENTED_EDGE('',*,*,#59434,.F.);
#88241=ORIENTED_EDGE('',*,*,#59435,.F.);
#88242=ORIENTED_EDGE('',*,*,#59436,.F.);
#88243=ORIENTED_EDGE('',*,*,#59437,.F.);
#88244=ORIENTED_EDGE('',*,*,#59438,.F.);
#88245=ORIENTED_EDGE('',*,*,#59439,.F.);
#88246=ORIENTED_EDGE('',*,*,#59440,.F.);
#88247=ORIENTED_EDGE('',*,*,#59441,.F.);
#88248=ORIENTED_EDGE('',*,*,#59442,.F.);
#88249=ORIENTED_EDGE('',*,*,#59443,.F.);
#88250=ORIENTED_EDGE('',*,*,#59444,.F.);
#88251=ORIENTED_EDGE('',*,*,#59445,.F.);
#88252=ORIENTED_EDGE('',*,*,#59446,.F.);
#88253=ORIENTED_EDGE('',*,*,#59447,.F.);
#88254=ORIENTED_EDGE('',*,*,#59448,.F.);
#88255=ORIENTED_EDGE('',*,*,#59449,.F.);
#88256=ORIENTED_EDGE('',*,*,#59450,.F.);
#88257=ORIENTED_EDGE('',*,*,#59451,.F.);
#88258=ORIENTED_EDGE('',*,*,#59452,.F.);
#88259=ORIENTED_EDGE('',*,*,#59453,.F.);
#88260=ORIENTED_EDGE('',*,*,#59454,.F.);
#88261=ORIENTED_EDGE('',*,*,#59455,.F.);
#88262=ORIENTED_EDGE('',*,*,#59456,.F.);
#88263=ORIENTED_EDGE('',*,*,#59457,.F.);
#88264=ORIENTED_EDGE('',*,*,#59458,.F.);
#88265=ORIENTED_EDGE('',*,*,#59459,.F.);
#88266=ORIENTED_EDGE('',*,*,#59460,.F.);
#88267=ORIENTED_EDGE('',*,*,#59461,.F.);
#88268=ORIENTED_EDGE('',*,*,#59462,.F.);
#88269=ORIENTED_EDGE('',*,*,#59463,.F.);
#88270=ORIENTED_EDGE('',*,*,#59464,.F.);
#88271=ORIENTED_EDGE('',*,*,#59465,.F.);
#88272=ORIENTED_EDGE('',*,*,#59466,.F.);
#88273=ORIENTED_EDGE('',*,*,#59467,.F.);
#88274=ORIENTED_EDGE('',*,*,#59468,.F.);
#88275=ORIENTED_EDGE('',*,*,#59469,.F.);
#88276=ORIENTED_EDGE('',*,*,#59470,.F.);
#88277=ORIENTED_EDGE('',*,*,#59471,.F.);
#88278=ORIENTED_EDGE('',*,*,#59472,.F.);
#88279=ORIENTED_EDGE('',*,*,#59473,.F.);
#88280=ORIENTED_EDGE('',*,*,#59474,.F.);
#88281=ORIENTED_EDGE('',*,*,#59363,.F.);
#88282=ORIENTED_EDGE('',*,*,#59475,.T.);
#88283=ORIENTED_EDGE('',*,*,#59421,.T.);
#88284=ORIENTED_EDGE('',*,*,#59476,.F.);
#88285=ORIENTED_EDGE('',*,*,#59418,.F.);
#88286=ORIENTED_EDGE('',*,*,#59477,.T.);
#88287=ORIENTED_EDGE('',*,*,#59422,.T.);
#88288=ORIENTED_EDGE('',*,*,#59475,.F.);
#88289=ORIENTED_EDGE('',*,*,#59417,.F.);
#88290=ORIENTED_EDGE('',*,*,#59478,.T.);
#88291=ORIENTED_EDGE('',*,*,#59423,.T.);
#88292=ORIENTED_EDGE('',*,*,#59477,.F.);
#88293=ORIENTED_EDGE('',*,*,#59416,.F.);
#88294=ORIENTED_EDGE('',*,*,#59479,.T.);
#88295=ORIENTED_EDGE('',*,*,#59424,.T.);
#88296=ORIENTED_EDGE('',*,*,#59478,.F.);
#88297=ORIENTED_EDGE('',*,*,#59415,.F.);
#88298=ORIENTED_EDGE('',*,*,#59480,.T.);
#88299=ORIENTED_EDGE('',*,*,#59425,.T.);
#88300=ORIENTED_EDGE('',*,*,#59479,.F.);
#88301=ORIENTED_EDGE('',*,*,#59414,.F.);
#88302=ORIENTED_EDGE('',*,*,#59481,.T.);
#88303=ORIENTED_EDGE('',*,*,#59426,.T.);
#88304=ORIENTED_EDGE('',*,*,#59480,.F.);
#88305=ORIENTED_EDGE('',*,*,#59413,.F.);
#88306=ORIENTED_EDGE('',*,*,#59482,.T.);
#88307=ORIENTED_EDGE('',*,*,#59427,.T.);
#88308=ORIENTED_EDGE('',*,*,#59481,.F.);
#88309=ORIENTED_EDGE('',*,*,#59412,.F.);
#88310=ORIENTED_EDGE('',*,*,#59483,.T.);
#88311=ORIENTED_EDGE('',*,*,#59428,.T.);
#88312=ORIENTED_EDGE('',*,*,#59482,.F.);
#88313=ORIENTED_EDGE('',*,*,#59411,.F.);
#88314=ORIENTED_EDGE('',*,*,#59484,.T.);
#88315=ORIENTED_EDGE('',*,*,#59429,.T.);
#88316=ORIENTED_EDGE('',*,*,#59483,.F.);
#88317=ORIENTED_EDGE('',*,*,#59410,.F.);
#88318=ORIENTED_EDGE('',*,*,#59485,.T.);
#88319=ORIENTED_EDGE('',*,*,#59430,.T.);
#88320=ORIENTED_EDGE('',*,*,#59484,.F.);
#88321=ORIENTED_EDGE('',*,*,#59409,.F.);
#88322=ORIENTED_EDGE('',*,*,#59486,.T.);
#88323=ORIENTED_EDGE('',*,*,#59431,.T.);
#88324=ORIENTED_EDGE('',*,*,#59485,.F.);
#88325=ORIENTED_EDGE('',*,*,#59408,.F.);
#88326=ORIENTED_EDGE('',*,*,#59487,.T.);
#88327=ORIENTED_EDGE('',*,*,#59432,.T.);
#88328=ORIENTED_EDGE('',*,*,#59486,.F.);
#88329=ORIENTED_EDGE('',*,*,#59407,.F.);
#88330=ORIENTED_EDGE('',*,*,#59488,.T.);
#88331=ORIENTED_EDGE('',*,*,#59433,.T.);
#88332=ORIENTED_EDGE('',*,*,#59487,.F.);
#88333=ORIENTED_EDGE('',*,*,#59406,.F.);
#88334=ORIENTED_EDGE('',*,*,#59489,.T.);
#88335=ORIENTED_EDGE('',*,*,#59434,.T.);
#88336=ORIENTED_EDGE('',*,*,#59488,.F.);
#88337=ORIENTED_EDGE('',*,*,#59405,.F.);
#88338=ORIENTED_EDGE('',*,*,#59490,.T.);
#88339=ORIENTED_EDGE('',*,*,#59435,.T.);
#88340=ORIENTED_EDGE('',*,*,#59489,.F.);
#88341=ORIENTED_EDGE('',*,*,#59404,.F.);
#88342=ORIENTED_EDGE('',*,*,#59491,.T.);
#88343=ORIENTED_EDGE('',*,*,#59436,.T.);
#88344=ORIENTED_EDGE('',*,*,#59490,.F.);
#88345=ORIENTED_EDGE('',*,*,#59403,.F.);
#88346=ORIENTED_EDGE('',*,*,#59492,.T.);
#88347=ORIENTED_EDGE('',*,*,#59437,.T.);
#88348=ORIENTED_EDGE('',*,*,#59491,.F.);
#88349=ORIENTED_EDGE('',*,*,#59402,.F.);
#88350=ORIENTED_EDGE('',*,*,#59493,.T.);
#88351=ORIENTED_EDGE('',*,*,#59438,.T.);
#88352=ORIENTED_EDGE('',*,*,#59492,.F.);
#88353=ORIENTED_EDGE('',*,*,#59401,.F.);
#88354=ORIENTED_EDGE('',*,*,#59494,.T.);
#88355=ORIENTED_EDGE('',*,*,#59439,.T.);
#88356=ORIENTED_EDGE('',*,*,#59493,.F.);
#88357=ORIENTED_EDGE('',*,*,#59400,.F.);
#88358=ORIENTED_EDGE('',*,*,#59495,.T.);
#88359=ORIENTED_EDGE('',*,*,#59440,.T.);
#88360=ORIENTED_EDGE('',*,*,#59494,.F.);
#88361=ORIENTED_EDGE('',*,*,#59399,.F.);
#88362=ORIENTED_EDGE('',*,*,#59496,.T.);
#88363=ORIENTED_EDGE('',*,*,#59441,.T.);
#88364=ORIENTED_EDGE('',*,*,#59495,.F.);
#88365=ORIENTED_EDGE('',*,*,#59398,.F.);
#88366=ORIENTED_EDGE('',*,*,#59497,.T.);
#88367=ORIENTED_EDGE('',*,*,#59442,.T.);
#88368=ORIENTED_EDGE('',*,*,#59496,.F.);
#88369=ORIENTED_EDGE('',*,*,#59397,.F.);
#88370=ORIENTED_EDGE('',*,*,#59498,.T.);
#88371=ORIENTED_EDGE('',*,*,#59443,.T.);
#88372=ORIENTED_EDGE('',*,*,#59497,.F.);
#88373=ORIENTED_EDGE('',*,*,#59396,.F.);
#88374=ORIENTED_EDGE('',*,*,#59499,.T.);
#88375=ORIENTED_EDGE('',*,*,#59444,.T.);
#88376=ORIENTED_EDGE('',*,*,#59498,.F.);
#88377=ORIENTED_EDGE('',*,*,#59395,.F.);
#88378=ORIENTED_EDGE('',*,*,#59500,.T.);
#88379=ORIENTED_EDGE('',*,*,#59445,.T.);
#88380=ORIENTED_EDGE('',*,*,#59499,.F.);
#88381=ORIENTED_EDGE('',*,*,#59394,.F.);
#88382=ORIENTED_EDGE('',*,*,#59501,.T.);
#88383=ORIENTED_EDGE('',*,*,#59446,.T.);
#88384=ORIENTED_EDGE('',*,*,#59500,.F.);
#88385=ORIENTED_EDGE('',*,*,#59393,.F.);
#88386=ORIENTED_EDGE('',*,*,#59502,.T.);
#88387=ORIENTED_EDGE('',*,*,#59447,.T.);
#88388=ORIENTED_EDGE('',*,*,#59501,.F.);
#88389=ORIENTED_EDGE('',*,*,#59392,.F.);
#88390=ORIENTED_EDGE('',*,*,#59503,.T.);
#88391=ORIENTED_EDGE('',*,*,#59448,.T.);
#88392=ORIENTED_EDGE('',*,*,#59502,.F.);
#88393=ORIENTED_EDGE('',*,*,#59391,.F.);
#88394=ORIENTED_EDGE('',*,*,#59504,.T.);
#88395=ORIENTED_EDGE('',*,*,#59449,.T.);
#88396=ORIENTED_EDGE('',*,*,#59503,.F.);
#88397=ORIENTED_EDGE('',*,*,#59390,.F.);
#88398=ORIENTED_EDGE('',*,*,#59505,.T.);
#88399=ORIENTED_EDGE('',*,*,#59450,.T.);
#88400=ORIENTED_EDGE('',*,*,#59504,.F.);
#88401=ORIENTED_EDGE('',*,*,#59389,.F.);
#88402=ORIENTED_EDGE('',*,*,#59506,.T.);
#88403=ORIENTED_EDGE('',*,*,#59451,.T.);
#88404=ORIENTED_EDGE('',*,*,#59505,.F.);
#88405=ORIENTED_EDGE('',*,*,#59388,.F.);
#88406=ORIENTED_EDGE('',*,*,#59507,.T.);
#88407=ORIENTED_EDGE('',*,*,#59452,.T.);
#88408=ORIENTED_EDGE('',*,*,#59506,.F.);
#88409=ORIENTED_EDGE('',*,*,#59387,.F.);
#88410=ORIENTED_EDGE('',*,*,#59508,.T.);
#88411=ORIENTED_EDGE('',*,*,#59453,.T.);
#88412=ORIENTED_EDGE('',*,*,#59507,.F.);
#88413=ORIENTED_EDGE('',*,*,#59386,.F.);
#88414=ORIENTED_EDGE('',*,*,#59509,.T.);
#88415=ORIENTED_EDGE('',*,*,#59454,.T.);
#88416=ORIENTED_EDGE('',*,*,#59508,.F.);
#88417=ORIENTED_EDGE('',*,*,#59385,.F.);
#88418=ORIENTED_EDGE('',*,*,#59510,.T.);
#88419=ORIENTED_EDGE('',*,*,#59455,.T.);
#88420=ORIENTED_EDGE('',*,*,#59509,.F.);
#88421=ORIENTED_EDGE('',*,*,#59384,.F.);
#88422=ORIENTED_EDGE('',*,*,#59511,.T.);
#88423=ORIENTED_EDGE('',*,*,#59456,.T.);
#88424=ORIENTED_EDGE('',*,*,#59510,.F.);
#88425=ORIENTED_EDGE('',*,*,#59383,.F.);
#88426=ORIENTED_EDGE('',*,*,#59512,.T.);
#88427=ORIENTED_EDGE('',*,*,#59457,.T.);
#88428=ORIENTED_EDGE('',*,*,#59511,.F.);
#88429=ORIENTED_EDGE('',*,*,#59382,.F.);
#88430=ORIENTED_EDGE('',*,*,#59513,.T.);
#88431=ORIENTED_EDGE('',*,*,#59458,.T.);
#88432=ORIENTED_EDGE('',*,*,#59512,.F.);
#88433=ORIENTED_EDGE('',*,*,#59381,.F.);
#88434=ORIENTED_EDGE('',*,*,#59514,.T.);
#88435=ORIENTED_EDGE('',*,*,#59459,.T.);
#88436=ORIENTED_EDGE('',*,*,#59513,.F.);
#88437=ORIENTED_EDGE('',*,*,#59380,.F.);
#88438=ORIENTED_EDGE('',*,*,#59515,.T.);
#88439=ORIENTED_EDGE('',*,*,#59460,.T.);
#88440=ORIENTED_EDGE('',*,*,#59514,.F.);
#88441=ORIENTED_EDGE('',*,*,#59379,.F.);
#88442=ORIENTED_EDGE('',*,*,#59516,.T.);
#88443=ORIENTED_EDGE('',*,*,#59461,.T.);
#88444=ORIENTED_EDGE('',*,*,#59515,.F.);
#88445=ORIENTED_EDGE('',*,*,#59378,.F.);
#88446=ORIENTED_EDGE('',*,*,#59517,.T.);
#88447=ORIENTED_EDGE('',*,*,#59462,.T.);
#88448=ORIENTED_EDGE('',*,*,#59516,.F.);
#88449=ORIENTED_EDGE('',*,*,#59377,.F.);
#88450=ORIENTED_EDGE('',*,*,#59518,.T.);
#88451=ORIENTED_EDGE('',*,*,#59463,.T.);
#88452=ORIENTED_EDGE('',*,*,#59517,.F.);
#88453=ORIENTED_EDGE('',*,*,#59376,.F.);
#88454=ORIENTED_EDGE('',*,*,#59519,.T.);
#88455=ORIENTED_EDGE('',*,*,#59464,.T.);
#88456=ORIENTED_EDGE('',*,*,#59518,.F.);
#88457=ORIENTED_EDGE('',*,*,#59375,.F.);
#88458=ORIENTED_EDGE('',*,*,#59520,.T.);
#88459=ORIENTED_EDGE('',*,*,#59465,.T.);
#88460=ORIENTED_EDGE('',*,*,#59519,.F.);
#88461=ORIENTED_EDGE('',*,*,#59374,.F.);
#88462=ORIENTED_EDGE('',*,*,#59521,.T.);
#88463=ORIENTED_EDGE('',*,*,#59466,.T.);
#88464=ORIENTED_EDGE('',*,*,#59520,.F.);
#88465=ORIENTED_EDGE('',*,*,#59373,.F.);
#88466=ORIENTED_EDGE('',*,*,#59522,.T.);
#88467=ORIENTED_EDGE('',*,*,#59467,.T.);
#88468=ORIENTED_EDGE('',*,*,#59521,.F.);
#88469=ORIENTED_EDGE('',*,*,#59372,.F.);
#88470=ORIENTED_EDGE('',*,*,#59523,.T.);
#88471=ORIENTED_EDGE('',*,*,#59468,.T.);
#88472=ORIENTED_EDGE('',*,*,#59522,.F.);
#88473=ORIENTED_EDGE('',*,*,#59371,.F.);
#88474=ORIENTED_EDGE('',*,*,#59524,.T.);
#88475=ORIENTED_EDGE('',*,*,#59469,.T.);
#88476=ORIENTED_EDGE('',*,*,#59523,.F.);
#88477=ORIENTED_EDGE('',*,*,#59370,.F.);
#88478=ORIENTED_EDGE('',*,*,#59525,.T.);
#88479=ORIENTED_EDGE('',*,*,#59470,.T.);
#88480=ORIENTED_EDGE('',*,*,#59524,.F.);
#88481=ORIENTED_EDGE('',*,*,#59369,.F.);
#88482=ORIENTED_EDGE('',*,*,#59526,.T.);
#88483=ORIENTED_EDGE('',*,*,#59471,.T.);
#88484=ORIENTED_EDGE('',*,*,#59525,.F.);
#88485=ORIENTED_EDGE('',*,*,#59368,.F.);
#88486=ORIENTED_EDGE('',*,*,#59527,.T.);
#88487=ORIENTED_EDGE('',*,*,#59472,.T.);
#88488=ORIENTED_EDGE('',*,*,#59526,.F.);
#88489=ORIENTED_EDGE('',*,*,#59367,.F.);
#88490=ORIENTED_EDGE('',*,*,#59528,.T.);
#88491=ORIENTED_EDGE('',*,*,#59473,.T.);
#88492=ORIENTED_EDGE('',*,*,#59527,.F.);
#88493=ORIENTED_EDGE('',*,*,#59366,.F.);
#88494=ORIENTED_EDGE('',*,*,#59529,.T.);
#88495=ORIENTED_EDGE('',*,*,#59474,.T.);
#88496=ORIENTED_EDGE('',*,*,#59528,.F.);
#88497=ORIENTED_EDGE('',*,*,#59365,.F.);
#88498=ORIENTED_EDGE('',*,*,#59530,.T.);
#88499=ORIENTED_EDGE('',*,*,#59419,.T.);
#88500=ORIENTED_EDGE('',*,*,#59529,.F.);
#88501=ORIENTED_EDGE('',*,*,#59364,.F.);
#88502=ORIENTED_EDGE('',*,*,#59476,.T.);
#88503=ORIENTED_EDGE('',*,*,#59420,.T.);
#88504=ORIENTED_EDGE('',*,*,#59530,.F.);
#88505=ORIENTED_EDGE('',*,*,#59531,.T.);
#88506=ORIENTED_EDGE('',*,*,#59532,.T.);
#88507=ORIENTED_EDGE('',*,*,#59533,.F.);
#88508=ORIENTED_EDGE('',*,*,#59534,.F.);
#88509=ORIENTED_EDGE('',*,*,#59535,.T.);
#88510=ORIENTED_EDGE('',*,*,#59536,.T.);
#88511=ORIENTED_EDGE('',*,*,#59537,.T.);
#88512=ORIENTED_EDGE('',*,*,#59538,.T.);
#88513=ORIENTED_EDGE('',*,*,#59539,.T.);
#88514=ORIENTED_EDGE('',*,*,#59540,.T.);
#88515=ORIENTED_EDGE('',*,*,#59533,.T.);
#88516=ORIENTED_EDGE('',*,*,#59541,.T.);
#88517=ORIENTED_EDGE('',*,*,#59542,.T.);
#88518=ORIENTED_EDGE('',*,*,#59543,.T.);
#88519=ORIENTED_EDGE('',*,*,#59544,.T.);
#88520=ORIENTED_EDGE('',*,*,#59545,.T.);
#88521=ORIENTED_EDGE('',*,*,#59546,.T.);
#88522=ORIENTED_EDGE('',*,*,#59547,.T.);
#88523=ORIENTED_EDGE('',*,*,#59548,.T.);
#88524=ORIENTED_EDGE('',*,*,#59549,.T.);
#88525=ORIENTED_EDGE('',*,*,#59550,.F.);
#88526=ORIENTED_EDGE('',*,*,#59551,.T.);
#88527=ORIENTED_EDGE('',*,*,#59552,.T.);
#88528=ORIENTED_EDGE('',*,*,#59549,.F.);
#88529=ORIENTED_EDGE('',*,*,#59553,.F.);
#88530=ORIENTED_EDGE('',*,*,#59554,.T.);
#88531=ORIENTED_EDGE('',*,*,#59550,.T.);
#88532=ORIENTED_EDGE('',*,*,#59548,.F.);
#88533=ORIENTED_EDGE('',*,*,#59555,.F.);
#88534=ORIENTED_EDGE('',*,*,#59556,.T.);
#88535=ORIENTED_EDGE('',*,*,#59553,.T.);
#88536=ORIENTED_EDGE('',*,*,#59547,.F.);
#88537=ORIENTED_EDGE('',*,*,#59557,.F.);
#88538=ORIENTED_EDGE('',*,*,#59558,.T.);
#88539=ORIENTED_EDGE('',*,*,#59555,.T.);
#88540=ORIENTED_EDGE('',*,*,#59546,.F.);
#88541=ORIENTED_EDGE('',*,*,#59559,.F.);
#88542=ORIENTED_EDGE('',*,*,#59560,.T.);
#88543=ORIENTED_EDGE('',*,*,#59557,.T.);
#88544=ORIENTED_EDGE('',*,*,#59545,.F.);
#88545=ORIENTED_EDGE('',*,*,#59561,.F.);
#88546=ORIENTED_EDGE('',*,*,#59562,.T.);
#88547=ORIENTED_EDGE('',*,*,#59559,.T.);
#88548=ORIENTED_EDGE('',*,*,#59544,.F.);
#88549=ORIENTED_EDGE('',*,*,#59563,.F.);
#88550=ORIENTED_EDGE('',*,*,#59564,.T.);
#88551=ORIENTED_EDGE('',*,*,#59561,.T.);
#88552=ORIENTED_EDGE('',*,*,#59543,.F.);
#88553=ORIENTED_EDGE('',*,*,#59565,.F.);
#88554=ORIENTED_EDGE('',*,*,#59566,.T.);
#88555=ORIENTED_EDGE('',*,*,#59563,.T.);
#88556=ORIENTED_EDGE('',*,*,#59542,.F.);
#88557=ORIENTED_EDGE('',*,*,#59532,.F.);
#88558=ORIENTED_EDGE('',*,*,#59567,.T.);
#88559=ORIENTED_EDGE('',*,*,#59565,.T.);
#88560=ORIENTED_EDGE('',*,*,#59541,.F.);
#88561=ORIENTED_EDGE('',*,*,#59568,.F.);
#88562=ORIENTED_EDGE('',*,*,#59569,.T.);
#88563=ORIENTED_EDGE('',*,*,#59534,.T.);
#88564=ORIENTED_EDGE('',*,*,#59540,.F.);
#88565=ORIENTED_EDGE('',*,*,#59570,.F.);
#88566=ORIENTED_EDGE('',*,*,#59571,.T.);
#88567=ORIENTED_EDGE('',*,*,#59568,.T.);
#88568=ORIENTED_EDGE('',*,*,#59539,.F.);
#88569=ORIENTED_EDGE('',*,*,#59572,.F.);
#88570=ORIENTED_EDGE('',*,*,#59573,.T.);
#88571=ORIENTED_EDGE('',*,*,#59570,.T.);
#88572=ORIENTED_EDGE('',*,*,#59538,.F.);
#88573=ORIENTED_EDGE('',*,*,#59574,.F.);
#88574=ORIENTED_EDGE('',*,*,#59575,.T.);
#88575=ORIENTED_EDGE('',*,*,#59572,.T.);
#88576=ORIENTED_EDGE('',*,*,#59537,.F.);
#88577=ORIENTED_EDGE('',*,*,#59576,.F.);
#88578=ORIENTED_EDGE('',*,*,#59577,.T.);
#88579=ORIENTED_EDGE('',*,*,#59574,.T.);
#88580=ORIENTED_EDGE('',*,*,#59536,.F.);
#88581=ORIENTED_EDGE('',*,*,#59552,.F.);
#88582=ORIENTED_EDGE('',*,*,#59578,.T.);
#88583=ORIENTED_EDGE('',*,*,#59576,.T.);
#88584=ORIENTED_EDGE('',*,*,#59535,.F.);
#88585=ORIENTED_EDGE('',*,*,#59578,.F.);
#88586=ORIENTED_EDGE('',*,*,#59551,.F.);
#88587=ORIENTED_EDGE('',*,*,#59554,.F.);
#88588=ORIENTED_EDGE('',*,*,#59556,.F.);
#88589=ORIENTED_EDGE('',*,*,#59558,.F.);
#88590=ORIENTED_EDGE('',*,*,#59560,.F.);
#88591=ORIENTED_EDGE('',*,*,#59562,.F.);
#88592=ORIENTED_EDGE('',*,*,#59564,.F.);
#88593=ORIENTED_EDGE('',*,*,#59566,.F.);
#88594=ORIENTED_EDGE('',*,*,#59567,.F.);
#88595=ORIENTED_EDGE('',*,*,#59531,.F.);
#88596=ORIENTED_EDGE('',*,*,#59569,.F.);
#88597=ORIENTED_EDGE('',*,*,#59571,.F.);
#88598=ORIENTED_EDGE('',*,*,#59573,.F.);
#88599=ORIENTED_EDGE('',*,*,#59575,.F.);
#88600=ORIENTED_EDGE('',*,*,#59577,.F.);
#88601=ORIENTED_EDGE('',*,*,#59579,.T.);
#88602=ORIENTED_EDGE('',*,*,#59580,.T.);
#88603=ORIENTED_EDGE('',*,*,#59581,.T.);
#88604=ORIENTED_EDGE('',*,*,#59582,.T.);
#88605=ORIENTED_EDGE('',*,*,#59583,.T.);
#88606=ORIENTED_EDGE('',*,*,#59584,.T.);
#88607=ORIENTED_EDGE('',*,*,#59585,.T.);
#88608=ORIENTED_EDGE('',*,*,#59586,.T.);
#88609=ORIENTED_EDGE('',*,*,#59587,.F.);
#88610=ORIENTED_EDGE('',*,*,#59588,.T.);
#88611=ORIENTED_EDGE('',*,*,#59589,.T.);
#88612=ORIENTED_EDGE('',*,*,#59586,.F.);
#88613=ORIENTED_EDGE('',*,*,#59590,.F.);
#88614=ORIENTED_EDGE('',*,*,#59591,.T.);
#88615=ORIENTED_EDGE('',*,*,#59587,.T.);
#88616=ORIENTED_EDGE('',*,*,#59585,.F.);
#88617=ORIENTED_EDGE('',*,*,#59592,.F.);
#88618=ORIENTED_EDGE('',*,*,#59593,.T.);
#88619=ORIENTED_EDGE('',*,*,#59590,.T.);
#88620=ORIENTED_EDGE('',*,*,#59584,.F.);
#88621=ORIENTED_EDGE('',*,*,#59594,.F.);
#88622=ORIENTED_EDGE('',*,*,#59595,.T.);
#88623=ORIENTED_EDGE('',*,*,#59592,.T.);
#88624=ORIENTED_EDGE('',*,*,#59583,.F.);
#88625=ORIENTED_EDGE('',*,*,#59596,.F.);
#88626=ORIENTED_EDGE('',*,*,#59597,.T.);
#88627=ORIENTED_EDGE('',*,*,#59594,.T.);
#88628=ORIENTED_EDGE('',*,*,#59582,.F.);
#88629=ORIENTED_EDGE('',*,*,#59598,.F.);
#88630=ORIENTED_EDGE('',*,*,#59599,.T.);
#88631=ORIENTED_EDGE('',*,*,#59596,.T.);
#88632=ORIENTED_EDGE('',*,*,#59581,.F.);
#88633=ORIENTED_EDGE('',*,*,#59600,.F.);
#88634=ORIENTED_EDGE('',*,*,#59601,.T.);
#88635=ORIENTED_EDGE('',*,*,#59598,.T.);
#88636=ORIENTED_EDGE('',*,*,#59580,.F.);
#88637=ORIENTED_EDGE('',*,*,#59589,.F.);
#88638=ORIENTED_EDGE('',*,*,#59602,.T.);
#88639=ORIENTED_EDGE('',*,*,#59600,.T.);
#88640=ORIENTED_EDGE('',*,*,#59579,.F.);
#88641=ORIENTED_EDGE('',*,*,#59602,.F.);
#88642=ORIENTED_EDGE('',*,*,#59588,.F.);
#88643=ORIENTED_EDGE('',*,*,#59591,.F.);
#88644=ORIENTED_EDGE('',*,*,#59593,.F.);
#88645=ORIENTED_EDGE('',*,*,#59595,.F.);
#88646=ORIENTED_EDGE('',*,*,#59597,.F.);
#88647=ORIENTED_EDGE('',*,*,#59599,.F.);
#88648=ORIENTED_EDGE('',*,*,#59601,.F.);
#88649=ORIENTED_EDGE('',*,*,#59603,.T.);
#88650=ORIENTED_EDGE('',*,*,#59604,.T.);
#88651=ORIENTED_EDGE('',*,*,#59605,.F.);
#88652=ORIENTED_EDGE('',*,*,#59606,.F.);
#88653=ORIENTED_EDGE('',*,*,#59607,.T.);
#88654=ORIENTED_EDGE('',*,*,#59608,.T.);
#88655=ORIENTED_EDGE('',*,*,#59605,.T.);
#88656=ORIENTED_EDGE('',*,*,#59609,.T.);
#88657=ORIENTED_EDGE('',*,*,#59610,.T.);
#88658=ORIENTED_EDGE('',*,*,#59611,.T.);
#88659=ORIENTED_EDGE('',*,*,#59612,.T.);
#88660=ORIENTED_EDGE('',*,*,#59613,.T.);
#88661=ORIENTED_EDGE('',*,*,#59614,.T.);
#88662=ORIENTED_EDGE('',*,*,#59615,.T.);
#88663=ORIENTED_EDGE('',*,*,#59616,.T.);
#88664=ORIENTED_EDGE('',*,*,#59617,.T.);
#88665=ORIENTED_EDGE('',*,*,#59618,.T.);
#88666=ORIENTED_EDGE('',*,*,#59619,.T.);
#88667=ORIENTED_EDGE('',*,*,#59620,.T.);
#88668=ORIENTED_EDGE('',*,*,#59621,.T.);
#88669=ORIENTED_EDGE('',*,*,#59622,.F.);
#88670=ORIENTED_EDGE('',*,*,#59623,.T.);
#88671=ORIENTED_EDGE('',*,*,#59624,.T.);
#88672=ORIENTED_EDGE('',*,*,#59621,.F.);
#88673=ORIENTED_EDGE('',*,*,#59625,.F.);
#88674=ORIENTED_EDGE('',*,*,#59626,.T.);
#88675=ORIENTED_EDGE('',*,*,#59622,.T.);
#88676=ORIENTED_EDGE('',*,*,#59620,.F.);
#88677=ORIENTED_EDGE('',*,*,#59627,.F.);
#88678=ORIENTED_EDGE('',*,*,#59628,.T.);
#88679=ORIENTED_EDGE('',*,*,#59625,.T.);
#88680=ORIENTED_EDGE('',*,*,#59619,.F.);
#88681=ORIENTED_EDGE('',*,*,#59629,.F.);
#88682=ORIENTED_EDGE('',*,*,#59630,.T.);
#88683=ORIENTED_EDGE('',*,*,#59627,.T.);
#88684=ORIENTED_EDGE('',*,*,#59618,.F.);
#88685=ORIENTED_EDGE('',*,*,#59631,.F.);
#88686=ORIENTED_EDGE('',*,*,#59632,.T.);
#88687=ORIENTED_EDGE('',*,*,#59629,.T.);
#88688=ORIENTED_EDGE('',*,*,#59617,.F.);
#88689=ORIENTED_EDGE('',*,*,#59633,.F.);
#88690=ORIENTED_EDGE('',*,*,#59634,.T.);
#88691=ORIENTED_EDGE('',*,*,#59631,.T.);
#88692=ORIENTED_EDGE('',*,*,#59616,.F.);
#88693=ORIENTED_EDGE('',*,*,#59635,.F.);
#88694=ORIENTED_EDGE('',*,*,#59636,.T.);
#88695=ORIENTED_EDGE('',*,*,#59633,.T.);
#88696=ORIENTED_EDGE('',*,*,#59615,.F.);
#88697=ORIENTED_EDGE('',*,*,#59637,.F.);
#88698=ORIENTED_EDGE('',*,*,#59638,.T.);
#88699=ORIENTED_EDGE('',*,*,#59635,.T.);
#88700=ORIENTED_EDGE('',*,*,#59614,.F.);
#88701=ORIENTED_EDGE('',*,*,#59639,.F.);
#88702=ORIENTED_EDGE('',*,*,#59640,.T.);
#88703=ORIENTED_EDGE('',*,*,#59637,.T.);
#88704=ORIENTED_EDGE('',*,*,#59613,.F.);
#88705=ORIENTED_EDGE('',*,*,#59641,.F.);
#88706=ORIENTED_EDGE('',*,*,#59642,.T.);
#88707=ORIENTED_EDGE('',*,*,#59639,.T.);
#88708=ORIENTED_EDGE('',*,*,#59612,.F.);
#88709=ORIENTED_EDGE('',*,*,#59643,.F.);
#88710=ORIENTED_EDGE('',*,*,#59644,.T.);
#88711=ORIENTED_EDGE('',*,*,#59641,.T.);
#88712=ORIENTED_EDGE('',*,*,#59611,.F.);
#88713=ORIENTED_EDGE('',*,*,#59645,.F.);
#88714=ORIENTED_EDGE('',*,*,#59646,.T.);
#88715=ORIENTED_EDGE('',*,*,#59643,.T.);
#88716=ORIENTED_EDGE('',*,*,#59610,.F.);
#88717=ORIENTED_EDGE('',*,*,#59604,.F.);
#88718=ORIENTED_EDGE('',*,*,#59647,.T.);
#88719=ORIENTED_EDGE('',*,*,#59645,.T.);
#88720=ORIENTED_EDGE('',*,*,#59609,.F.);
#88721=ORIENTED_EDGE('',*,*,#59648,.F.);
#88722=ORIENTED_EDGE('',*,*,#59649,.T.);
#88723=ORIENTED_EDGE('',*,*,#59606,.T.);
#88724=ORIENTED_EDGE('',*,*,#59608,.F.);
#88725=ORIENTED_EDGE('',*,*,#59624,.F.);
#88726=ORIENTED_EDGE('',*,*,#59650,.T.);
#88727=ORIENTED_EDGE('',*,*,#59648,.T.);
#88728=ORIENTED_EDGE('',*,*,#59607,.F.);
#88729=ORIENTED_EDGE('',*,*,#59650,.F.);
#88730=ORIENTED_EDGE('',*,*,#59623,.F.);
#88731=ORIENTED_EDGE('',*,*,#59626,.F.);
#88732=ORIENTED_EDGE('',*,*,#59628,.F.);
#88733=ORIENTED_EDGE('',*,*,#59630,.F.);
#88734=ORIENTED_EDGE('',*,*,#59632,.F.);
#88735=ORIENTED_EDGE('',*,*,#59634,.F.);
#88736=ORIENTED_EDGE('',*,*,#59636,.F.);
#88737=ORIENTED_EDGE('',*,*,#59638,.F.);
#88738=ORIENTED_EDGE('',*,*,#59640,.F.);
#88739=ORIENTED_EDGE('',*,*,#59642,.F.);
#88740=ORIENTED_EDGE('',*,*,#59644,.F.);
#88741=ORIENTED_EDGE('',*,*,#59646,.F.);
#88742=ORIENTED_EDGE('',*,*,#59647,.F.);
#88743=ORIENTED_EDGE('',*,*,#59603,.F.);
#88744=ORIENTED_EDGE('',*,*,#59649,.F.);
#88745=ORIENTED_EDGE('',*,*,#59651,.T.);
#88746=ORIENTED_EDGE('',*,*,#59652,.T.);
#88747=ORIENTED_EDGE('',*,*,#59653,.T.);
#88748=ORIENTED_EDGE('',*,*,#59654,.T.);
#88749=ORIENTED_EDGE('',*,*,#59655,.T.);
#88750=ORIENTED_EDGE('',*,*,#59656,.T.);
#88751=ORIENTED_EDGE('',*,*,#59657,.T.);
#88752=ORIENTED_EDGE('',*,*,#59658,.T.);
#88753=ORIENTED_EDGE('',*,*,#59659,.F.);
#88754=ORIENTED_EDGE('',*,*,#59660,.T.);
#88755=ORIENTED_EDGE('',*,*,#59661,.T.);
#88756=ORIENTED_EDGE('',*,*,#59658,.F.);
#88757=ORIENTED_EDGE('',*,*,#59662,.F.);
#88758=ORIENTED_EDGE('',*,*,#59663,.T.);
#88759=ORIENTED_EDGE('',*,*,#59659,.T.);
#88760=ORIENTED_EDGE('',*,*,#59657,.F.);
#88761=ORIENTED_EDGE('',*,*,#59664,.F.);
#88762=ORIENTED_EDGE('',*,*,#59665,.T.);
#88763=ORIENTED_EDGE('',*,*,#59662,.T.);
#88764=ORIENTED_EDGE('',*,*,#59656,.F.);
#88765=ORIENTED_EDGE('',*,*,#59666,.F.);
#88766=ORIENTED_EDGE('',*,*,#59667,.T.);
#88767=ORIENTED_EDGE('',*,*,#59664,.T.);
#88768=ORIENTED_EDGE('',*,*,#59655,.F.);
#88769=ORIENTED_EDGE('',*,*,#59668,.F.);
#88770=ORIENTED_EDGE('',*,*,#59669,.T.);
#88771=ORIENTED_EDGE('',*,*,#59666,.T.);
#88772=ORIENTED_EDGE('',*,*,#59654,.F.);
#88773=ORIENTED_EDGE('',*,*,#59670,.F.);
#88774=ORIENTED_EDGE('',*,*,#59671,.T.);
#88775=ORIENTED_EDGE('',*,*,#59668,.T.);
#88776=ORIENTED_EDGE('',*,*,#59653,.F.);
#88777=ORIENTED_EDGE('',*,*,#59672,.F.);
#88778=ORIENTED_EDGE('',*,*,#59673,.T.);
#88779=ORIENTED_EDGE('',*,*,#59670,.T.);
#88780=ORIENTED_EDGE('',*,*,#59652,.F.);
#88781=ORIENTED_EDGE('',*,*,#59661,.F.);
#88782=ORIENTED_EDGE('',*,*,#59674,.T.);
#88783=ORIENTED_EDGE('',*,*,#59672,.T.);
#88784=ORIENTED_EDGE('',*,*,#59651,.F.);
#88785=ORIENTED_EDGE('',*,*,#59674,.F.);
#88786=ORIENTED_EDGE('',*,*,#59660,.F.);
#88787=ORIENTED_EDGE('',*,*,#59663,.F.);
#88788=ORIENTED_EDGE('',*,*,#59665,.F.);
#88789=ORIENTED_EDGE('',*,*,#59667,.F.);
#88790=ORIENTED_EDGE('',*,*,#59669,.F.);
#88791=ORIENTED_EDGE('',*,*,#59671,.F.);
#88792=ORIENTED_EDGE('',*,*,#59673,.F.);
#88793=ORIENTED_EDGE('',*,*,#59675,.T.);
#88794=ORIENTED_EDGE('',*,*,#59676,.T.);
#88795=ORIENTED_EDGE('',*,*,#59677,.F.);
#88796=ORIENTED_EDGE('',*,*,#59678,.F.);
#88797=ORIENTED_EDGE('',*,*,#59679,.T.);
#88798=ORIENTED_EDGE('',*,*,#59680,.T.);
#88799=ORIENTED_EDGE('',*,*,#59677,.T.);
#88800=ORIENTED_EDGE('',*,*,#59681,.T.);
#88801=ORIENTED_EDGE('',*,*,#59682,.T.);
#88802=ORIENTED_EDGE('',*,*,#59683,.T.);
#88803=ORIENTED_EDGE('',*,*,#59684,.T.);
#88804=ORIENTED_EDGE('',*,*,#59685,.T.);
#88805=ORIENTED_EDGE('',*,*,#59686,.T.);
#88806=ORIENTED_EDGE('',*,*,#59687,.T.);
#88807=ORIENTED_EDGE('',*,*,#59688,.T.);
#88808=ORIENTED_EDGE('',*,*,#59689,.T.);
#88809=ORIENTED_EDGE('',*,*,#59690,.T.);
#88810=ORIENTED_EDGE('',*,*,#59691,.T.);
#88811=ORIENTED_EDGE('',*,*,#59692,.T.);
#88812=ORIENTED_EDGE('',*,*,#59693,.T.);
#88813=ORIENTED_EDGE('',*,*,#59694,.F.);
#88814=ORIENTED_EDGE('',*,*,#59695,.T.);
#88815=ORIENTED_EDGE('',*,*,#59696,.T.);
#88816=ORIENTED_EDGE('',*,*,#59693,.F.);
#88817=ORIENTED_EDGE('',*,*,#59697,.F.);
#88818=ORIENTED_EDGE('',*,*,#59698,.T.);
#88819=ORIENTED_EDGE('',*,*,#59694,.T.);
#88820=ORIENTED_EDGE('',*,*,#59692,.F.);
#88821=ORIENTED_EDGE('',*,*,#59699,.F.);
#88822=ORIENTED_EDGE('',*,*,#59700,.T.);
#88823=ORIENTED_EDGE('',*,*,#59697,.T.);
#88824=ORIENTED_EDGE('',*,*,#59691,.F.);
#88825=ORIENTED_EDGE('',*,*,#59701,.F.);
#88826=ORIENTED_EDGE('',*,*,#59702,.T.);
#88827=ORIENTED_EDGE('',*,*,#59699,.T.);
#88828=ORIENTED_EDGE('',*,*,#59690,.F.);
#88829=ORIENTED_EDGE('',*,*,#59703,.F.);
#88830=ORIENTED_EDGE('',*,*,#59704,.T.);
#88831=ORIENTED_EDGE('',*,*,#59701,.T.);
#88832=ORIENTED_EDGE('',*,*,#59689,.F.);
#88833=ORIENTED_EDGE('',*,*,#59705,.F.);
#88834=ORIENTED_EDGE('',*,*,#59706,.T.);
#88835=ORIENTED_EDGE('',*,*,#59703,.T.);
#88836=ORIENTED_EDGE('',*,*,#59688,.F.);
#88837=ORIENTED_EDGE('',*,*,#59707,.F.);
#88838=ORIENTED_EDGE('',*,*,#59708,.T.);
#88839=ORIENTED_EDGE('',*,*,#59705,.T.);
#88840=ORIENTED_EDGE('',*,*,#59687,.F.);
#88841=ORIENTED_EDGE('',*,*,#59709,.F.);
#88842=ORIENTED_EDGE('',*,*,#59710,.T.);
#88843=ORIENTED_EDGE('',*,*,#59707,.T.);
#88844=ORIENTED_EDGE('',*,*,#59686,.F.);
#88845=ORIENTED_EDGE('',*,*,#59711,.F.);
#88846=ORIENTED_EDGE('',*,*,#59712,.T.);
#88847=ORIENTED_EDGE('',*,*,#59709,.T.);
#88848=ORIENTED_EDGE('',*,*,#59685,.F.);
#88849=ORIENTED_EDGE('',*,*,#59713,.F.);
#88850=ORIENTED_EDGE('',*,*,#59714,.T.);
#88851=ORIENTED_EDGE('',*,*,#59711,.T.);
#88852=ORIENTED_EDGE('',*,*,#59684,.F.);
#88853=ORIENTED_EDGE('',*,*,#59715,.F.);
#88854=ORIENTED_EDGE('',*,*,#59716,.T.);
#88855=ORIENTED_EDGE('',*,*,#59713,.T.);
#88856=ORIENTED_EDGE('',*,*,#59683,.F.);
#88857=ORIENTED_EDGE('',*,*,#59717,.F.);
#88858=ORIENTED_EDGE('',*,*,#59718,.T.);
#88859=ORIENTED_EDGE('',*,*,#59715,.T.);
#88860=ORIENTED_EDGE('',*,*,#59682,.F.);
#88861=ORIENTED_EDGE('',*,*,#59676,.F.);
#88862=ORIENTED_EDGE('',*,*,#59719,.T.);
#88863=ORIENTED_EDGE('',*,*,#59717,.T.);
#88864=ORIENTED_EDGE('',*,*,#59681,.F.);
#88865=ORIENTED_EDGE('',*,*,#59720,.F.);
#88866=ORIENTED_EDGE('',*,*,#59721,.T.);
#88867=ORIENTED_EDGE('',*,*,#59678,.T.);
#88868=ORIENTED_EDGE('',*,*,#59680,.F.);
#88869=ORIENTED_EDGE('',*,*,#59696,.F.);
#88870=ORIENTED_EDGE('',*,*,#59722,.T.);
#88871=ORIENTED_EDGE('',*,*,#59720,.T.);
#88872=ORIENTED_EDGE('',*,*,#59679,.F.);
#88873=ORIENTED_EDGE('',*,*,#59722,.F.);
#88874=ORIENTED_EDGE('',*,*,#59695,.F.);
#88875=ORIENTED_EDGE('',*,*,#59698,.F.);
#88876=ORIENTED_EDGE('',*,*,#59700,.F.);
#88877=ORIENTED_EDGE('',*,*,#59702,.F.);
#88878=ORIENTED_EDGE('',*,*,#59704,.F.);
#88879=ORIENTED_EDGE('',*,*,#59706,.F.);
#88880=ORIENTED_EDGE('',*,*,#59708,.F.);
#88881=ORIENTED_EDGE('',*,*,#59710,.F.);
#88882=ORIENTED_EDGE('',*,*,#59712,.F.);
#88883=ORIENTED_EDGE('',*,*,#59714,.F.);
#88884=ORIENTED_EDGE('',*,*,#59716,.F.);
#88885=ORIENTED_EDGE('',*,*,#59718,.F.);
#88886=ORIENTED_EDGE('',*,*,#59719,.F.);
#88887=ORIENTED_EDGE('',*,*,#59675,.F.);
#88888=ORIENTED_EDGE('',*,*,#59721,.F.);
#88889=ORIENTED_EDGE('',*,*,#59723,.T.);
#88890=ORIENTED_EDGE('',*,*,#59724,.T.);
#88891=ORIENTED_EDGE('',*,*,#59725,.T.);
#88892=ORIENTED_EDGE('',*,*,#59726,.T.);
#88893=ORIENTED_EDGE('',*,*,#59727,.T.);
#88894=ORIENTED_EDGE('',*,*,#59728,.T.);
#88895=ORIENTED_EDGE('',*,*,#59729,.T.);
#88896=ORIENTED_EDGE('',*,*,#59730,.T.);
#88897=ORIENTED_EDGE('',*,*,#59731,.F.);
#88898=ORIENTED_EDGE('',*,*,#59732,.T.);
#88899=ORIENTED_EDGE('',*,*,#59733,.T.);
#88900=ORIENTED_EDGE('',*,*,#59730,.F.);
#88901=ORIENTED_EDGE('',*,*,#59734,.F.);
#88902=ORIENTED_EDGE('',*,*,#59735,.T.);
#88903=ORIENTED_EDGE('',*,*,#59731,.T.);
#88904=ORIENTED_EDGE('',*,*,#59729,.F.);
#88905=ORIENTED_EDGE('',*,*,#59736,.F.);
#88906=ORIENTED_EDGE('',*,*,#59737,.T.);
#88907=ORIENTED_EDGE('',*,*,#59734,.T.);
#88908=ORIENTED_EDGE('',*,*,#59728,.F.);
#88909=ORIENTED_EDGE('',*,*,#59738,.F.);
#88910=ORIENTED_EDGE('',*,*,#59739,.T.);
#88911=ORIENTED_EDGE('',*,*,#59736,.T.);
#88912=ORIENTED_EDGE('',*,*,#59727,.F.);
#88913=ORIENTED_EDGE('',*,*,#59740,.F.);
#88914=ORIENTED_EDGE('',*,*,#59741,.T.);
#88915=ORIENTED_EDGE('',*,*,#59738,.T.);
#88916=ORIENTED_EDGE('',*,*,#59726,.F.);
#88917=ORIENTED_EDGE('',*,*,#59742,.F.);
#88918=ORIENTED_EDGE('',*,*,#59743,.T.);
#88919=ORIENTED_EDGE('',*,*,#59740,.T.);
#88920=ORIENTED_EDGE('',*,*,#59725,.F.);
#88921=ORIENTED_EDGE('',*,*,#59744,.F.);
#88922=ORIENTED_EDGE('',*,*,#59745,.T.);
#88923=ORIENTED_EDGE('',*,*,#59742,.T.);
#88924=ORIENTED_EDGE('',*,*,#59724,.F.);
#88925=ORIENTED_EDGE('',*,*,#59733,.F.);
#88926=ORIENTED_EDGE('',*,*,#59746,.T.);
#88927=ORIENTED_EDGE('',*,*,#59744,.T.);
#88928=ORIENTED_EDGE('',*,*,#59723,.F.);
#88929=ORIENTED_EDGE('',*,*,#59746,.F.);
#88930=ORIENTED_EDGE('',*,*,#59732,.F.);
#88931=ORIENTED_EDGE('',*,*,#59735,.F.);
#88932=ORIENTED_EDGE('',*,*,#59737,.F.);
#88933=ORIENTED_EDGE('',*,*,#59739,.F.);
#88934=ORIENTED_EDGE('',*,*,#59741,.F.);
#88935=ORIENTED_EDGE('',*,*,#59743,.F.);
#88936=ORIENTED_EDGE('',*,*,#59745,.F.);
#88937=ORIENTED_EDGE('',*,*,#59747,.F.);
#88938=ORIENTED_EDGE('',*,*,#59748,.T.);
#88939=ORIENTED_EDGE('',*,*,#59749,.T.);
#88940=ORIENTED_EDGE('',*,*,#59750,.T.);
#88941=ORIENTED_EDGE('',*,*,#59751,.F.);
#88942=ORIENTED_EDGE('',*,*,#59752,.T.);
#88943=ORIENTED_EDGE('',*,*,#59753,.T.);
#88944=ORIENTED_EDGE('',*,*,#59754,.F.);
#88945=ORIENTED_EDGE('',*,*,#59755,.F.);
#88946=ORIENTED_EDGE('',*,*,#59756,.T.);
#88947=ORIENTED_EDGE('',*,*,#59757,.T.);
#88948=ORIENTED_EDGE('',*,*,#59758,.F.);
#88949=ORIENTED_EDGE('',*,*,#59759,.F.);
#88950=ORIENTED_EDGE('',*,*,#59758,.T.);
#88951=ORIENTED_EDGE('',*,*,#59760,.T.);
#88952=ORIENTED_EDGE('',*,*,#59761,.F.);
#88953=ORIENTED_EDGE('',*,*,#59762,.F.);
#88954=ORIENTED_EDGE('',*,*,#59761,.T.);
#88955=ORIENTED_EDGE('',*,*,#59763,.T.);
#88956=ORIENTED_EDGE('',*,*,#59764,.F.);
#88957=ORIENTED_EDGE('',*,*,#59765,.F.);
#88958=ORIENTED_EDGE('',*,*,#59764,.T.);
#88959=ORIENTED_EDGE('',*,*,#59766,.T.);
#88960=ORIENTED_EDGE('',*,*,#59767,.F.);
#88961=ORIENTED_EDGE('',*,*,#59768,.F.);
#88962=ORIENTED_EDGE('',*,*,#59767,.T.);
#88963=ORIENTED_EDGE('',*,*,#59769,.T.);
#88964=ORIENTED_EDGE('',*,*,#59770,.F.);
#88965=ORIENTED_EDGE('',*,*,#59771,.F.);
#88966=ORIENTED_EDGE('',*,*,#59770,.T.);
#88967=ORIENTED_EDGE('',*,*,#59772,.T.);
#88968=ORIENTED_EDGE('',*,*,#59773,.F.);
#88969=ORIENTED_EDGE('',*,*,#59774,.F.);
#88970=ORIENTED_EDGE('',*,*,#59773,.T.);
#88971=ORIENTED_EDGE('',*,*,#59775,.T.);
#88972=ORIENTED_EDGE('',*,*,#59776,.F.);
#88973=ORIENTED_EDGE('',*,*,#59777,.F.);
#88974=ORIENTED_EDGE('',*,*,#59776,.T.);
#88975=ORIENTED_EDGE('',*,*,#59778,.T.);
#88976=ORIENTED_EDGE('',*,*,#59779,.F.);
#88977=ORIENTED_EDGE('',*,*,#59780,.F.);
#88978=ORIENTED_EDGE('',*,*,#59779,.T.);
#88979=ORIENTED_EDGE('',*,*,#59781,.T.);
#88980=ORIENTED_EDGE('',*,*,#59782,.F.);
#88981=ORIENTED_EDGE('',*,*,#59783,.F.);
#88982=ORIENTED_EDGE('',*,*,#59782,.T.);
#88983=ORIENTED_EDGE('',*,*,#59784,.T.);
#88984=ORIENTED_EDGE('',*,*,#59785,.F.);
#88985=ORIENTED_EDGE('',*,*,#59786,.F.);
#88986=ORIENTED_EDGE('',*,*,#59785,.T.);
#88987=ORIENTED_EDGE('',*,*,#59787,.T.);
#88988=ORIENTED_EDGE('',*,*,#59788,.F.);
#88989=ORIENTED_EDGE('',*,*,#59789,.F.);
#88990=ORIENTED_EDGE('',*,*,#59788,.T.);
#88991=ORIENTED_EDGE('',*,*,#59790,.T.);
#88992=ORIENTED_EDGE('',*,*,#59791,.F.);
#88993=ORIENTED_EDGE('',*,*,#59792,.F.);
#88994=ORIENTED_EDGE('',*,*,#59791,.T.);
#88995=ORIENTED_EDGE('',*,*,#59793,.T.);
#88996=ORIENTED_EDGE('',*,*,#59794,.F.);
#88997=ORIENTED_EDGE('',*,*,#59795,.F.);
#88998=ORIENTED_EDGE('',*,*,#59794,.T.);
#88999=ORIENTED_EDGE('',*,*,#59796,.T.);
#89000=ORIENTED_EDGE('',*,*,#59797,.F.);
#89001=ORIENTED_EDGE('',*,*,#59798,.F.);
#89002=ORIENTED_EDGE('',*,*,#59799,.T.);
#89003=ORIENTED_EDGE('',*,*,#59800,.T.);
#89004=ORIENTED_EDGE('',*,*,#59801,.F.);
#89005=ORIENTED_EDGE('',*,*,#59802,.F.);
#89006=ORIENTED_EDGE('',*,*,#59801,.T.);
#89007=ORIENTED_EDGE('',*,*,#59803,.T.);
#89008=ORIENTED_EDGE('',*,*,#59804,.F.);
#89009=ORIENTED_EDGE('',*,*,#59805,.F.);
#89010=ORIENTED_EDGE('',*,*,#59804,.T.);
#89011=ORIENTED_EDGE('',*,*,#59806,.T.);
#89012=ORIENTED_EDGE('',*,*,#59807,.F.);
#89013=ORIENTED_EDGE('',*,*,#59808,.F.);
#89014=ORIENTED_EDGE('',*,*,#59807,.T.);
#89015=ORIENTED_EDGE('',*,*,#59809,.T.);
#89016=ORIENTED_EDGE('',*,*,#59810,.F.);
#89017=ORIENTED_EDGE('',*,*,#59811,.F.);
#89018=ORIENTED_EDGE('',*,*,#59810,.T.);
#89019=ORIENTED_EDGE('',*,*,#59812,.T.);
#89020=ORIENTED_EDGE('',*,*,#59813,.F.);
#89021=ORIENTED_EDGE('',*,*,#59814,.F.);
#89022=ORIENTED_EDGE('',*,*,#59813,.T.);
#89023=ORIENTED_EDGE('',*,*,#59815,.T.);
#89024=ORIENTED_EDGE('',*,*,#59816,.F.);
#89025=ORIENTED_EDGE('',*,*,#59817,.F.);
#89026=ORIENTED_EDGE('',*,*,#59816,.T.);
#89027=ORIENTED_EDGE('',*,*,#59818,.T.);
#89028=ORIENTED_EDGE('',*,*,#59819,.F.);
#89029=ORIENTED_EDGE('',*,*,#59820,.F.);
#89030=ORIENTED_EDGE('',*,*,#59819,.T.);
#89031=ORIENTED_EDGE('',*,*,#59821,.T.);
#89032=ORIENTED_EDGE('',*,*,#59822,.F.);
#89033=ORIENTED_EDGE('',*,*,#59823,.F.);
#89034=ORIENTED_EDGE('',*,*,#59822,.T.);
#89035=ORIENTED_EDGE('',*,*,#59824,.T.);
#89036=ORIENTED_EDGE('',*,*,#59825,.F.);
#89037=ORIENTED_EDGE('',*,*,#59826,.F.);
#89038=ORIENTED_EDGE('',*,*,#59825,.T.);
#89039=ORIENTED_EDGE('',*,*,#59827,.T.);
#89040=ORIENTED_EDGE('',*,*,#59828,.F.);
#89041=ORIENTED_EDGE('',*,*,#59829,.F.);
#89042=ORIENTED_EDGE('',*,*,#59828,.T.);
#89043=ORIENTED_EDGE('',*,*,#59830,.T.);
#89044=ORIENTED_EDGE('',*,*,#59831,.F.);
#89045=ORIENTED_EDGE('',*,*,#59832,.F.);
#89046=ORIENTED_EDGE('',*,*,#59831,.T.);
#89047=ORIENTED_EDGE('',*,*,#59833,.T.);
#89048=ORIENTED_EDGE('',*,*,#59834,.F.);
#89049=ORIENTED_EDGE('',*,*,#59835,.F.);
#89050=ORIENTED_EDGE('',*,*,#59834,.T.);
#89051=ORIENTED_EDGE('',*,*,#59836,.T.);
#89052=ORIENTED_EDGE('',*,*,#59837,.F.);
#89053=ORIENTED_EDGE('',*,*,#59838,.F.);
#89054=ORIENTED_EDGE('',*,*,#59837,.T.);
#89055=ORIENTED_EDGE('',*,*,#59839,.T.);
#89056=ORIENTED_EDGE('',*,*,#59840,.F.);
#89057=ORIENTED_EDGE('',*,*,#59841,.F.);
#89058=ORIENTED_EDGE('',*,*,#59840,.T.);
#89059=ORIENTED_EDGE('',*,*,#59842,.T.);
#89060=ORIENTED_EDGE('',*,*,#59843,.F.);
#89061=ORIENTED_EDGE('',*,*,#59844,.F.);
#89062=ORIENTED_EDGE('',*,*,#59843,.T.);
#89063=ORIENTED_EDGE('',*,*,#59845,.T.);
#89064=ORIENTED_EDGE('',*,*,#59846,.F.);
#89065=ORIENTED_EDGE('',*,*,#59847,.F.);
#89066=ORIENTED_EDGE('',*,*,#59846,.T.);
#89067=ORIENTED_EDGE('',*,*,#59848,.T.);
#89068=ORIENTED_EDGE('',*,*,#59849,.F.);
#89069=ORIENTED_EDGE('',*,*,#59850,.F.);
#89070=ORIENTED_EDGE('',*,*,#59849,.T.);
#89071=ORIENTED_EDGE('',*,*,#59851,.T.);
#89072=ORIENTED_EDGE('',*,*,#59852,.F.);
#89073=ORIENTED_EDGE('',*,*,#59853,.F.);
#89074=ORIENTED_EDGE('',*,*,#59852,.T.);
#89075=ORIENTED_EDGE('',*,*,#59854,.T.);
#89076=ORIENTED_EDGE('',*,*,#59855,.F.);
#89077=ORIENTED_EDGE('',*,*,#59856,.F.);
#89078=ORIENTED_EDGE('',*,*,#59855,.T.);
#89079=ORIENTED_EDGE('',*,*,#59857,.T.);
#89080=ORIENTED_EDGE('',*,*,#59748,.F.);
#89081=ORIENTED_EDGE('',*,*,#59858,.F.);
#89082=ORIENTED_EDGE('',*,*,#59859,.T.);
#89083=ORIENTED_EDGE('',*,*,#59860,.T.);
#89084=ORIENTED_EDGE('',*,*,#59861,.F.);
#89085=ORIENTED_EDGE('',*,*,#59862,.F.);
#89086=ORIENTED_EDGE('',*,*,#59861,.T.);
#89087=ORIENTED_EDGE('',*,*,#59863,.T.);
#89088=ORIENTED_EDGE('',*,*,#59864,.F.);
#89089=ORIENTED_EDGE('',*,*,#59865,.F.);
#89090=ORIENTED_EDGE('',*,*,#59864,.T.);
#89091=ORIENTED_EDGE('',*,*,#59866,.T.);
#89092=ORIENTED_EDGE('',*,*,#59867,.F.);
#89093=ORIENTED_EDGE('',*,*,#59868,.F.);
#89094=ORIENTED_EDGE('',*,*,#59867,.T.);
#89095=ORIENTED_EDGE('',*,*,#59869,.T.);
#89096=ORIENTED_EDGE('',*,*,#59870,.F.);
#89097=ORIENTED_EDGE('',*,*,#59871,.F.);
#89098=ORIENTED_EDGE('',*,*,#59870,.T.);
#89099=ORIENTED_EDGE('',*,*,#59872,.T.);
#89100=ORIENTED_EDGE('',*,*,#59873,.F.);
#89101=ORIENTED_EDGE('',*,*,#59874,.F.);
#89102=ORIENTED_EDGE('',*,*,#59873,.T.);
#89103=ORIENTED_EDGE('',*,*,#59875,.T.);
#89104=ORIENTED_EDGE('',*,*,#59876,.F.);
#89105=ORIENTED_EDGE('',*,*,#59877,.F.);
#89106=ORIENTED_EDGE('',*,*,#59876,.T.);
#89107=ORIENTED_EDGE('',*,*,#59878,.T.);
#89108=ORIENTED_EDGE('',*,*,#59879,.F.);
#89109=ORIENTED_EDGE('',*,*,#59880,.F.);
#89110=ORIENTED_EDGE('',*,*,#59879,.T.);
#89111=ORIENTED_EDGE('',*,*,#59881,.T.);
#89112=ORIENTED_EDGE('',*,*,#59882,.F.);
#89113=ORIENTED_EDGE('',*,*,#59883,.F.);
#89114=ORIENTED_EDGE('',*,*,#59882,.T.);
#89115=ORIENTED_EDGE('',*,*,#59884,.T.);
#89116=ORIENTED_EDGE('',*,*,#59885,.F.);
#89117=ORIENTED_EDGE('',*,*,#59886,.F.);
#89118=ORIENTED_EDGE('',*,*,#59885,.T.);
#89119=ORIENTED_EDGE('',*,*,#59887,.T.);
#89120=ORIENTED_EDGE('',*,*,#59888,.F.);
#89121=ORIENTED_EDGE('',*,*,#59889,.F.);
#89122=ORIENTED_EDGE('',*,*,#59888,.T.);
#89123=ORIENTED_EDGE('',*,*,#59890,.T.);
#89124=ORIENTED_EDGE('',*,*,#59891,.F.);
#89125=ORIENTED_EDGE('',*,*,#59892,.F.);
#89126=ORIENTED_EDGE('',*,*,#59891,.T.);
#89127=ORIENTED_EDGE('',*,*,#59893,.T.);
#89128=ORIENTED_EDGE('',*,*,#59894,.F.);
#89129=ORIENTED_EDGE('',*,*,#59895,.F.);
#89130=ORIENTED_EDGE('',*,*,#59894,.T.);
#89131=ORIENTED_EDGE('',*,*,#59896,.T.);
#89132=ORIENTED_EDGE('',*,*,#59897,.T.);
#89133=ORIENTED_EDGE('',*,*,#59898,.F.);
#89134=ORIENTED_EDGE('',*,*,#59754,.T.);
#89135=ORIENTED_EDGE('',*,*,#59899,.T.);
#89136=ORIENTED_EDGE('',*,*,#59900,.F.);
#89137=ORIENTED_EDGE('',*,*,#59901,.F.);
#89138=ORIENTED_EDGE('',*,*,#59900,.T.);
#89139=ORIENTED_EDGE('',*,*,#59902,.T.);
#89140=ORIENTED_EDGE('',*,*,#59903,.F.);
#89141=ORIENTED_EDGE('',*,*,#59904,.F.);
#89142=ORIENTED_EDGE('',*,*,#59903,.T.);
#89143=ORIENTED_EDGE('',*,*,#59905,.T.);
#89144=ORIENTED_EDGE('',*,*,#59906,.F.);
#89145=ORIENTED_EDGE('',*,*,#59907,.F.);
#89146=ORIENTED_EDGE('',*,*,#59906,.T.);
#89147=ORIENTED_EDGE('',*,*,#59908,.T.);
#89148=ORIENTED_EDGE('',*,*,#59909,.F.);
#89149=ORIENTED_EDGE('',*,*,#59910,.F.);
#89150=ORIENTED_EDGE('',*,*,#59909,.T.);
#89151=ORIENTED_EDGE('',*,*,#59911,.T.);
#89152=ORIENTED_EDGE('',*,*,#59912,.F.);
#89153=ORIENTED_EDGE('',*,*,#59913,.F.);
#89154=ORIENTED_EDGE('',*,*,#59912,.T.);
#89155=ORIENTED_EDGE('',*,*,#59914,.T.);
#89156=ORIENTED_EDGE('',*,*,#59756,.F.);
#89157=ORIENTED_EDGE('',*,*,#59915,.F.);
#89158=ORIENTED_EDGE('',*,*,#59916,.T.);
#89159=ORIENTED_EDGE('',*,*,#59917,.T.);
#89160=ORIENTED_EDGE('',*,*,#59918,.F.);
#89161=ORIENTED_EDGE('',*,*,#59919,.F.);
#89162=ORIENTED_EDGE('',*,*,#59918,.T.);
#89163=ORIENTED_EDGE('',*,*,#59920,.T.);
#89164=ORIENTED_EDGE('',*,*,#59921,.F.);
#89165=ORIENTED_EDGE('',*,*,#59922,.F.);
#89166=ORIENTED_EDGE('',*,*,#59921,.T.);
#89167=ORIENTED_EDGE('',*,*,#59923,.T.);
#89168=ORIENTED_EDGE('',*,*,#59924,.F.);
#89169=ORIENTED_EDGE('',*,*,#59925,.F.);
#89170=ORIENTED_EDGE('',*,*,#59924,.T.);
#89171=ORIENTED_EDGE('',*,*,#59926,.T.);
#89172=ORIENTED_EDGE('',*,*,#59927,.F.);
#89173=ORIENTED_EDGE('',*,*,#59928,.F.);
#89174=ORIENTED_EDGE('',*,*,#59927,.T.);
#89175=ORIENTED_EDGE('',*,*,#59929,.T.);
#89176=ORIENTED_EDGE('',*,*,#59930,.F.);
#89177=ORIENTED_EDGE('',*,*,#59931,.F.);
#89178=ORIENTED_EDGE('',*,*,#59930,.T.);
#89179=ORIENTED_EDGE('',*,*,#59932,.T.);
#89180=ORIENTED_EDGE('',*,*,#59933,.F.);
#89181=ORIENTED_EDGE('',*,*,#59934,.F.);
#89182=ORIENTED_EDGE('',*,*,#59933,.T.);
#89183=ORIENTED_EDGE('',*,*,#59935,.T.);
#89184=ORIENTED_EDGE('',*,*,#59936,.F.);
#89185=ORIENTED_EDGE('',*,*,#59937,.F.);
#89186=ORIENTED_EDGE('',*,*,#59936,.T.);
#89187=ORIENTED_EDGE('',*,*,#59938,.T.);
#89188=ORIENTED_EDGE('',*,*,#59939,.F.);
#89189=ORIENTED_EDGE('',*,*,#59940,.F.);
#89190=ORIENTED_EDGE('',*,*,#59939,.T.);
#89191=ORIENTED_EDGE('',*,*,#59941,.T.);
#89192=ORIENTED_EDGE('',*,*,#59942,.F.);
#89193=ORIENTED_EDGE('',*,*,#59943,.F.);
#89194=ORIENTED_EDGE('',*,*,#59942,.T.);
#89195=ORIENTED_EDGE('',*,*,#59944,.T.);
#89196=ORIENTED_EDGE('',*,*,#59945,.F.);
#89197=ORIENTED_EDGE('',*,*,#59946,.F.);
#89198=ORIENTED_EDGE('',*,*,#59945,.T.);
#89199=ORIENTED_EDGE('',*,*,#59947,.T.);
#89200=ORIENTED_EDGE('',*,*,#59948,.F.);
#89201=ORIENTED_EDGE('',*,*,#59949,.F.);
#89202=ORIENTED_EDGE('',*,*,#59948,.T.);
#89203=ORIENTED_EDGE('',*,*,#59950,.T.);
#89204=ORIENTED_EDGE('',*,*,#59951,.F.);
#89205=ORIENTED_EDGE('',*,*,#59952,.F.);
#89206=ORIENTED_EDGE('',*,*,#59951,.T.);
#89207=ORIENTED_EDGE('',*,*,#59953,.T.);
#89208=ORIENTED_EDGE('',*,*,#59799,.F.);
#89209=ORIENTED_EDGE('',*,*,#59954,.F.);
#89210=ORIENTED_EDGE('',*,*,#59955,.T.);
#89211=ORIENTED_EDGE('',*,*,#59956,.T.);
#89212=ORIENTED_EDGE('',*,*,#59957,.F.);
#89213=ORIENTED_EDGE('',*,*,#59958,.F.);
#89214=ORIENTED_EDGE('',*,*,#59957,.T.);
#89215=ORIENTED_EDGE('',*,*,#59959,.T.);
#89216=ORIENTED_EDGE('',*,*,#59960,.F.);
#89217=ORIENTED_EDGE('',*,*,#59961,.F.);
#89218=ORIENTED_EDGE('',*,*,#59960,.T.);
#89219=ORIENTED_EDGE('',*,*,#59962,.T.);
#89220=ORIENTED_EDGE('',*,*,#59963,.F.);
#89221=ORIENTED_EDGE('',*,*,#59964,.F.);
#89222=ORIENTED_EDGE('',*,*,#59963,.T.);
#89223=ORIENTED_EDGE('',*,*,#59965,.T.);
#89224=ORIENTED_EDGE('',*,*,#59966,.F.);
#89225=ORIENTED_EDGE('',*,*,#59967,.F.);
#89226=ORIENTED_EDGE('',*,*,#59966,.T.);
#89227=ORIENTED_EDGE('',*,*,#59968,.T.);
#89228=ORIENTED_EDGE('',*,*,#59969,.F.);
#89229=ORIENTED_EDGE('',*,*,#59970,.F.);
#89230=ORIENTED_EDGE('',*,*,#59969,.T.);
#89231=ORIENTED_EDGE('',*,*,#59971,.T.);
#89232=ORIENTED_EDGE('',*,*,#59972,.F.);
#89233=ORIENTED_EDGE('',*,*,#59973,.F.);
#89234=ORIENTED_EDGE('',*,*,#59972,.T.);
#89235=ORIENTED_EDGE('',*,*,#59974,.T.);
#89236=ORIENTED_EDGE('',*,*,#59975,.F.);
#89237=ORIENTED_EDGE('',*,*,#59976,.F.);
#89238=ORIENTED_EDGE('',*,*,#59975,.T.);
#89239=ORIENTED_EDGE('',*,*,#59977,.T.);
#89240=ORIENTED_EDGE('',*,*,#59978,.F.);
#89241=ORIENTED_EDGE('',*,*,#59979,.F.);
#89242=ORIENTED_EDGE('',*,*,#59978,.T.);
#89243=ORIENTED_EDGE('',*,*,#59980,.T.);
#89244=ORIENTED_EDGE('',*,*,#59981,.F.);
#89245=ORIENTED_EDGE('',*,*,#59982,.F.);
#89246=ORIENTED_EDGE('',*,*,#59981,.T.);
#89247=ORIENTED_EDGE('',*,*,#59983,.T.);
#89248=ORIENTED_EDGE('',*,*,#59984,.F.);
#89249=ORIENTED_EDGE('',*,*,#59985,.F.);
#89250=ORIENTED_EDGE('',*,*,#59984,.T.);
#89251=ORIENTED_EDGE('',*,*,#59986,.T.);
#89252=ORIENTED_EDGE('',*,*,#59987,.F.);
#89253=ORIENTED_EDGE('',*,*,#59988,.F.);
#89254=ORIENTED_EDGE('',*,*,#59987,.T.);
#89255=ORIENTED_EDGE('',*,*,#59989,.T.);
#89256=ORIENTED_EDGE('',*,*,#59990,.F.);
#89257=ORIENTED_EDGE('',*,*,#59991,.F.);
#89258=ORIENTED_EDGE('',*,*,#59990,.T.);
#89259=ORIENTED_EDGE('',*,*,#59992,.T.);
#89260=ORIENTED_EDGE('',*,*,#59993,.F.);
#89261=ORIENTED_EDGE('',*,*,#59994,.F.);
#89262=ORIENTED_EDGE('',*,*,#59993,.T.);
#89263=ORIENTED_EDGE('',*,*,#59995,.T.);
#89264=ORIENTED_EDGE('',*,*,#59996,.F.);
#89265=ORIENTED_EDGE('',*,*,#59997,.F.);
#89266=ORIENTED_EDGE('',*,*,#59996,.T.);
#89267=ORIENTED_EDGE('',*,*,#59998,.T.);
#89268=ORIENTED_EDGE('',*,*,#59999,.F.);
#89269=ORIENTED_EDGE('',*,*,#60000,.F.);
#89270=ORIENTED_EDGE('',*,*,#59999,.T.);
#89271=ORIENTED_EDGE('',*,*,#60001,.T.);
#89272=ORIENTED_EDGE('',*,*,#60002,.F.);
#89273=ORIENTED_EDGE('',*,*,#60003,.F.);
#89274=ORIENTED_EDGE('',*,*,#60002,.T.);
#89275=ORIENTED_EDGE('',*,*,#60004,.T.);
#89276=ORIENTED_EDGE('',*,*,#60005,.F.);
#89277=ORIENTED_EDGE('',*,*,#60006,.F.);
#89278=ORIENTED_EDGE('',*,*,#60005,.T.);
#89279=ORIENTED_EDGE('',*,*,#60007,.T.);
#89280=ORIENTED_EDGE('',*,*,#60008,.F.);
#89281=ORIENTED_EDGE('',*,*,#60009,.F.);
#89282=ORIENTED_EDGE('',*,*,#60008,.T.);
#89283=ORIENTED_EDGE('',*,*,#60010,.T.);
#89284=ORIENTED_EDGE('',*,*,#60011,.F.);
#89285=ORIENTED_EDGE('',*,*,#60012,.F.);
#89286=ORIENTED_EDGE('',*,*,#60011,.T.);
#89287=ORIENTED_EDGE('',*,*,#60013,.T.);
#89288=ORIENTED_EDGE('',*,*,#60014,.F.);
#89289=ORIENTED_EDGE('',*,*,#60015,.F.);
#89290=ORIENTED_EDGE('',*,*,#60014,.T.);
#89291=ORIENTED_EDGE('',*,*,#60016,.T.);
#89292=ORIENTED_EDGE('',*,*,#60017,.F.);
#89293=ORIENTED_EDGE('',*,*,#60018,.F.);
#89294=ORIENTED_EDGE('',*,*,#60017,.T.);
#89295=ORIENTED_EDGE('',*,*,#60019,.T.);
#89296=ORIENTED_EDGE('',*,*,#60020,.F.);
#89297=ORIENTED_EDGE('',*,*,#60021,.F.);
#89298=ORIENTED_EDGE('',*,*,#60020,.T.);
#89299=ORIENTED_EDGE('',*,*,#60022,.T.);
#89300=ORIENTED_EDGE('',*,*,#60023,.F.);
#89301=ORIENTED_EDGE('',*,*,#60024,.F.);
#89302=ORIENTED_EDGE('',*,*,#60023,.T.);
#89303=ORIENTED_EDGE('',*,*,#60025,.T.);
#89304=ORIENTED_EDGE('',*,*,#60026,.F.);
#89305=ORIENTED_EDGE('',*,*,#60027,.F.);
#89306=ORIENTED_EDGE('',*,*,#60026,.T.);
#89307=ORIENTED_EDGE('',*,*,#60028,.T.);
#89308=ORIENTED_EDGE('',*,*,#60029,.F.);
#89309=ORIENTED_EDGE('',*,*,#60030,.F.);
#89310=ORIENTED_EDGE('',*,*,#60029,.T.);
#89311=ORIENTED_EDGE('',*,*,#60031,.T.);
#89312=ORIENTED_EDGE('',*,*,#60032,.F.);
#89313=ORIENTED_EDGE('',*,*,#60033,.F.);
#89314=ORIENTED_EDGE('',*,*,#60032,.T.);
#89315=ORIENTED_EDGE('',*,*,#60034,.T.);
#89316=ORIENTED_EDGE('',*,*,#60035,.F.);
#89317=ORIENTED_EDGE('',*,*,#60036,.F.);
#89318=ORIENTED_EDGE('',*,*,#60035,.T.);
#89319=ORIENTED_EDGE('',*,*,#60037,.T.);
#89320=ORIENTED_EDGE('',*,*,#60038,.F.);
#89321=ORIENTED_EDGE('',*,*,#60039,.F.);
#89322=ORIENTED_EDGE('',*,*,#60038,.T.);
#89323=ORIENTED_EDGE('',*,*,#60040,.T.);
#89324=ORIENTED_EDGE('',*,*,#60041,.F.);
#89325=ORIENTED_EDGE('',*,*,#60042,.F.);
#89326=ORIENTED_EDGE('',*,*,#60041,.T.);
#89327=ORIENTED_EDGE('',*,*,#60043,.T.);
#89328=ORIENTED_EDGE('',*,*,#60044,.F.);
#89329=ORIENTED_EDGE('',*,*,#60045,.F.);
#89330=ORIENTED_EDGE('',*,*,#60044,.T.);
#89331=ORIENTED_EDGE('',*,*,#60046,.T.);
#89332=ORIENTED_EDGE('',*,*,#60047,.F.);
#89333=ORIENTED_EDGE('',*,*,#60048,.F.);
#89334=ORIENTED_EDGE('',*,*,#60047,.T.);
#89335=ORIENTED_EDGE('',*,*,#60049,.T.);
#89336=ORIENTED_EDGE('',*,*,#60050,.F.);
#89337=ORIENTED_EDGE('',*,*,#60051,.F.);
#89338=ORIENTED_EDGE('',*,*,#60050,.T.);
#89339=ORIENTED_EDGE('',*,*,#60052,.T.);
#89340=ORIENTED_EDGE('',*,*,#60053,.F.);
#89341=ORIENTED_EDGE('',*,*,#60054,.F.);
#89342=ORIENTED_EDGE('',*,*,#60053,.T.);
#89343=ORIENTED_EDGE('',*,*,#60055,.T.);
#89344=ORIENTED_EDGE('',*,*,#60056,.F.);
#89345=ORIENTED_EDGE('',*,*,#60057,.F.);
#89346=ORIENTED_EDGE('',*,*,#60056,.T.);
#89347=ORIENTED_EDGE('',*,*,#60058,.T.);
#89348=ORIENTED_EDGE('',*,*,#60059,.F.);
#89349=ORIENTED_EDGE('',*,*,#60060,.F.);
#89350=ORIENTED_EDGE('',*,*,#60059,.T.);
#89351=ORIENTED_EDGE('',*,*,#60061,.T.);
#89352=ORIENTED_EDGE('',*,*,#60062,.F.);
#89353=ORIENTED_EDGE('',*,*,#60063,.F.);
#89354=ORIENTED_EDGE('',*,*,#60062,.T.);
#89355=ORIENTED_EDGE('',*,*,#60064,.T.);
#89356=ORIENTED_EDGE('',*,*,#60065,.F.);
#89357=ORIENTED_EDGE('',*,*,#60066,.F.);
#89358=ORIENTED_EDGE('',*,*,#60065,.T.);
#89359=ORIENTED_EDGE('',*,*,#60067,.T.);
#89360=ORIENTED_EDGE('',*,*,#60068,.F.);
#89361=ORIENTED_EDGE('',*,*,#60069,.F.);
#89362=ORIENTED_EDGE('',*,*,#60068,.T.);
#89363=ORIENTED_EDGE('',*,*,#60070,.T.);
#89364=ORIENTED_EDGE('',*,*,#59916,.F.);
#89365=ORIENTED_EDGE('',*,*,#60071,.F.);
#89366=ORIENTED_EDGE('',*,*,#60072,.T.);
#89367=ORIENTED_EDGE('',*,*,#60073,.T.);
#89368=ORIENTED_EDGE('',*,*,#60074,.F.);
#89369=ORIENTED_EDGE('',*,*,#60075,.F.);
#89370=ORIENTED_EDGE('',*,*,#60074,.T.);
#89371=ORIENTED_EDGE('',*,*,#60076,.T.);
#89372=ORIENTED_EDGE('',*,*,#60077,.F.);
#89373=ORIENTED_EDGE('',*,*,#60078,.F.);
#89374=ORIENTED_EDGE('',*,*,#60077,.T.);
#89375=ORIENTED_EDGE('',*,*,#60079,.T.);
#89376=ORIENTED_EDGE('',*,*,#60080,.F.);
#89377=ORIENTED_EDGE('',*,*,#60081,.F.);
#89378=ORIENTED_EDGE('',*,*,#60080,.T.);
#89379=ORIENTED_EDGE('',*,*,#60082,.T.);
#89380=ORIENTED_EDGE('',*,*,#60083,.F.);
#89381=ORIENTED_EDGE('',*,*,#60084,.F.);
#89382=ORIENTED_EDGE('',*,*,#60083,.T.);
#89383=ORIENTED_EDGE('',*,*,#60085,.T.);
#89384=ORIENTED_EDGE('',*,*,#60086,.F.);
#89385=ORIENTED_EDGE('',*,*,#60087,.F.);
#89386=ORIENTED_EDGE('',*,*,#60086,.T.);
#89387=ORIENTED_EDGE('',*,*,#60088,.T.);
#89388=ORIENTED_EDGE('',*,*,#60089,.F.);
#89389=ORIENTED_EDGE('',*,*,#60090,.F.);
#89390=ORIENTED_EDGE('',*,*,#60089,.T.);
#89391=ORIENTED_EDGE('',*,*,#60091,.T.);
#89392=ORIENTED_EDGE('',*,*,#60092,.F.);
#89393=ORIENTED_EDGE('',*,*,#60093,.F.);
#89394=ORIENTED_EDGE('',*,*,#60092,.T.);
#89395=ORIENTED_EDGE('',*,*,#60094,.T.);
#89396=ORIENTED_EDGE('',*,*,#60095,.F.);
#89397=ORIENTED_EDGE('',*,*,#60096,.F.);
#89398=ORIENTED_EDGE('',*,*,#60095,.T.);
#89399=ORIENTED_EDGE('',*,*,#60097,.T.);
#89400=ORIENTED_EDGE('',*,*,#60098,.F.);
#89401=ORIENTED_EDGE('',*,*,#60099,.F.);
#89402=ORIENTED_EDGE('',*,*,#60098,.T.);
#89403=ORIENTED_EDGE('',*,*,#60100,.T.);
#89404=ORIENTED_EDGE('',*,*,#60101,.F.);
#89405=ORIENTED_EDGE('',*,*,#60102,.F.);
#89406=ORIENTED_EDGE('',*,*,#60101,.T.);
#89407=ORIENTED_EDGE('',*,*,#60103,.T.);
#89408=ORIENTED_EDGE('',*,*,#60104,.F.);
#89409=ORIENTED_EDGE('',*,*,#60105,.F.);
#89410=ORIENTED_EDGE('',*,*,#60104,.T.);
#89411=ORIENTED_EDGE('',*,*,#60106,.T.);
#89412=ORIENTED_EDGE('',*,*,#60107,.F.);
#89413=ORIENTED_EDGE('',*,*,#60108,.F.);
#89414=ORIENTED_EDGE('',*,*,#60107,.T.);
#89415=ORIENTED_EDGE('',*,*,#60109,.T.);
#89416=ORIENTED_EDGE('',*,*,#59955,.F.);
#89417=ORIENTED_EDGE('',*,*,#60110,.F.);
#89418=ORIENTED_EDGE('',*,*,#60111,.T.);
#89419=ORIENTED_EDGE('',*,*,#60112,.T.);
#89420=ORIENTED_EDGE('',*,*,#60113,.F.);
#89421=ORIENTED_EDGE('',*,*,#60114,.F.);
#89422=ORIENTED_EDGE('',*,*,#60113,.T.);
#89423=ORIENTED_EDGE('',*,*,#60115,.T.);
#89424=ORIENTED_EDGE('',*,*,#60116,.F.);
#89425=ORIENTED_EDGE('',*,*,#60117,.F.);
#89426=ORIENTED_EDGE('',*,*,#60116,.T.);
#89427=ORIENTED_EDGE('',*,*,#60118,.T.);
#89428=ORIENTED_EDGE('',*,*,#60119,.F.);
#89429=ORIENTED_EDGE('',*,*,#60120,.F.);
#89430=ORIENTED_EDGE('',*,*,#60119,.T.);
#89431=ORIENTED_EDGE('',*,*,#60121,.T.);
#89432=ORIENTED_EDGE('',*,*,#60122,.F.);
#89433=ORIENTED_EDGE('',*,*,#60123,.F.);
#89434=ORIENTED_EDGE('',*,*,#60122,.T.);
#89435=ORIENTED_EDGE('',*,*,#60124,.T.);
#89436=ORIENTED_EDGE('',*,*,#60125,.F.);
#89437=ORIENTED_EDGE('',*,*,#60126,.F.);
#89438=ORIENTED_EDGE('',*,*,#60125,.T.);
#89439=ORIENTED_EDGE('',*,*,#60127,.T.);
#89440=ORIENTED_EDGE('',*,*,#60128,.F.);
#89441=ORIENTED_EDGE('',*,*,#60129,.F.);
#89442=ORIENTED_EDGE('',*,*,#60128,.T.);
#89443=ORIENTED_EDGE('',*,*,#60130,.T.);
#89444=ORIENTED_EDGE('',*,*,#60131,.F.);
#89445=ORIENTED_EDGE('',*,*,#60132,.F.);
#89446=ORIENTED_EDGE('',*,*,#60131,.T.);
#89447=ORIENTED_EDGE('',*,*,#60133,.T.);
#89448=ORIENTED_EDGE('',*,*,#60134,.F.);
#89449=ORIENTED_EDGE('',*,*,#60135,.F.);
#89450=ORIENTED_EDGE('',*,*,#60134,.T.);
#89451=ORIENTED_EDGE('',*,*,#60136,.T.);
#89452=ORIENTED_EDGE('',*,*,#60137,.F.);
#89453=ORIENTED_EDGE('',*,*,#60138,.F.);
#89454=ORIENTED_EDGE('',*,*,#60137,.T.);
#89455=ORIENTED_EDGE('',*,*,#60139,.T.);
#89456=ORIENTED_EDGE('',*,*,#60140,.F.);
#89457=ORIENTED_EDGE('',*,*,#60141,.F.);
#89458=ORIENTED_EDGE('',*,*,#60140,.T.);
#89459=ORIENTED_EDGE('',*,*,#60142,.T.);
#89460=ORIENTED_EDGE('',*,*,#60143,.F.);
#89461=ORIENTED_EDGE('',*,*,#60144,.F.);
#89462=ORIENTED_EDGE('',*,*,#60143,.T.);
#89463=ORIENTED_EDGE('',*,*,#60145,.T.);
#89464=ORIENTED_EDGE('',*,*,#60146,.F.);
#89465=ORIENTED_EDGE('',*,*,#60147,.F.);
#89466=ORIENTED_EDGE('',*,*,#60146,.T.);
#89467=ORIENTED_EDGE('',*,*,#60148,.T.);
#89468=ORIENTED_EDGE('',*,*,#60149,.F.);
#89469=ORIENTED_EDGE('',*,*,#60150,.F.);
#89470=ORIENTED_EDGE('',*,*,#60149,.T.);
#89471=ORIENTED_EDGE('',*,*,#60151,.T.);
#89472=ORIENTED_EDGE('',*,*,#60152,.F.);
#89473=ORIENTED_EDGE('',*,*,#60153,.F.);
#89474=ORIENTED_EDGE('',*,*,#60152,.T.);
#89475=ORIENTED_EDGE('',*,*,#60154,.T.);
#89476=ORIENTED_EDGE('',*,*,#60155,.F.);
#89477=ORIENTED_EDGE('',*,*,#60156,.F.);
#89478=ORIENTED_EDGE('',*,*,#60155,.T.);
#89479=ORIENTED_EDGE('',*,*,#60157,.T.);
#89480=ORIENTED_EDGE('',*,*,#60158,.F.);
#89481=ORIENTED_EDGE('',*,*,#60159,.F.);
#89482=ORIENTED_EDGE('',*,*,#60158,.T.);
#89483=ORIENTED_EDGE('',*,*,#60160,.T.);
#89484=ORIENTED_EDGE('',*,*,#60161,.F.);
#89485=ORIENTED_EDGE('',*,*,#60162,.F.);
#89486=ORIENTED_EDGE('',*,*,#60161,.T.);
#89487=ORIENTED_EDGE('',*,*,#60163,.T.);
#89488=ORIENTED_EDGE('',*,*,#60164,.F.);
#89489=ORIENTED_EDGE('',*,*,#60165,.F.);
#89490=ORIENTED_EDGE('',*,*,#60164,.T.);
#89491=ORIENTED_EDGE('',*,*,#60166,.T.);
#89492=ORIENTED_EDGE('',*,*,#60167,.F.);
#89493=ORIENTED_EDGE('',*,*,#60168,.F.);
#89494=ORIENTED_EDGE('',*,*,#60167,.T.);
#89495=ORIENTED_EDGE('',*,*,#60169,.T.);
#89496=ORIENTED_EDGE('',*,*,#60170,.F.);
#89497=ORIENTED_EDGE('',*,*,#60171,.F.);
#89498=ORIENTED_EDGE('',*,*,#60170,.T.);
#89499=ORIENTED_EDGE('',*,*,#60172,.T.);
#89500=ORIENTED_EDGE('',*,*,#60173,.F.);
#89501=ORIENTED_EDGE('',*,*,#60174,.F.);
#89502=ORIENTED_EDGE('',*,*,#60173,.T.);
#89503=ORIENTED_EDGE('',*,*,#60175,.T.);
#89504=ORIENTED_EDGE('',*,*,#60176,.F.);
#89505=ORIENTED_EDGE('',*,*,#60177,.F.);
#89506=ORIENTED_EDGE('',*,*,#60176,.T.);
#89507=ORIENTED_EDGE('',*,*,#60178,.T.);
#89508=ORIENTED_EDGE('',*,*,#60179,.F.);
#89509=ORIENTED_EDGE('',*,*,#60180,.F.);
#89510=ORIENTED_EDGE('',*,*,#60179,.T.);
#89511=ORIENTED_EDGE('',*,*,#60181,.T.);
#89512=ORIENTED_EDGE('',*,*,#60182,.F.);
#89513=ORIENTED_EDGE('',*,*,#60183,.F.);
#89514=ORIENTED_EDGE('',*,*,#60182,.T.);
#89515=ORIENTED_EDGE('',*,*,#60184,.T.);
#89516=ORIENTED_EDGE('',*,*,#60185,.F.);
#89517=ORIENTED_EDGE('',*,*,#60186,.F.);
#89518=ORIENTED_EDGE('',*,*,#60185,.T.);
#89519=ORIENTED_EDGE('',*,*,#60187,.T.);
#89520=ORIENTED_EDGE('',*,*,#60188,.F.);
#89521=ORIENTED_EDGE('',*,*,#60189,.F.);
#89522=ORIENTED_EDGE('',*,*,#60188,.T.);
#89523=ORIENTED_EDGE('',*,*,#60190,.T.);
#89524=ORIENTED_EDGE('',*,*,#60191,.F.);
#89525=ORIENTED_EDGE('',*,*,#60192,.F.);
#89526=ORIENTED_EDGE('',*,*,#60191,.T.);
#89527=ORIENTED_EDGE('',*,*,#60193,.T.);
#89528=ORIENTED_EDGE('',*,*,#60194,.F.);
#89529=ORIENTED_EDGE('',*,*,#60195,.F.);
#89530=ORIENTED_EDGE('',*,*,#60194,.T.);
#89531=ORIENTED_EDGE('',*,*,#60196,.T.);
#89532=ORIENTED_EDGE('',*,*,#60197,.F.);
#89533=ORIENTED_EDGE('',*,*,#60198,.F.);
#89534=ORIENTED_EDGE('',*,*,#60197,.T.);
#89535=ORIENTED_EDGE('',*,*,#60199,.T.);
#89536=ORIENTED_EDGE('',*,*,#60200,.F.);
#89537=ORIENTED_EDGE('',*,*,#60201,.F.);
#89538=ORIENTED_EDGE('',*,*,#60200,.T.);
#89539=ORIENTED_EDGE('',*,*,#60202,.T.);
#89540=ORIENTED_EDGE('',*,*,#60203,.F.);
#89541=ORIENTED_EDGE('',*,*,#60204,.F.);
#89542=ORIENTED_EDGE('',*,*,#60203,.T.);
#89543=ORIENTED_EDGE('',*,*,#60205,.T.);
#89544=ORIENTED_EDGE('',*,*,#60206,.F.);
#89545=ORIENTED_EDGE('',*,*,#60207,.F.);
#89546=ORIENTED_EDGE('',*,*,#60206,.T.);
#89547=ORIENTED_EDGE('',*,*,#60208,.T.);
#89548=ORIENTED_EDGE('',*,*,#60209,.F.);
#89549=ORIENTED_EDGE('',*,*,#60210,.F.);
#89550=ORIENTED_EDGE('',*,*,#60209,.T.);
#89551=ORIENTED_EDGE('',*,*,#60211,.T.);
#89552=ORIENTED_EDGE('',*,*,#60212,.F.);
#89553=ORIENTED_EDGE('',*,*,#60213,.F.);
#89554=ORIENTED_EDGE('',*,*,#60212,.T.);
#89555=ORIENTED_EDGE('',*,*,#60214,.T.);
#89556=ORIENTED_EDGE('',*,*,#60215,.F.);
#89557=ORIENTED_EDGE('',*,*,#60216,.F.);
#89558=ORIENTED_EDGE('',*,*,#60215,.T.);
#89559=ORIENTED_EDGE('',*,*,#60217,.T.);
#89560=ORIENTED_EDGE('',*,*,#60218,.F.);
#89561=ORIENTED_EDGE('',*,*,#60219,.F.);
#89562=ORIENTED_EDGE('',*,*,#60218,.T.);
#89563=ORIENTED_EDGE('',*,*,#60220,.T.);
#89564=ORIENTED_EDGE('',*,*,#60221,.F.);
#89565=ORIENTED_EDGE('',*,*,#60222,.F.);
#89566=ORIENTED_EDGE('',*,*,#60221,.T.);
#89567=ORIENTED_EDGE('',*,*,#60223,.T.);
#89568=ORIENTED_EDGE('',*,*,#60224,.F.);
#89569=ORIENTED_EDGE('',*,*,#60225,.F.);
#89570=ORIENTED_EDGE('',*,*,#60224,.T.);
#89571=ORIENTED_EDGE('',*,*,#60226,.T.);
#89572=ORIENTED_EDGE('',*,*,#60072,.F.);
#89573=ORIENTED_EDGE('',*,*,#60227,.F.);
#89574=ORIENTED_EDGE('',*,*,#60228,.T.);
#89575=ORIENTED_EDGE('',*,*,#60229,.T.);
#89576=ORIENTED_EDGE('',*,*,#60230,.F.);
#89577=ORIENTED_EDGE('',*,*,#60231,.F.);
#89578=ORIENTED_EDGE('',*,*,#60230,.T.);
#89579=ORIENTED_EDGE('',*,*,#60232,.T.);
#89580=ORIENTED_EDGE('',*,*,#60233,.F.);
#89581=ORIENTED_EDGE('',*,*,#60234,.F.);
#89582=ORIENTED_EDGE('',*,*,#60233,.T.);
#89583=ORIENTED_EDGE('',*,*,#60235,.T.);
#89584=ORIENTED_EDGE('',*,*,#60236,.F.);
#89585=ORIENTED_EDGE('',*,*,#60237,.F.);
#89586=ORIENTED_EDGE('',*,*,#60236,.T.);
#89587=ORIENTED_EDGE('',*,*,#60238,.T.);
#89588=ORIENTED_EDGE('',*,*,#60239,.F.);
#89589=ORIENTED_EDGE('',*,*,#60240,.F.);
#89590=ORIENTED_EDGE('',*,*,#60239,.T.);
#89591=ORIENTED_EDGE('',*,*,#60241,.T.);
#89592=ORIENTED_EDGE('',*,*,#60242,.F.);
#89593=ORIENTED_EDGE('',*,*,#60243,.F.);
#89594=ORIENTED_EDGE('',*,*,#60242,.T.);
#89595=ORIENTED_EDGE('',*,*,#60244,.T.);
#89596=ORIENTED_EDGE('',*,*,#60245,.F.);
#89597=ORIENTED_EDGE('',*,*,#60246,.F.);
#89598=ORIENTED_EDGE('',*,*,#60245,.T.);
#89599=ORIENTED_EDGE('',*,*,#60247,.T.);
#89600=ORIENTED_EDGE('',*,*,#60248,.F.);
#89601=ORIENTED_EDGE('',*,*,#60249,.F.);
#89602=ORIENTED_EDGE('',*,*,#60248,.T.);
#89603=ORIENTED_EDGE('',*,*,#60250,.T.);
#89604=ORIENTED_EDGE('',*,*,#60251,.F.);
#89605=ORIENTED_EDGE('',*,*,#60252,.F.);
#89606=ORIENTED_EDGE('',*,*,#60251,.T.);
#89607=ORIENTED_EDGE('',*,*,#60253,.T.);
#89608=ORIENTED_EDGE('',*,*,#60254,.F.);
#89609=ORIENTED_EDGE('',*,*,#60255,.F.);
#89610=ORIENTED_EDGE('',*,*,#60254,.T.);
#89611=ORIENTED_EDGE('',*,*,#60256,.T.);
#89612=ORIENTED_EDGE('',*,*,#60257,.F.);
#89613=ORIENTED_EDGE('',*,*,#60258,.F.);
#89614=ORIENTED_EDGE('',*,*,#60257,.T.);
#89615=ORIENTED_EDGE('',*,*,#60259,.T.);
#89616=ORIENTED_EDGE('',*,*,#60260,.F.);
#89617=ORIENTED_EDGE('',*,*,#60261,.F.);
#89618=ORIENTED_EDGE('',*,*,#60260,.T.);
#89619=ORIENTED_EDGE('',*,*,#60262,.T.);
#89620=ORIENTED_EDGE('',*,*,#60263,.F.);
#89621=ORIENTED_EDGE('',*,*,#60264,.F.);
#89622=ORIENTED_EDGE('',*,*,#60263,.T.);
#89623=ORIENTED_EDGE('',*,*,#60265,.T.);
#89624=ORIENTED_EDGE('',*,*,#60111,.F.);
#89625=ORIENTED_EDGE('',*,*,#60266,.F.);
#89626=ORIENTED_EDGE('',*,*,#59797,.T.);
#89627=ORIENTED_EDGE('',*,*,#60267,.T.);
#89628=ORIENTED_EDGE('',*,*,#60268,.F.);
#89629=ORIENTED_EDGE('',*,*,#60269,.F.);
#89630=ORIENTED_EDGE('',*,*,#60268,.T.);
#89631=ORIENTED_EDGE('',*,*,#60270,.T.);
#89632=ORIENTED_EDGE('',*,*,#60271,.F.);
#89633=ORIENTED_EDGE('',*,*,#60272,.F.);
#89634=ORIENTED_EDGE('',*,*,#60271,.T.);
#89635=ORIENTED_EDGE('',*,*,#60273,.T.);
#89636=ORIENTED_EDGE('',*,*,#60274,.F.);
#89637=ORIENTED_EDGE('',*,*,#60275,.F.);
#89638=ORIENTED_EDGE('',*,*,#60274,.T.);
#89639=ORIENTED_EDGE('',*,*,#60276,.T.);
#89640=ORIENTED_EDGE('',*,*,#60277,.F.);
#89641=ORIENTED_EDGE('',*,*,#60278,.F.);
#89642=ORIENTED_EDGE('',*,*,#60277,.T.);
#89643=ORIENTED_EDGE('',*,*,#60279,.T.);
#89644=ORIENTED_EDGE('',*,*,#60280,.F.);
#89645=ORIENTED_EDGE('',*,*,#60281,.F.);
#89646=ORIENTED_EDGE('',*,*,#60280,.T.);
#89647=ORIENTED_EDGE('',*,*,#60282,.T.);
#89648=ORIENTED_EDGE('',*,*,#60283,.F.);
#89649=ORIENTED_EDGE('',*,*,#60284,.F.);
#89650=ORIENTED_EDGE('',*,*,#60283,.T.);
#89651=ORIENTED_EDGE('',*,*,#60285,.T.);
#89652=ORIENTED_EDGE('',*,*,#60286,.F.);
#89653=ORIENTED_EDGE('',*,*,#60287,.F.);
#89654=ORIENTED_EDGE('',*,*,#60286,.T.);
#89655=ORIENTED_EDGE('',*,*,#60288,.T.);
#89656=ORIENTED_EDGE('',*,*,#60289,.F.);
#89657=ORIENTED_EDGE('',*,*,#60290,.F.);
#89658=ORIENTED_EDGE('',*,*,#60289,.T.);
#89659=ORIENTED_EDGE('',*,*,#60291,.T.);
#89660=ORIENTED_EDGE('',*,*,#60292,.F.);
#89661=ORIENTED_EDGE('',*,*,#60293,.F.);
#89662=ORIENTED_EDGE('',*,*,#60292,.T.);
#89663=ORIENTED_EDGE('',*,*,#60294,.T.);
#89664=ORIENTED_EDGE('',*,*,#60295,.F.);
#89665=ORIENTED_EDGE('',*,*,#60296,.F.);
#89666=ORIENTED_EDGE('',*,*,#60295,.T.);
#89667=ORIENTED_EDGE('',*,*,#60297,.T.);
#89668=ORIENTED_EDGE('',*,*,#60298,.F.);
#89669=ORIENTED_EDGE('',*,*,#60299,.F.);
#89670=ORIENTED_EDGE('',*,*,#60298,.T.);
#89671=ORIENTED_EDGE('',*,*,#60300,.T.);
#89672=ORIENTED_EDGE('',*,*,#60301,.F.);
#89673=ORIENTED_EDGE('',*,*,#60302,.F.);
#89674=ORIENTED_EDGE('',*,*,#60301,.T.);
#89675=ORIENTED_EDGE('',*,*,#60303,.T.);
#89676=ORIENTED_EDGE('',*,*,#60304,.F.);
#89677=ORIENTED_EDGE('',*,*,#60305,.F.);
#89678=ORIENTED_EDGE('',*,*,#60304,.T.);
#89679=ORIENTED_EDGE('',*,*,#60306,.T.);
#89680=ORIENTED_EDGE('',*,*,#60307,.F.);
#89681=ORIENTED_EDGE('',*,*,#60308,.F.);
#89682=ORIENTED_EDGE('',*,*,#60307,.T.);
#89683=ORIENTED_EDGE('',*,*,#60309,.T.);
#89684=ORIENTED_EDGE('',*,*,#60310,.F.);
#89685=ORIENTED_EDGE('',*,*,#60311,.F.);
#89686=ORIENTED_EDGE('',*,*,#60310,.T.);
#89687=ORIENTED_EDGE('',*,*,#60312,.T.);
#89688=ORIENTED_EDGE('',*,*,#60313,.F.);
#89689=ORIENTED_EDGE('',*,*,#60314,.F.);
#89690=ORIENTED_EDGE('',*,*,#60313,.T.);
#89691=ORIENTED_EDGE('',*,*,#60315,.T.);
#89692=ORIENTED_EDGE('',*,*,#60316,.F.);
#89693=ORIENTED_EDGE('',*,*,#60317,.F.);
#89694=ORIENTED_EDGE('',*,*,#60316,.T.);
#89695=ORIENTED_EDGE('',*,*,#60318,.T.);
#89696=ORIENTED_EDGE('',*,*,#60319,.F.);
#89697=ORIENTED_EDGE('',*,*,#60320,.F.);
#89698=ORIENTED_EDGE('',*,*,#60319,.T.);
#89699=ORIENTED_EDGE('',*,*,#60321,.T.);
#89700=ORIENTED_EDGE('',*,*,#60322,.F.);
#89701=ORIENTED_EDGE('',*,*,#60323,.F.);
#89702=ORIENTED_EDGE('',*,*,#60322,.T.);
#89703=ORIENTED_EDGE('',*,*,#60324,.T.);
#89704=ORIENTED_EDGE('',*,*,#60325,.F.);
#89705=ORIENTED_EDGE('',*,*,#60326,.F.);
#89706=ORIENTED_EDGE('',*,*,#60325,.T.);
#89707=ORIENTED_EDGE('',*,*,#60327,.T.);
#89708=ORIENTED_EDGE('',*,*,#60328,.F.);
#89709=ORIENTED_EDGE('',*,*,#60329,.F.);
#89710=ORIENTED_EDGE('',*,*,#60328,.T.);
#89711=ORIENTED_EDGE('',*,*,#60330,.T.);
#89712=ORIENTED_EDGE('',*,*,#60331,.F.);
#89713=ORIENTED_EDGE('',*,*,#60332,.F.);
#89714=ORIENTED_EDGE('',*,*,#60331,.T.);
#89715=ORIENTED_EDGE('',*,*,#60333,.T.);
#89716=ORIENTED_EDGE('',*,*,#60334,.F.);
#89717=ORIENTED_EDGE('',*,*,#60335,.F.);
#89718=ORIENTED_EDGE('',*,*,#60334,.T.);
#89719=ORIENTED_EDGE('',*,*,#60336,.T.);
#89720=ORIENTED_EDGE('',*,*,#60337,.F.);
#89721=ORIENTED_EDGE('',*,*,#60338,.F.);
#89722=ORIENTED_EDGE('',*,*,#60337,.T.);
#89723=ORIENTED_EDGE('',*,*,#60339,.T.);
#89724=ORIENTED_EDGE('',*,*,#60340,.F.);
#89725=ORIENTED_EDGE('',*,*,#60341,.F.);
#89726=ORIENTED_EDGE('',*,*,#60340,.T.);
#89727=ORIENTED_EDGE('',*,*,#60342,.T.);
#89728=ORIENTED_EDGE('',*,*,#60343,.F.);
#89729=ORIENTED_EDGE('',*,*,#60344,.F.);
#89730=ORIENTED_EDGE('',*,*,#60343,.T.);
#89731=ORIENTED_EDGE('',*,*,#60345,.T.);
#89732=ORIENTED_EDGE('',*,*,#60346,.F.);
#89733=ORIENTED_EDGE('',*,*,#60347,.F.);
#89734=ORIENTED_EDGE('',*,*,#60346,.T.);
#89735=ORIENTED_EDGE('',*,*,#60348,.T.);
#89736=ORIENTED_EDGE('',*,*,#60349,.F.);
#89737=ORIENTED_EDGE('',*,*,#60350,.F.);
#89738=ORIENTED_EDGE('',*,*,#60349,.T.);
#89739=ORIENTED_EDGE('',*,*,#60351,.T.);
#89740=ORIENTED_EDGE('',*,*,#60352,.F.);
#89741=ORIENTED_EDGE('',*,*,#60353,.F.);
#89742=ORIENTED_EDGE('',*,*,#60352,.T.);
#89743=ORIENTED_EDGE('',*,*,#60354,.T.);
#89744=ORIENTED_EDGE('',*,*,#60355,.F.);
#89745=ORIENTED_EDGE('',*,*,#60356,.F.);
#89746=ORIENTED_EDGE('',*,*,#60355,.T.);
#89747=ORIENTED_EDGE('',*,*,#60357,.T.);
#89748=ORIENTED_EDGE('',*,*,#60358,.F.);
#89749=ORIENTED_EDGE('',*,*,#60359,.F.);
#89750=ORIENTED_EDGE('',*,*,#60358,.T.);
#89751=ORIENTED_EDGE('',*,*,#60360,.T.);
#89752=ORIENTED_EDGE('',*,*,#60361,.F.);
#89753=ORIENTED_EDGE('',*,*,#60362,.F.);
#89754=ORIENTED_EDGE('',*,*,#60361,.T.);
#89755=ORIENTED_EDGE('',*,*,#60363,.T.);
#89756=ORIENTED_EDGE('',*,*,#60364,.F.);
#89757=ORIENTED_EDGE('',*,*,#60365,.F.);
#89758=ORIENTED_EDGE('',*,*,#60364,.T.);
#89759=ORIENTED_EDGE('',*,*,#60366,.T.);
#89760=ORIENTED_EDGE('',*,*,#60367,.F.);
#89761=ORIENTED_EDGE('',*,*,#60368,.F.);
#89762=ORIENTED_EDGE('',*,*,#60367,.T.);
#89763=ORIENTED_EDGE('',*,*,#60369,.T.);
#89764=ORIENTED_EDGE('',*,*,#60370,.F.);
#89765=ORIENTED_EDGE('',*,*,#60371,.F.);
#89766=ORIENTED_EDGE('',*,*,#60370,.T.);
#89767=ORIENTED_EDGE('',*,*,#60372,.T.);
#89768=ORIENTED_EDGE('',*,*,#60373,.F.);
#89769=ORIENTED_EDGE('',*,*,#60374,.F.);
#89770=ORIENTED_EDGE('',*,*,#60373,.T.);
#89771=ORIENTED_EDGE('',*,*,#60375,.T.);
#89772=ORIENTED_EDGE('',*,*,#60376,.F.);
#89773=ORIENTED_EDGE('',*,*,#60377,.F.);
#89774=ORIENTED_EDGE('',*,*,#60376,.T.);
#89775=ORIENTED_EDGE('',*,*,#60378,.T.);
#89776=ORIENTED_EDGE('',*,*,#60228,.F.);
#89777=ORIENTED_EDGE('',*,*,#60379,.F.);
#89778=ORIENTED_EDGE('',*,*,#60380,.F.);
#89779=ORIENTED_EDGE('',*,*,#60381,.T.);
#89780=ORIENTED_EDGE('',*,*,#59752,.F.);
#89781=ORIENTED_EDGE('',*,*,#60382,.F.);
#89782=ORIENTED_EDGE('',*,*,#59897,.F.);
#89783=ORIENTED_EDGE('',*,*,#60383,.T.);
#89784=ORIENTED_EDGE('',*,*,#60380,.T.);
#89785=ORIENTED_EDGE('',*,*,#60384,.F.);
#89786=ORIENTED_EDGE('',*,*,#59750,.F.);
#89787=ORIENTED_EDGE('',*,*,#60385,.T.);
#89788=ORIENTED_EDGE('',*,*,#60386,.T.);
#89789=ORIENTED_EDGE('',*,*,#60387,.F.);
#89790=ORIENTED_EDGE('',*,*,#60386,.F.);
#89791=ORIENTED_EDGE('',*,*,#60388,.T.);
#89792=ORIENTED_EDGE('',*,*,#59859,.F.);
#89793=ORIENTED_EDGE('',*,*,#60389,.F.);
#89794=ORIENTED_EDGE('',*,*,#60390,.F.);
#89795=ORIENTED_EDGE('',*,*,#60391,.F.);
#89796=ORIENTED_EDGE('',*,*,#60392,.T.);
#89797=ORIENTED_EDGE('',*,*,#60393,.F.);
#89798=ORIENTED_EDGE('',*,*,#60394,.T.);
#89799=ORIENTED_EDGE('',*,*,#60395,.T.);
#89800=ORIENTED_EDGE('',*,*,#60396,.F.);
#89801=ORIENTED_EDGE('',*,*,#60397,.F.);
#89802=ORIENTED_EDGE('',*,*,#60398,.F.);
#89803=ORIENTED_EDGE('',*,*,#60396,.T.);
#89804=ORIENTED_EDGE('',*,*,#60399,.T.);
#89805=ORIENTED_EDGE('',*,*,#60400,.T.);
#89806=ORIENTED_EDGE('',*,*,#60399,.F.);
#89807=ORIENTED_EDGE('',*,*,#60395,.F.);
#89808=ORIENTED_EDGE('',*,*,#60401,.T.);
#89809=ORIENTED_EDGE('',*,*,#60402,.T.);
#89810=ORIENTED_EDGE('',*,*,#60401,.F.);
#89811=ORIENTED_EDGE('',*,*,#60394,.F.);
#89812=ORIENTED_EDGE('',*,*,#60403,.T.);
#89813=ORIENTED_EDGE('',*,*,#60404,.F.);
#89814=ORIENTED_EDGE('',*,*,#60403,.F.);
#89815=ORIENTED_EDGE('',*,*,#60393,.T.);
#89816=ORIENTED_EDGE('',*,*,#60405,.T.);
#89817=ORIENTED_EDGE('',*,*,#60406,.T.);
#89818=ORIENTED_EDGE('',*,*,#60405,.F.);
#89819=ORIENTED_EDGE('',*,*,#60392,.F.);
#89820=ORIENTED_EDGE('',*,*,#60407,.T.);
#89821=ORIENTED_EDGE('',*,*,#60408,.F.);
#89822=ORIENTED_EDGE('',*,*,#60407,.F.);
#89823=ORIENTED_EDGE('',*,*,#60391,.T.);
#89824=ORIENTED_EDGE('',*,*,#60409,.T.);
#89825=ORIENTED_EDGE('',*,*,#60410,.F.);
#89826=ORIENTED_EDGE('',*,*,#60409,.F.);
#89827=ORIENTED_EDGE('',*,*,#60390,.T.);
#89828=ORIENTED_EDGE('',*,*,#60411,.T.);
#89829=ORIENTED_EDGE('',*,*,#60412,.F.);
#89830=ORIENTED_EDGE('',*,*,#60411,.F.);
#89831=ORIENTED_EDGE('',*,*,#60389,.T.);
#89832=ORIENTED_EDGE('',*,*,#60398,.T.);
#89833=ORIENTED_EDGE('',*,*,#60412,.T.);
#89834=ORIENTED_EDGE('',*,*,#60397,.T.);
#89835=ORIENTED_EDGE('',*,*,#60400,.F.);
#89836=ORIENTED_EDGE('',*,*,#60402,.F.);
#89837=ORIENTED_EDGE('',*,*,#60404,.T.);
#89838=ORIENTED_EDGE('',*,*,#60406,.F.);
#89839=ORIENTED_EDGE('',*,*,#60408,.T.);
#89840=ORIENTED_EDGE('',*,*,#60410,.T.);
#89841=ORIENTED_EDGE('',*,*,#59893,.F.);
#89842=ORIENTED_EDGE('',*,*,#59890,.F.);
#89843=ORIENTED_EDGE('',*,*,#59887,.F.);
#89844=ORIENTED_EDGE('',*,*,#59884,.F.);
#89845=ORIENTED_EDGE('',*,*,#59881,.F.);
#89846=ORIENTED_EDGE('',*,*,#59878,.F.);
#89847=ORIENTED_EDGE('',*,*,#59875,.F.);
#89848=ORIENTED_EDGE('',*,*,#59872,.F.);
#89849=ORIENTED_EDGE('',*,*,#59869,.F.);
#89850=ORIENTED_EDGE('',*,*,#59866,.F.);
#89851=ORIENTED_EDGE('',*,*,#59863,.F.);
#89852=ORIENTED_EDGE('',*,*,#59860,.F.);
#89853=ORIENTED_EDGE('',*,*,#60388,.F.);
#89854=ORIENTED_EDGE('',*,*,#60385,.F.);
#89855=ORIENTED_EDGE('',*,*,#59749,.F.);
#89856=ORIENTED_EDGE('',*,*,#59857,.F.);
#89857=ORIENTED_EDGE('',*,*,#59854,.F.);
#89858=ORIENTED_EDGE('',*,*,#59851,.F.);
#89859=ORIENTED_EDGE('',*,*,#59848,.F.);
#89860=ORIENTED_EDGE('',*,*,#59845,.F.);
#89861=ORIENTED_EDGE('',*,*,#59842,.F.);
#89862=ORIENTED_EDGE('',*,*,#59839,.F.);
#89863=ORIENTED_EDGE('',*,*,#59836,.F.);
#89864=ORIENTED_EDGE('',*,*,#59833,.F.);
#89865=ORIENTED_EDGE('',*,*,#59830,.F.);
#89866=ORIENTED_EDGE('',*,*,#59827,.F.);
#89867=ORIENTED_EDGE('',*,*,#59824,.F.);
#89868=ORIENTED_EDGE('',*,*,#59821,.F.);
#89869=ORIENTED_EDGE('',*,*,#59818,.F.);
#89870=ORIENTED_EDGE('',*,*,#59815,.F.);
#89871=ORIENTED_EDGE('',*,*,#59812,.F.);
#89872=ORIENTED_EDGE('',*,*,#59809,.F.);
#89873=ORIENTED_EDGE('',*,*,#59806,.F.);
#89874=ORIENTED_EDGE('',*,*,#59803,.F.);
#89875=ORIENTED_EDGE('',*,*,#59800,.F.);
#89876=ORIENTED_EDGE('',*,*,#59953,.F.);
#89877=ORIENTED_EDGE('',*,*,#59950,.F.);
#89878=ORIENTED_EDGE('',*,*,#59947,.F.);
#89879=ORIENTED_EDGE('',*,*,#59944,.F.);
#89880=ORIENTED_EDGE('',*,*,#59941,.F.);
#89881=ORIENTED_EDGE('',*,*,#59938,.F.);
#89882=ORIENTED_EDGE('',*,*,#59935,.F.);
#89883=ORIENTED_EDGE('',*,*,#59932,.F.);
#89884=ORIENTED_EDGE('',*,*,#59929,.F.);
#89885=ORIENTED_EDGE('',*,*,#59926,.F.);
#89886=ORIENTED_EDGE('',*,*,#59923,.F.);
#89887=ORIENTED_EDGE('',*,*,#59920,.F.);
#89888=ORIENTED_EDGE('',*,*,#59917,.F.);
#89889=ORIENTED_EDGE('',*,*,#60070,.F.);
#89890=ORIENTED_EDGE('',*,*,#60067,.F.);
#89891=ORIENTED_EDGE('',*,*,#60064,.F.);
#89892=ORIENTED_EDGE('',*,*,#60061,.F.);
#89893=ORIENTED_EDGE('',*,*,#60058,.F.);
#89894=ORIENTED_EDGE('',*,*,#60055,.F.);
#89895=ORIENTED_EDGE('',*,*,#60052,.F.);
#89896=ORIENTED_EDGE('',*,*,#60049,.F.);
#89897=ORIENTED_EDGE('',*,*,#60046,.F.);
#89898=ORIENTED_EDGE('',*,*,#60043,.F.);
#89899=ORIENTED_EDGE('',*,*,#60040,.F.);
#89900=ORIENTED_EDGE('',*,*,#60037,.F.);
#89901=ORIENTED_EDGE('',*,*,#60034,.F.);
#89902=ORIENTED_EDGE('',*,*,#60031,.F.);
#89903=ORIENTED_EDGE('',*,*,#60028,.F.);
#89904=ORIENTED_EDGE('',*,*,#60025,.F.);
#89905=ORIENTED_EDGE('',*,*,#60022,.F.);
#89906=ORIENTED_EDGE('',*,*,#60019,.F.);
#89907=ORIENTED_EDGE('',*,*,#60016,.F.);
#89908=ORIENTED_EDGE('',*,*,#60013,.F.);
#89909=ORIENTED_EDGE('',*,*,#60010,.F.);
#89910=ORIENTED_EDGE('',*,*,#60007,.F.);
#89911=ORIENTED_EDGE('',*,*,#60004,.F.);
#89912=ORIENTED_EDGE('',*,*,#60001,.F.);
#89913=ORIENTED_EDGE('',*,*,#59998,.F.);
#89914=ORIENTED_EDGE('',*,*,#59995,.F.);
#89915=ORIENTED_EDGE('',*,*,#59992,.F.);
#89916=ORIENTED_EDGE('',*,*,#59989,.F.);
#89917=ORIENTED_EDGE('',*,*,#59986,.F.);
#89918=ORIENTED_EDGE('',*,*,#59983,.F.);
#89919=ORIENTED_EDGE('',*,*,#59980,.F.);
#89920=ORIENTED_EDGE('',*,*,#59977,.F.);
#89921=ORIENTED_EDGE('',*,*,#59974,.F.);
#89922=ORIENTED_EDGE('',*,*,#59971,.F.);
#89923=ORIENTED_EDGE('',*,*,#59968,.F.);
#89924=ORIENTED_EDGE('',*,*,#59965,.F.);
#89925=ORIENTED_EDGE('',*,*,#59962,.F.);
#89926=ORIENTED_EDGE('',*,*,#59959,.F.);
#89927=ORIENTED_EDGE('',*,*,#59956,.F.);
#89928=ORIENTED_EDGE('',*,*,#60109,.F.);
#89929=ORIENTED_EDGE('',*,*,#60106,.F.);
#89930=ORIENTED_EDGE('',*,*,#60103,.F.);
#89931=ORIENTED_EDGE('',*,*,#60100,.F.);
#89932=ORIENTED_EDGE('',*,*,#60097,.F.);
#89933=ORIENTED_EDGE('',*,*,#60094,.F.);
#89934=ORIENTED_EDGE('',*,*,#60091,.F.);
#89935=ORIENTED_EDGE('',*,*,#60088,.F.);
#89936=ORIENTED_EDGE('',*,*,#60085,.F.);
#89937=ORIENTED_EDGE('',*,*,#60082,.F.);
#89938=ORIENTED_EDGE('',*,*,#60079,.F.);
#89939=ORIENTED_EDGE('',*,*,#60076,.F.);
#89940=ORIENTED_EDGE('',*,*,#60073,.F.);
#89941=ORIENTED_EDGE('',*,*,#60226,.F.);
#89942=ORIENTED_EDGE('',*,*,#60223,.F.);
#89943=ORIENTED_EDGE('',*,*,#60220,.F.);
#89944=ORIENTED_EDGE('',*,*,#60217,.F.);
#89945=ORIENTED_EDGE('',*,*,#60214,.F.);
#89946=ORIENTED_EDGE('',*,*,#60211,.F.);
#89947=ORIENTED_EDGE('',*,*,#60208,.F.);
#89948=ORIENTED_EDGE('',*,*,#60205,.F.);
#89949=ORIENTED_EDGE('',*,*,#60202,.F.);
#89950=ORIENTED_EDGE('',*,*,#60199,.F.);
#89951=ORIENTED_EDGE('',*,*,#60196,.F.);
#89952=ORIENTED_EDGE('',*,*,#60193,.F.);
#89953=ORIENTED_EDGE('',*,*,#60190,.F.);
#89954=ORIENTED_EDGE('',*,*,#60187,.F.);
#89955=ORIENTED_EDGE('',*,*,#60184,.F.);
#89956=ORIENTED_EDGE('',*,*,#60181,.F.);
#89957=ORIENTED_EDGE('',*,*,#60178,.F.);
#89958=ORIENTED_EDGE('',*,*,#60175,.F.);
#89959=ORIENTED_EDGE('',*,*,#60172,.F.);
#89960=ORIENTED_EDGE('',*,*,#60169,.F.);
#89961=ORIENTED_EDGE('',*,*,#60166,.F.);
#89962=ORIENTED_EDGE('',*,*,#60163,.F.);
#89963=ORIENTED_EDGE('',*,*,#60160,.F.);
#89964=ORIENTED_EDGE('',*,*,#60157,.F.);
#89965=ORIENTED_EDGE('',*,*,#60154,.F.);
#89966=ORIENTED_EDGE('',*,*,#60151,.F.);
#89967=ORIENTED_EDGE('',*,*,#60148,.F.);
#89968=ORIENTED_EDGE('',*,*,#60145,.F.);
#89969=ORIENTED_EDGE('',*,*,#60142,.F.);
#89970=ORIENTED_EDGE('',*,*,#60139,.F.);
#89971=ORIENTED_EDGE('',*,*,#60136,.F.);
#89972=ORIENTED_EDGE('',*,*,#60133,.F.);
#89973=ORIENTED_EDGE('',*,*,#60130,.F.);
#89974=ORIENTED_EDGE('',*,*,#60127,.F.);
#89975=ORIENTED_EDGE('',*,*,#60124,.F.);
#89976=ORIENTED_EDGE('',*,*,#60121,.F.);
#89977=ORIENTED_EDGE('',*,*,#60118,.F.);
#89978=ORIENTED_EDGE('',*,*,#60115,.F.);
#89979=ORIENTED_EDGE('',*,*,#60112,.F.);
#89980=ORIENTED_EDGE('',*,*,#60265,.F.);
#89981=ORIENTED_EDGE('',*,*,#60262,.F.);
#89982=ORIENTED_EDGE('',*,*,#60259,.F.);
#89983=ORIENTED_EDGE('',*,*,#60256,.F.);
#89984=ORIENTED_EDGE('',*,*,#60253,.F.);
#89985=ORIENTED_EDGE('',*,*,#60250,.F.);
#89986=ORIENTED_EDGE('',*,*,#60247,.F.);
#89987=ORIENTED_EDGE('',*,*,#60244,.F.);
#89988=ORIENTED_EDGE('',*,*,#60241,.F.);
#89989=ORIENTED_EDGE('',*,*,#60238,.F.);
#89990=ORIENTED_EDGE('',*,*,#60235,.F.);
#89991=ORIENTED_EDGE('',*,*,#60232,.F.);
#89992=ORIENTED_EDGE('',*,*,#60229,.F.);
#89993=ORIENTED_EDGE('',*,*,#60378,.F.);
#89994=ORIENTED_EDGE('',*,*,#60375,.F.);
#89995=ORIENTED_EDGE('',*,*,#60372,.F.);
#89996=ORIENTED_EDGE('',*,*,#60369,.F.);
#89997=ORIENTED_EDGE('',*,*,#60366,.F.);
#89998=ORIENTED_EDGE('',*,*,#60363,.F.);
#89999=ORIENTED_EDGE('',*,*,#60360,.F.);
#90000=ORIENTED_EDGE('',*,*,#60357,.F.);
#90001=ORIENTED_EDGE('',*,*,#60354,.F.);
#90002=ORIENTED_EDGE('',*,*,#60351,.F.);
#90003=ORIENTED_EDGE('',*,*,#60348,.F.);
#90004=ORIENTED_EDGE('',*,*,#60345,.F.);
#90005=ORIENTED_EDGE('',*,*,#60342,.F.);
#90006=ORIENTED_EDGE('',*,*,#60339,.F.);
#90007=ORIENTED_EDGE('',*,*,#60336,.F.);
#90008=ORIENTED_EDGE('',*,*,#60333,.F.);
#90009=ORIENTED_EDGE('',*,*,#60330,.F.);
#90010=ORIENTED_EDGE('',*,*,#60327,.F.);
#90011=ORIENTED_EDGE('',*,*,#60324,.F.);
#90012=ORIENTED_EDGE('',*,*,#60321,.F.);
#90013=ORIENTED_EDGE('',*,*,#60318,.F.);
#90014=ORIENTED_EDGE('',*,*,#60315,.F.);
#90015=ORIENTED_EDGE('',*,*,#60312,.F.);
#90016=ORIENTED_EDGE('',*,*,#60309,.F.);
#90017=ORIENTED_EDGE('',*,*,#60306,.F.);
#90018=ORIENTED_EDGE('',*,*,#60303,.F.);
#90019=ORIENTED_EDGE('',*,*,#60300,.F.);
#90020=ORIENTED_EDGE('',*,*,#60297,.F.);
#90021=ORIENTED_EDGE('',*,*,#60294,.F.);
#90022=ORIENTED_EDGE('',*,*,#60291,.F.);
#90023=ORIENTED_EDGE('',*,*,#60288,.F.);
#90024=ORIENTED_EDGE('',*,*,#60285,.F.);
#90025=ORIENTED_EDGE('',*,*,#60282,.F.);
#90026=ORIENTED_EDGE('',*,*,#60279,.F.);
#90027=ORIENTED_EDGE('',*,*,#60276,.F.);
#90028=ORIENTED_EDGE('',*,*,#60273,.F.);
#90029=ORIENTED_EDGE('',*,*,#60270,.F.);
#90030=ORIENTED_EDGE('',*,*,#60267,.F.);
#90031=ORIENTED_EDGE('',*,*,#59796,.F.);
#90032=ORIENTED_EDGE('',*,*,#59793,.F.);
#90033=ORIENTED_EDGE('',*,*,#59790,.F.);
#90034=ORIENTED_EDGE('',*,*,#59787,.F.);
#90035=ORIENTED_EDGE('',*,*,#59784,.F.);
#90036=ORIENTED_EDGE('',*,*,#59781,.F.);
#90037=ORIENTED_EDGE('',*,*,#59778,.F.);
#90038=ORIENTED_EDGE('',*,*,#59775,.F.);
#90039=ORIENTED_EDGE('',*,*,#59772,.F.);
#90040=ORIENTED_EDGE('',*,*,#59769,.F.);
#90041=ORIENTED_EDGE('',*,*,#59766,.F.);
#90042=ORIENTED_EDGE('',*,*,#59763,.F.);
#90043=ORIENTED_EDGE('',*,*,#59760,.F.);
#90044=ORIENTED_EDGE('',*,*,#59757,.F.);
#90045=ORIENTED_EDGE('',*,*,#59914,.F.);
#90046=ORIENTED_EDGE('',*,*,#59911,.F.);
#90047=ORIENTED_EDGE('',*,*,#59908,.F.);
#90048=ORIENTED_EDGE('',*,*,#59905,.F.);
#90049=ORIENTED_EDGE('',*,*,#59902,.F.);
#90050=ORIENTED_EDGE('',*,*,#59899,.F.);
#90051=ORIENTED_EDGE('',*,*,#59753,.F.);
#90052=ORIENTED_EDGE('',*,*,#60381,.F.);
#90053=ORIENTED_EDGE('',*,*,#60383,.F.);
#90054=ORIENTED_EDGE('',*,*,#59896,.F.);
#90055=ORIENTED_EDGE('',*,*,#60413,.F.);
#90056=ORIENTED_EDGE('',*,*,#60414,.F.);
#90057=ORIENTED_EDGE('',*,*,#60415,.T.);
#90058=ORIENTED_EDGE('',*,*,#60416,.T.);
#90059=ORIENTED_EDGE('',*,*,#60417,.F.);
#90060=ORIENTED_EDGE('',*,*,#60416,.F.);
#90061=ORIENTED_EDGE('',*,*,#60418,.T.);
#90062=ORIENTED_EDGE('',*,*,#60419,.T.);
#90063=ORIENTED_EDGE('',*,*,#60420,.F.);
#90064=ORIENTED_EDGE('',*,*,#60419,.F.);
#90065=ORIENTED_EDGE('',*,*,#60421,.T.);
#90066=ORIENTED_EDGE('',*,*,#60422,.T.);
#90067=ORIENTED_EDGE('',*,*,#60423,.F.);
#90068=ORIENTED_EDGE('',*,*,#60422,.F.);
#90069=ORIENTED_EDGE('',*,*,#60424,.T.);
#90070=ORIENTED_EDGE('',*,*,#60414,.T.);
#90071=ORIENTED_EDGE('',*,*,#60424,.F.);
#90072=ORIENTED_EDGE('',*,*,#60421,.F.);
#90073=ORIENTED_EDGE('',*,*,#60418,.F.);
#90074=ORIENTED_EDGE('',*,*,#60415,.F.);
#90075=ORIENTED_EDGE('',*,*,#59886,.T.);
#90076=ORIENTED_EDGE('',*,*,#59889,.T.);
#90077=ORIENTED_EDGE('',*,*,#59892,.T.);
#90078=ORIENTED_EDGE('',*,*,#59895,.T.);
#90079=ORIENTED_EDGE('',*,*,#60382,.T.);
#90080=ORIENTED_EDGE('',*,*,#60379,.T.);
#90081=ORIENTED_EDGE('',*,*,#59751,.T.);
#90082=ORIENTED_EDGE('',*,*,#59898,.T.);
#90083=ORIENTED_EDGE('',*,*,#59901,.T.);
#90084=ORIENTED_EDGE('',*,*,#59904,.T.);
#90085=ORIENTED_EDGE('',*,*,#59907,.T.);
#90086=ORIENTED_EDGE('',*,*,#59910,.T.);
#90087=ORIENTED_EDGE('',*,*,#59913,.T.);
#90088=ORIENTED_EDGE('',*,*,#59755,.T.);
#90089=ORIENTED_EDGE('',*,*,#59759,.T.);
#90090=ORIENTED_EDGE('',*,*,#59762,.T.);
#90091=ORIENTED_EDGE('',*,*,#59765,.T.);
#90092=ORIENTED_EDGE('',*,*,#59768,.T.);
#90093=ORIENTED_EDGE('',*,*,#59771,.T.);
#90094=ORIENTED_EDGE('',*,*,#59774,.T.);
#90095=ORIENTED_EDGE('',*,*,#59777,.T.);
#90096=ORIENTED_EDGE('',*,*,#59780,.T.);
#90097=ORIENTED_EDGE('',*,*,#59783,.T.);
#90098=ORIENTED_EDGE('',*,*,#59786,.T.);
#90099=ORIENTED_EDGE('',*,*,#59789,.T.);
#90100=ORIENTED_EDGE('',*,*,#59792,.T.);
#90101=ORIENTED_EDGE('',*,*,#59795,.T.);
#90102=ORIENTED_EDGE('',*,*,#60266,.T.);
#90103=ORIENTED_EDGE('',*,*,#60269,.T.);
#90104=ORIENTED_EDGE('',*,*,#60272,.T.);
#90105=ORIENTED_EDGE('',*,*,#60275,.T.);
#90106=ORIENTED_EDGE('',*,*,#60278,.T.);
#90107=ORIENTED_EDGE('',*,*,#60281,.T.);
#90108=ORIENTED_EDGE('',*,*,#60284,.T.);
#90109=ORIENTED_EDGE('',*,*,#60287,.T.);
#90110=ORIENTED_EDGE('',*,*,#60290,.T.);
#90111=ORIENTED_EDGE('',*,*,#60293,.T.);
#90112=ORIENTED_EDGE('',*,*,#60296,.T.);
#90113=ORIENTED_EDGE('',*,*,#60299,.T.);
#90114=ORIENTED_EDGE('',*,*,#60302,.T.);
#90115=ORIENTED_EDGE('',*,*,#60305,.T.);
#90116=ORIENTED_EDGE('',*,*,#60308,.T.);
#90117=ORIENTED_EDGE('',*,*,#60311,.T.);
#90118=ORIENTED_EDGE('',*,*,#60314,.T.);
#90119=ORIENTED_EDGE('',*,*,#60317,.T.);
#90120=ORIENTED_EDGE('',*,*,#60320,.T.);
#90121=ORIENTED_EDGE('',*,*,#60323,.T.);
#90122=ORIENTED_EDGE('',*,*,#60326,.T.);
#90123=ORIENTED_EDGE('',*,*,#60329,.T.);
#90124=ORIENTED_EDGE('',*,*,#60332,.T.);
#90125=ORIENTED_EDGE('',*,*,#60335,.T.);
#90126=ORIENTED_EDGE('',*,*,#60338,.T.);
#90127=ORIENTED_EDGE('',*,*,#60341,.T.);
#90128=ORIENTED_EDGE('',*,*,#60344,.T.);
#90129=ORIENTED_EDGE('',*,*,#60347,.T.);
#90130=ORIENTED_EDGE('',*,*,#60350,.T.);
#90131=ORIENTED_EDGE('',*,*,#60353,.T.);
#90132=ORIENTED_EDGE('',*,*,#60356,.T.);
#90133=ORIENTED_EDGE('',*,*,#60359,.T.);
#90134=ORIENTED_EDGE('',*,*,#60362,.T.);
#90135=ORIENTED_EDGE('',*,*,#60365,.T.);
#90136=ORIENTED_EDGE('',*,*,#60368,.T.);
#90137=ORIENTED_EDGE('',*,*,#60371,.T.);
#90138=ORIENTED_EDGE('',*,*,#60374,.T.);
#90139=ORIENTED_EDGE('',*,*,#60377,.T.);
#90140=ORIENTED_EDGE('',*,*,#60227,.T.);
#90141=ORIENTED_EDGE('',*,*,#60231,.T.);
#90142=ORIENTED_EDGE('',*,*,#60234,.T.);
#90143=ORIENTED_EDGE('',*,*,#60237,.T.);
#90144=ORIENTED_EDGE('',*,*,#60240,.T.);
#90145=ORIENTED_EDGE('',*,*,#60243,.T.);
#90146=ORIENTED_EDGE('',*,*,#60246,.T.);
#90147=ORIENTED_EDGE('',*,*,#60249,.T.);
#90148=ORIENTED_EDGE('',*,*,#60252,.T.);
#90149=ORIENTED_EDGE('',*,*,#60255,.T.);
#90150=ORIENTED_EDGE('',*,*,#60258,.T.);
#90151=ORIENTED_EDGE('',*,*,#60261,.T.);
#90152=ORIENTED_EDGE('',*,*,#60264,.T.);
#90153=ORIENTED_EDGE('',*,*,#60110,.T.);
#90154=ORIENTED_EDGE('',*,*,#60114,.T.);
#90155=ORIENTED_EDGE('',*,*,#60117,.T.);
#90156=ORIENTED_EDGE('',*,*,#60120,.T.);
#90157=ORIENTED_EDGE('',*,*,#60123,.T.);
#90158=ORIENTED_EDGE('',*,*,#60126,.T.);
#90159=ORIENTED_EDGE('',*,*,#60129,.T.);
#90160=ORIENTED_EDGE('',*,*,#60132,.T.);
#90161=ORIENTED_EDGE('',*,*,#60135,.T.);
#90162=ORIENTED_EDGE('',*,*,#60138,.T.);
#90163=ORIENTED_EDGE('',*,*,#60141,.T.);
#90164=ORIENTED_EDGE('',*,*,#60144,.T.);
#90165=ORIENTED_EDGE('',*,*,#60147,.T.);
#90166=ORIENTED_EDGE('',*,*,#60150,.T.);
#90167=ORIENTED_EDGE('',*,*,#60153,.T.);
#90168=ORIENTED_EDGE('',*,*,#60156,.T.);
#90169=ORIENTED_EDGE('',*,*,#60159,.T.);
#90170=ORIENTED_EDGE('',*,*,#60162,.T.);
#90171=ORIENTED_EDGE('',*,*,#60165,.T.);
#90172=ORIENTED_EDGE('',*,*,#60168,.T.);
#90173=ORIENTED_EDGE('',*,*,#60171,.T.);
#90174=ORIENTED_EDGE('',*,*,#60174,.T.);
#90175=ORIENTED_EDGE('',*,*,#60177,.T.);
#90176=ORIENTED_EDGE('',*,*,#60180,.T.);
#90177=ORIENTED_EDGE('',*,*,#60183,.T.);
#90178=ORIENTED_EDGE('',*,*,#60186,.T.);
#90179=ORIENTED_EDGE('',*,*,#60189,.T.);
#90180=ORIENTED_EDGE('',*,*,#60192,.T.);
#90181=ORIENTED_EDGE('',*,*,#60195,.T.);
#90182=ORIENTED_EDGE('',*,*,#60198,.T.);
#90183=ORIENTED_EDGE('',*,*,#60201,.T.);
#90184=ORIENTED_EDGE('',*,*,#60204,.T.);
#90185=ORIENTED_EDGE('',*,*,#60207,.T.);
#90186=ORIENTED_EDGE('',*,*,#60210,.T.);
#90187=ORIENTED_EDGE('',*,*,#60213,.T.);
#90188=ORIENTED_EDGE('',*,*,#60216,.T.);
#90189=ORIENTED_EDGE('',*,*,#60219,.T.);
#90190=ORIENTED_EDGE('',*,*,#60222,.T.);
#90191=ORIENTED_EDGE('',*,*,#60225,.T.);
#90192=ORIENTED_EDGE('',*,*,#60071,.T.);
#90193=ORIENTED_EDGE('',*,*,#60075,.T.);
#90194=ORIENTED_EDGE('',*,*,#60078,.T.);
#90195=ORIENTED_EDGE('',*,*,#60081,.T.);
#90196=ORIENTED_EDGE('',*,*,#60084,.T.);
#90197=ORIENTED_EDGE('',*,*,#60087,.T.);
#90198=ORIENTED_EDGE('',*,*,#60090,.T.);
#90199=ORIENTED_EDGE('',*,*,#60093,.T.);
#90200=ORIENTED_EDGE('',*,*,#60096,.T.);
#90201=ORIENTED_EDGE('',*,*,#60099,.T.);
#90202=ORIENTED_EDGE('',*,*,#60102,.T.);
#90203=ORIENTED_EDGE('',*,*,#60105,.T.);
#90204=ORIENTED_EDGE('',*,*,#60108,.T.);
#90205=ORIENTED_EDGE('',*,*,#59954,.T.);
#90206=ORIENTED_EDGE('',*,*,#59958,.T.);
#90207=ORIENTED_EDGE('',*,*,#59961,.T.);
#90208=ORIENTED_EDGE('',*,*,#59964,.T.);
#90209=ORIENTED_EDGE('',*,*,#59967,.T.);
#90210=ORIENTED_EDGE('',*,*,#59970,.T.);
#90211=ORIENTED_EDGE('',*,*,#59973,.T.);
#90212=ORIENTED_EDGE('',*,*,#59976,.T.);
#90213=ORIENTED_EDGE('',*,*,#59979,.T.);
#90214=ORIENTED_EDGE('',*,*,#59982,.T.);
#90215=ORIENTED_EDGE('',*,*,#59985,.T.);
#90216=ORIENTED_EDGE('',*,*,#59988,.T.);
#90217=ORIENTED_EDGE('',*,*,#59991,.T.);
#90218=ORIENTED_EDGE('',*,*,#59994,.T.);
#90219=ORIENTED_EDGE('',*,*,#59997,.T.);
#90220=ORIENTED_EDGE('',*,*,#60000,.T.);
#90221=ORIENTED_EDGE('',*,*,#60003,.T.);
#90222=ORIENTED_EDGE('',*,*,#60006,.T.);
#90223=ORIENTED_EDGE('',*,*,#60009,.T.);
#90224=ORIENTED_EDGE('',*,*,#60012,.T.);
#90225=ORIENTED_EDGE('',*,*,#60015,.T.);
#90226=ORIENTED_EDGE('',*,*,#60018,.T.);
#90227=ORIENTED_EDGE('',*,*,#60021,.T.);
#90228=ORIENTED_EDGE('',*,*,#60024,.T.);
#90229=ORIENTED_EDGE('',*,*,#60027,.T.);
#90230=ORIENTED_EDGE('',*,*,#60030,.T.);
#90231=ORIENTED_EDGE('',*,*,#60033,.T.);
#90232=ORIENTED_EDGE('',*,*,#60036,.T.);
#90233=ORIENTED_EDGE('',*,*,#60039,.T.);
#90234=ORIENTED_EDGE('',*,*,#60042,.T.);
#90235=ORIENTED_EDGE('',*,*,#60045,.T.);
#90236=ORIENTED_EDGE('',*,*,#60048,.T.);
#90237=ORIENTED_EDGE('',*,*,#60051,.T.);
#90238=ORIENTED_EDGE('',*,*,#60054,.T.);
#90239=ORIENTED_EDGE('',*,*,#60057,.T.);
#90240=ORIENTED_EDGE('',*,*,#60060,.T.);
#90241=ORIENTED_EDGE('',*,*,#60063,.T.);
#90242=ORIENTED_EDGE('',*,*,#60066,.T.);
#90243=ORIENTED_EDGE('',*,*,#60069,.T.);
#90244=ORIENTED_EDGE('',*,*,#59915,.T.);
#90245=ORIENTED_EDGE('',*,*,#59919,.T.);
#90246=ORIENTED_EDGE('',*,*,#59922,.T.);
#90247=ORIENTED_EDGE('',*,*,#59925,.T.);
#90248=ORIENTED_EDGE('',*,*,#59928,.T.);
#90249=ORIENTED_EDGE('',*,*,#59931,.T.);
#90250=ORIENTED_EDGE('',*,*,#59934,.T.);
#90251=ORIENTED_EDGE('',*,*,#59937,.T.);
#90252=ORIENTED_EDGE('',*,*,#59940,.T.);
#90253=ORIENTED_EDGE('',*,*,#59943,.T.);
#90254=ORIENTED_EDGE('',*,*,#59946,.T.);
#90255=ORIENTED_EDGE('',*,*,#59949,.T.);
#90256=ORIENTED_EDGE('',*,*,#59952,.T.);
#90257=ORIENTED_EDGE('',*,*,#59798,.T.);
#90258=ORIENTED_EDGE('',*,*,#59802,.T.);
#90259=ORIENTED_EDGE('',*,*,#59805,.T.);
#90260=ORIENTED_EDGE('',*,*,#59808,.T.);
#90261=ORIENTED_EDGE('',*,*,#59811,.T.);
#90262=ORIENTED_EDGE('',*,*,#59814,.T.);
#90263=ORIENTED_EDGE('',*,*,#59817,.T.);
#90264=ORIENTED_EDGE('',*,*,#59820,.T.);
#90265=ORIENTED_EDGE('',*,*,#59823,.T.);
#90266=ORIENTED_EDGE('',*,*,#59826,.T.);
#90267=ORIENTED_EDGE('',*,*,#59829,.T.);
#90268=ORIENTED_EDGE('',*,*,#59832,.T.);
#90269=ORIENTED_EDGE('',*,*,#59835,.T.);
#90270=ORIENTED_EDGE('',*,*,#59838,.T.);
#90271=ORIENTED_EDGE('',*,*,#59841,.T.);
#90272=ORIENTED_EDGE('',*,*,#59844,.T.);
#90273=ORIENTED_EDGE('',*,*,#59847,.T.);
#90274=ORIENTED_EDGE('',*,*,#59850,.T.);
#90275=ORIENTED_EDGE('',*,*,#59853,.T.);
#90276=ORIENTED_EDGE('',*,*,#59856,.T.);
#90277=ORIENTED_EDGE('',*,*,#59747,.T.);
#90278=ORIENTED_EDGE('',*,*,#60384,.T.);
#90279=ORIENTED_EDGE('',*,*,#60387,.T.);
#90280=ORIENTED_EDGE('',*,*,#59858,.T.);
#90281=ORIENTED_EDGE('',*,*,#59862,.T.);
#90282=ORIENTED_EDGE('',*,*,#59865,.T.);
#90283=ORIENTED_EDGE('',*,*,#59868,.T.);
#90284=ORIENTED_EDGE('',*,*,#59871,.T.);
#90285=ORIENTED_EDGE('',*,*,#59874,.T.);
#90286=ORIENTED_EDGE('',*,*,#59877,.T.);
#90287=ORIENTED_EDGE('',*,*,#59880,.T.);
#90288=ORIENTED_EDGE('',*,*,#59883,.T.);
#90289=ORIENTED_EDGE('',*,*,#60423,.T.);
#90290=ORIENTED_EDGE('',*,*,#60413,.T.);
#90291=ORIENTED_EDGE('',*,*,#60417,.T.);
#90292=ORIENTED_EDGE('',*,*,#60420,.T.);
#92447=CYLINDRICAL_SURFACE('',#110987,6.3);
#92448=CYLINDRICAL_SURFACE('',#111000,9.92159999999999);
#92449=CYLINDRICAL_SURFACE('',#111003,6.3);
#92450=CYLINDRICAL_SURFACE('',#111006,9.92159999999999);
#92451=CYLINDRICAL_SURFACE('',#111009,6.29999999999999);
#92452=CYLINDRICAL_SURFACE('',#111012,9.92159999999999);
#92453=CYLINDRICAL_SURFACE('',#111015,6.29999999999999);
#92454=CYLINDRICAL_SURFACE('',#111018,9.9216);
#92455=CYLINDRICAL_SURFACE('',#111027,1.8);
#92456=CYLINDRICAL_SURFACE('',#111030,1.8);
#92457=CYLINDRICAL_SURFACE('',#111033,1.8);
#92458=CYLINDRICAL_SURFACE('',#111036,1.8);
#92459=CYLINDRICAL_SURFACE('',#111089,2.7);
#92460=CYLINDRICAL_SURFACE('',#111091,2.69999999999999);
#92461=CYLINDRICAL_SURFACE('',#111093,2.69999999999999);
#92462=CYLINDRICAL_SURFACE('',#111097,2.7);
#92463=CYLINDRICAL_SURFACE('',#111099,2.7);
#92464=CYLINDRICAL_SURFACE('',#111101,2.7);
#92465=CYLINDRICAL_SURFACE('',#111103,2.7);
#92466=CYLINDRICAL_SURFACE('',#111105,2.69999999999999);
#92467=CYLINDRICAL_SURFACE('',#111107,2.69999999999999);
#92468=CYLINDRICAL_SURFACE('',#111111,2.7);
#92469=CYLINDRICAL_SURFACE('',#111113,2.7);
#92470=CYLINDRICAL_SURFACE('',#111115,2.7);
#92471=CYLINDRICAL_SURFACE('',#111117,2.7);
#92472=CYLINDRICAL_SURFACE('',#111119,2.7);
#92473=CYLINDRICAL_SURFACE('',#111121,2.69999999999999);
#92474=CYLINDRICAL_SURFACE('',#111125,2.69999999999999);
#92475=CYLINDRICAL_SURFACE('',#111127,2.7);
#92476=CYLINDRICAL_SURFACE('',#111129,2.7);
#92477=CYLINDRICAL_SURFACE('',#111131,2.7);
#92478=CYLINDRICAL_SURFACE('',#111133,2.69999999999999);
#92479=CYLINDRICAL_SURFACE('',#111135,2.7);
#92480=CYLINDRICAL_SURFACE('',#111139,2.69999999999999);
#92481=CYLINDRICAL_SURFACE('',#111141,2.7);
#92482=CYLINDRICAL_SURFACE('',#111143,2.7);
#92483=CYLINDRICAL_SURFACE('',#111145,6.29999999999999);
#92484=CYLINDRICAL_SURFACE('',#111157,6.3);
#92485=CYLINDRICAL_SURFACE('',#111160,9.92159999999999);
#92486=CYLINDRICAL_SURFACE('',#111163,6.3);
#92487=CYLINDRICAL_SURFACE('',#111166,9.92159999999999);
#92488=CYLINDRICAL_SURFACE('',#111170,9.92159999999999);
#92489=CYLINDRICAL_SURFACE('',#111173,6.29999999999999);
#92490=CYLINDRICAL_SURFACE('',#111176,9.9216);
#92491=CYLINDRICAL_SURFACE('',#111185,1.8);
#92492=CYLINDRICAL_SURFACE('',#111188,1.8);
#92493=CYLINDRICAL_SURFACE('',#111191,1.8);
#92494=CYLINDRICAL_SURFACE('',#111194,1.8);
#92495=CYLINDRICAL_SURFACE('',#111197,6.29999999999999);
#92496=CYLINDRICAL_SURFACE('',#111209,6.3);
#92497=CYLINDRICAL_SURFACE('',#111212,9.92159999999999);
#92498=CYLINDRICAL_SURFACE('',#111215,6.3);
#92499=CYLINDRICAL_SURFACE('',#111218,9.92159999999999);
#92500=CYLINDRICAL_SURFACE('',#111221,6.29999999999999);
#92501=CYLINDRICAL_SURFACE('',#111224,9.92159999999999);
#92502=CYLINDRICAL_SURFACE('',#111228,9.9216);
#92503=CYLINDRICAL_SURFACE('',#111237,1.8);
#92504=CYLINDRICAL_SURFACE('',#111240,1.8);
#92505=CYLINDRICAL_SURFACE('',#111243,1.8);
#92506=CYLINDRICAL_SURFACE('',#111246,1.8);
#92507=CYLINDRICAL_SURFACE('',#111249,6.29999999999999);
#92508=CYLINDRICAL_SURFACE('',#111261,6.3);
#92509=CYLINDRICAL_SURFACE('',#111264,9.92159999999999);
#92510=CYLINDRICAL_SURFACE('',#111267,6.3);
#92511=CYLINDRICAL_SURFACE('',#111270,9.92159999999999);
#92512=CYLINDRICAL_SURFACE('',#111273,6.29999999999999);
#92513=CYLINDRICAL_SURFACE('',#111276,9.92159999999999);
#92514=CYLINDRICAL_SURFACE('',#111280,9.9216);
#92515=CYLINDRICAL_SURFACE('',#111289,1.8);
#92516=CYLINDRICAL_SURFACE('',#111292,1.8);
#92517=CYLINDRICAL_SURFACE('',#111295,1.8);
#92518=CYLINDRICAL_SURFACE('',#111298,1.8);
#92519=CYLINDRICAL_SURFACE('',#111306,0.899999999999998);
#92520=CYLINDRICAL_SURFACE('',#111310,0.899999999999998);
#92521=CYLINDRICAL_SURFACE('',#111314,0.899999999999998);
#92522=CYLINDRICAL_SURFACE('',#111318,0.899999999999991);
#92523=CYLINDRICAL_SURFACE('',#111329,0.899999999999995);
#92524=CYLINDRICAL_SURFACE('',#111333,0.900000000000001);
#92525=CYLINDRICAL_SURFACE('',#111337,0.899999999999996);
#92526=CYLINDRICAL_SURFACE('',#111341,0.899999999999998);
#92527=CYLINDRICAL_SURFACE('',#111348,0.899999999999998);
#92528=CYLINDRICAL_SURFACE('',#111352,0.899999999999998);
#92529=CYLINDRICAL_SURFACE('',#111356,0.899999999999991);
#92530=CYLINDRICAL_SURFACE('',#111360,0.899999999999998);
#92531=CYLINDRICAL_SURFACE('',#111367,3.65760000000007);
#92532=CYLINDRICAL_SURFACE('',#111374,0.899999999999991);
#92533=CYLINDRICAL_SURFACE('',#111378,0.899999999999998);
#92534=CYLINDRICAL_SURFACE('',#111382,0.899999999999998);
#92535=CYLINDRICAL_SURFACE('',#111386,0.899999999999998);
#92536=CYLINDRICAL_SURFACE('',#111393,0.899999999999998);
#92537=CYLINDRICAL_SURFACE('',#111397,0.899999999999998);
#92538=CYLINDRICAL_SURFACE('',#111401,0.899999999999998);
#92539=CYLINDRICAL_SURFACE('',#111405,0.899999999999991);
#92540=CYLINDRICAL_SURFACE('',#111415,0.899999999999995);
#92541=CYLINDRICAL_SURFACE('',#111419,0.900000000000001);
#92542=CYLINDRICAL_SURFACE('',#111423,0.899999999999996);
#92543=CYLINDRICAL_SURFACE('',#111427,0.899999999999998);
#92544=CYLINDRICAL_SURFACE('',#111434,0.899999999999998);
#92545=CYLINDRICAL_SURFACE('',#111438,0.899999999999998);
#92546=CYLINDRICAL_SURFACE('',#111442,0.899999999999991);
#92547=CYLINDRICAL_SURFACE('',#111446,0.899999999999998);
#92548=CYLINDRICAL_SURFACE('',#111453,3.65760000000007);
#92549=CYLINDRICAL_SURFACE('',#111460,0.899999999999991);
#92550=CYLINDRICAL_SURFACE('',#111464,0.899999999999998);
#92551=CYLINDRICAL_SURFACE('',#111468,0.899999999999998);
#92552=CYLINDRICAL_SURFACE('',#111472,0.899999999999998);
#92553=CYLINDRICAL_SURFACE('',#111479,0.899999999999998);
#92554=CYLINDRICAL_SURFACE('',#111483,0.899999999999996);
#92555=CYLINDRICAL_SURFACE('',#111487,0.900000000000001);
#92556=CYLINDRICAL_SURFACE('',#111491,0.899999999999995);
#92557=CYLINDRICAL_SURFACE('',#111501,0.899999999999991);
#92558=CYLINDRICAL_SURFACE('',#111505,0.899999999999998);
#92559=CYLINDRICAL_SURFACE('',#111509,0.899999999999998);
#92560=CYLINDRICAL_SURFACE('',#111513,0.899999999999998);
#92561=CYLINDRICAL_SURFACE('',#111520,0.899999999999998);
#92562=CYLINDRICAL_SURFACE('',#111524,0.899999999999998);
#92563=CYLINDRICAL_SURFACE('',#111528,0.899999999999991);
#92564=CYLINDRICAL_SURFACE('',#111532,0.899999999999998);
#92565=CYLINDRICAL_SURFACE('',#111539,3.65760000000007);
#92566=CYLINDRICAL_SURFACE('',#111546,0.899999999999991);
#92567=CYLINDRICAL_SURFACE('',#111550,0.899999999999998);
#92568=CYLINDRICAL_SURFACE('',#111554,0.899999999999998);
#92569=CYLINDRICAL_SURFACE('',#111558,0.899999999999998);
#92570=CYLINDRICAL_SURFACE('',#111565,0.899999999999998);
#92571=CYLINDRICAL_SURFACE('',#111569,0.899999999999996);
#92572=CYLINDRICAL_SURFACE('',#111573,0.900000000000001);
#92573=CYLINDRICAL_SURFACE('',#111577,0.899999999999995);
#92574=CYLINDRICAL_SURFACE('',#111586,0.899999999999991);
#92575=CYLINDRICAL_SURFACE('',#111590,0.899999999999998);
#92576=CYLINDRICAL_SURFACE('',#111594,0.899999999999998);
#92577=CYLINDRICAL_SURFACE('',#111598,0.899999999999998);
#92578=CYLINDRICAL_SURFACE('',#111605,0.899999999999998);
#92579=CYLINDRICAL_SURFACE('',#111609,0.899999999999998);
#92580=CYLINDRICAL_SURFACE('',#111613,0.899999999999991);
#92581=CYLINDRICAL_SURFACE('',#111617,0.899999999999998);
#92582=CYLINDRICAL_SURFACE('',#111624,3.65760000000007);
#92583=CYLINDRICAL_SURFACE('',#111631,0.899999999999991);
#92584=CYLINDRICAL_SURFACE('',#111635,0.899999999999998);
#92585=CYLINDRICAL_SURFACE('',#111639,0.899999999999998);
#92586=CYLINDRICAL_SURFACE('',#111643,0.899999999999998);
#98297=ADVANCED_FACE('',(#13324),#92447,.F.);
#98298=ADVANCED_FACE('',(#13325),#7354,.F.);
#98299=ADVANCED_FACE('',(#13326),#7355,.T.);
#98300=ADVANCED_FACE('',(#13327),#7356,.T.);
#98301=ADVANCED_FACE('',(#13328),#92448,.F.);
#98302=ADVANCED_FACE('',(#13329),#7357,.T.);
#98303=ADVANCED_FACE('',(#13330),#92449,.F.);
#98304=ADVANCED_FACE('',(#13331),#7358,.T.);
#98305=ADVANCED_FACE('',(#13332),#92450,.F.);
#98306=ADVANCED_FACE('',(#13333),#7359,.T.);
#98307=ADVANCED_FACE('',(#13334),#92451,.F.);
#98308=ADVANCED_FACE('',(#13335),#7360,.T.);
#98309=ADVANCED_FACE('',(#13336),#92452,.F.);
#98310=ADVANCED_FACE('',(#13337),#7361,.T.);
#98311=ADVANCED_FACE('',(#13338),#92453,.F.);
#98312=ADVANCED_FACE('',(#13339),#7362,.T.);
#98313=ADVANCED_FACE('',(#13340),#92454,.F.);
#98314=ADVANCED_FACE('',(#13341),#7363,.F.);
#98315=ADVANCED_FACE('',(#13342),#7364,.F.);
#98316=ADVANCED_FACE('',(#13343),#7365,.T.);
#98317=ADVANCED_FACE('',(#13344),#92455,.F.);
#98318=ADVANCED_FACE('',(#13345),#7366,.T.);
#98319=ADVANCED_FACE('',(#13346),#92456,.F.);
#98320=ADVANCED_FACE('',(#13347),#7367,.T.);
#98321=ADVANCED_FACE('',(#13348),#92457,.F.);
#98322=ADVANCED_FACE('',(#13349),#7368,.T.);
#98323=ADVANCED_FACE('',(#13350),#92458,.F.);
#98324=ADVANCED_FACE('',(#13351),#7369,.F.);
#98325=ADVANCED_FACE('',(#13352),#7370,.F.);
#98326=ADVANCED_FACE('',(#13353),#7371,.F.);
#98327=ADVANCED_FACE('',(#13354),#92459,.F.);
#98328=ADVANCED_FACE('',(#13355),#7372,.F.);
#98329=ADVANCED_FACE('',(#13356),#92460,.T.);
#98330=ADVANCED_FACE('',(#13357),#7373,.F.);
#98331=ADVANCED_FACE('',(#13358),#92461,.F.);
#98332=ADVANCED_FACE('',(#13359),#7374,.F.);
#98333=ADVANCED_FACE('',(#13360),#7375,.F.);
#98334=ADVANCED_FACE('',(#13361),#7376,.F.);
#98335=ADVANCED_FACE('',(#13362),#92462,.F.);
#98336=ADVANCED_FACE('',(#13363),#7377,.F.);
#98337=ADVANCED_FACE('',(#13364),#92463,.T.);
#98338=ADVANCED_FACE('',(#13365),#7378,.F.);
#98339=ADVANCED_FACE('',(#13366),#92464,.F.);
#98340=ADVANCED_FACE('',(#13367),#7379,.F.);
#98341=ADVANCED_FACE('',(#13368),#92465,.F.);
#98342=ADVANCED_FACE('',(#13369),#7380,.F.);
#98343=ADVANCED_FACE('',(#13370),#92466,.T.);
#98344=ADVANCED_FACE('',(#13371),#7381,.F.);
#98345=ADVANCED_FACE('',(#13372),#92467,.F.);
#98346=ADVANCED_FACE('',(#13373),#7382,.F.);
#98347=ADVANCED_FACE('',(#13374),#7383,.F.);
#98348=ADVANCED_FACE('',(#13375),#7384,.F.);
#98349=ADVANCED_FACE('',(#13376),#92468,.F.);
#98350=ADVANCED_FACE('',(#13377),#7385,.F.);
#98351=ADVANCED_FACE('',(#13378),#92469,.T.);
#98352=ADVANCED_FACE('',(#13379),#7386,.F.);
#98353=ADVANCED_FACE('',(#13380),#92470,.F.);
#98354=ADVANCED_FACE('',(#13381),#7387,.F.);
#98355=ADVANCED_FACE('',(#13382),#92471,.F.);
#98356=ADVANCED_FACE('',(#13383),#7388,.F.);
#98357=ADVANCED_FACE('',(#13384),#92472,.T.);
#98358=ADVANCED_FACE('',(#13385),#7389,.F.);
#98359=ADVANCED_FACE('',(#13386),#92473,.F.);
#98360=ADVANCED_FACE('',(#13387),#7390,.F.);
#98361=ADVANCED_FACE('',(#13388),#7391,.F.);
#98362=ADVANCED_FACE('',(#13389),#7392,.F.);
#98363=ADVANCED_FACE('',(#13390),#92474,.F.);
#98364=ADVANCED_FACE('',(#13391),#7393,.F.);
#98365=ADVANCED_FACE('',(#13392),#92475,.T.);
#98366=ADVANCED_FACE('',(#13393),#7394,.F.);
#98367=ADVANCED_FACE('',(#13394),#92476,.F.);
#98368=ADVANCED_FACE('',(#13395),#7395,.F.);
#98369=ADVANCED_FACE('',(#13396),#92477,.F.);
#98370=ADVANCED_FACE('',(#13397),#7396,.F.);
#98371=ADVANCED_FACE('',(#13398),#92478,.T.);
#98372=ADVANCED_FACE('',(#13399),#7397,.F.);
#98373=ADVANCED_FACE('',(#13400),#92479,.F.);
#98374=ADVANCED_FACE('',(#13401),#7398,.F.);
#98375=ADVANCED_FACE('',(#13402),#7399,.F.);
#98376=ADVANCED_FACE('',(#13403),#7400,.F.);
#98377=ADVANCED_FACE('',(#13404),#92480,.F.);
#98378=ADVANCED_FACE('',(#13405),#7401,.F.);
#98379=ADVANCED_FACE('',(#13406),#92481,.T.);
#98380=ADVANCED_FACE('',(#13407),#7402,.F.);
#98381=ADVANCED_FACE('',(#13408),#92482,.F.);
#98382=ADVANCED_FACE('',(#13409),#7403,.F.);
#98383=ADVANCED_FACE('',(#13410),#92483,.F.);
#98384=ADVANCED_FACE('',(#13411),#7404,.F.);
#98385=ADVANCED_FACE('',(#13412),#7405,.T.);
#98386=ADVANCED_FACE('',(#13413),#92484,.F.);
#98387=ADVANCED_FACE('',(#13414),#7406,.T.);
#98388=ADVANCED_FACE('',(#13415),#92485,.F.);
#98389=ADVANCED_FACE('',(#13416),#7407,.T.);
#98390=ADVANCED_FACE('',(#13417),#92486,.F.);
#98391=ADVANCED_FACE('',(#13418),#7408,.T.);
#98392=ADVANCED_FACE('',(#13419),#92487,.F.);
#98393=ADVANCED_FACE('',(#13420),#7409,.T.);
#98394=ADVANCED_FACE('',(#13421),#7410,.T.);
#98395=ADVANCED_FACE('',(#13422),#92488,.F.);
#98396=ADVANCED_FACE('',(#13423),#7411,.T.);
#98397=ADVANCED_FACE('',(#13424),#92489,.F.);
#98398=ADVANCED_FACE('',(#13425),#7412,.T.);
#98399=ADVANCED_FACE('',(#13426),#92490,.F.);
#98400=ADVANCED_FACE('',(#13427),#7413,.F.);
#98401=ADVANCED_FACE('',(#13428),#7414,.F.);
#98402=ADVANCED_FACE('',(#13429),#7415,.T.);
#98403=ADVANCED_FACE('',(#13430),#92491,.F.);
#98404=ADVANCED_FACE('',(#13431),#7416,.T.);
#98405=ADVANCED_FACE('',(#13432),#92492,.F.);
#98406=ADVANCED_FACE('',(#13433),#7417,.T.);
#98407=ADVANCED_FACE('',(#13434),#92493,.F.);
#98408=ADVANCED_FACE('',(#13435),#7418,.T.);
#98409=ADVANCED_FACE('',(#13436),#92494,.F.);
#98410=ADVANCED_FACE('',(#13437),#7419,.F.);
#98411=ADVANCED_FACE('',(#13438),#92495,.F.);
#98412=ADVANCED_FACE('',(#13439),#7420,.F.);
#98413=ADVANCED_FACE('',(#13440),#7421,.T.);
#98414=ADVANCED_FACE('',(#13441),#92496,.F.);
#98415=ADVANCED_FACE('',(#13442),#7422,.T.);
#98416=ADVANCED_FACE('',(#13443),#92497,.F.);
#98417=ADVANCED_FACE('',(#13444),#7423,.T.);
#98418=ADVANCED_FACE('',(#13445),#92498,.F.);
#98419=ADVANCED_FACE('',(#13446),#7424,.T.);
#98420=ADVANCED_FACE('',(#13447),#92499,.F.);
#98421=ADVANCED_FACE('',(#13448),#7425,.T.);
#98422=ADVANCED_FACE('',(#13449),#92500,.F.);
#98423=ADVANCED_FACE('',(#13450),#7426,.T.);
#98424=ADVANCED_FACE('',(#13451),#92501,.F.);
#98425=ADVANCED_FACE('',(#13452),#7427,.T.);
#98426=ADVANCED_FACE('',(#13453),#7428,.T.);
#98427=ADVANCED_FACE('',(#13454),#92502,.F.);
#98428=ADVANCED_FACE('',(#13455),#7429,.F.);
#98429=ADVANCED_FACE('',(#13456),#7430,.F.);
#98430=ADVANCED_FACE('',(#13457),#7431,.T.);
#98431=ADVANCED_FACE('',(#13458),#92503,.F.);
#98432=ADVANCED_FACE('',(#13459),#7432,.T.);
#98433=ADVANCED_FACE('',(#13460),#92504,.F.);
#98434=ADVANCED_FACE('',(#13461),#7433,.T.);
#98435=ADVANCED_FACE('',(#13462),#92505,.F.);
#98436=ADVANCED_FACE('',(#13463),#7434,.T.);
#98437=ADVANCED_FACE('',(#13464),#92506,.F.);
#98438=ADVANCED_FACE('',(#13465),#7435,.F.);
#98439=ADVANCED_FACE('',(#13466),#92507,.F.);
#98440=ADVANCED_FACE('',(#13467),#7436,.F.);
#98441=ADVANCED_FACE('',(#13468),#7437,.T.);
#98442=ADVANCED_FACE('',(#13469),#92508,.F.);
#98443=ADVANCED_FACE('',(#13470),#7438,.T.);
#98444=ADVANCED_FACE('',(#13471),#92509,.F.);
#98445=ADVANCED_FACE('',(#13472),#7439,.T.);
#98446=ADVANCED_FACE('',(#13473),#92510,.F.);
#98447=ADVANCED_FACE('',(#13474),#7440,.T.);
#98448=ADVANCED_FACE('',(#13475),#92511,.F.);
#98449=ADVANCED_FACE('',(#13476),#7441,.T.);
#98450=ADVANCED_FACE('',(#13477),#92512,.F.);
#98451=ADVANCED_FACE('',(#13478),#7442,.T.);
#98452=ADVANCED_FACE('',(#13479),#92513,.F.);
#98453=ADVANCED_FACE('',(#13480),#7443,.T.);
#98454=ADVANCED_FACE('',(#13481),#7444,.T.);
#98455=ADVANCED_FACE('',(#13482),#92514,.F.);
#98456=ADVANCED_FACE('',(#13483),#7445,.F.);
#98457=ADVANCED_FACE('',(#13484),#7446,.F.);
#98458=ADVANCED_FACE('',(#13485),#7447,.T.);
#98459=ADVANCED_FACE('',(#13486),#92515,.F.);
#98460=ADVANCED_FACE('',(#13487),#7448,.T.);
#98461=ADVANCED_FACE('',(#13488),#92516,.F.);
#98462=ADVANCED_FACE('',(#13489),#7449,.T.);
#98463=ADVANCED_FACE('',(#13490),#92517,.F.);
#98464=ADVANCED_FACE('',(#13491),#7450,.T.);
#98465=ADVANCED_FACE('',(#13492),#92518,.F.);
#98466=ADVANCED_FACE('',(#13493),#7451,.F.);
#98467=ADVANCED_FACE('',(#13494),#7452,.F.);
#98468=ADVANCED_FACE('',(#13495),#7453,.F.);
#98469=ADVANCED_FACE('',(#13496),#7454,.F.);
#98470=ADVANCED_FACE('',(#13497),#7455,.F.);
#98471=ADVANCED_FACE('',(#13498),#7456,.F.);
#98472=ADVANCED_FACE('',(#13499),#92519,.F.);
#98473=ADVANCED_FACE('',(#13500),#7457,.F.);
#98474=ADVANCED_FACE('',(#13501),#92520,.F.);
#98475=ADVANCED_FACE('',(#13502),#7458,.F.);
#98476=ADVANCED_FACE('',(#13503),#92521,.F.);
#98477=ADVANCED_FACE('',(#13504),#7459,.F.);
#98478=ADVANCED_FACE('',(#13505),#92522,.T.);
#98479=ADVANCED_FACE('',(#13506),#7460,.F.);
#98480=ADVANCED_FACE('',(#13507),#7461,.F.);
#98481=ADVANCED_FACE('',(#13508),#7462,.F.);
#98482=ADVANCED_FACE('',(#13509),#7463,.F.);
#98483=ADVANCED_FACE('',(#13510),#7464,.F.);
#98484=ADVANCED_FACE('',(#13511),#7465,.F.);
#98485=ADVANCED_FACE('',(#13512),#7466,.F.);
#98486=ADVANCED_FACE('',(#13513),#7467,.F.);
#98487=ADVANCED_FACE('',(#13514),#92523,.T.);
#98488=ADVANCED_FACE('',(#13515),#7468,.F.);
#98489=ADVANCED_FACE('',(#13516),#92524,.F.);
#98490=ADVANCED_FACE('',(#13517),#7469,.F.);
#98491=ADVANCED_FACE('',(#13518),#92525,.F.);
#98492=ADVANCED_FACE('',(#13519),#7470,.F.);
#98493=ADVANCED_FACE('',(#13520),#92526,.F.);
#98494=ADVANCED_FACE('',(#13521),#7471,.F.);
#98495=ADVANCED_FACE('',(#13522),#7472,.F.);
#98496=ADVANCED_FACE('',(#13523),#7473,.F.);
#98497=ADVANCED_FACE('',(#13524),#7474,.F.);
#98498=ADVANCED_FACE('',(#13525),#92527,.F.);
#98499=ADVANCED_FACE('',(#13526),#7475,.F.);
#98500=ADVANCED_FACE('',(#13527),#92528,.F.);
#98501=ADVANCED_FACE('',(#13528),#7476,.F.);
#98502=ADVANCED_FACE('',(#13529),#92529,.F.);
#98503=ADVANCED_FACE('',(#13530),#7477,.F.);
#98504=ADVANCED_FACE('',(#13531),#92530,.T.);
#98505=ADVANCED_FACE('',(#13532),#7478,.F.);
#98506=ADVANCED_FACE('',(#13533),#7479,.F.);
#98507=ADVANCED_FACE('',(#13534),#7480,.F.);
#98508=ADVANCED_FACE('',(#13535),#7481,.F.);
#98509=ADVANCED_FACE('',(#13536),#92531,.T.);
#98510=ADVANCED_FACE('',(#13537),#7482,.F.);
#98511=ADVANCED_FACE('',(#13538),#7483,.F.);
#98512=ADVANCED_FACE('',(#13539),#7484,.F.);
#98513=ADVANCED_FACE('',(#13540),#7485,.F.);
#98514=ADVANCED_FACE('',(#13541),#92532,.T.);
#98515=ADVANCED_FACE('',(#13542),#7486,.F.);
#98516=ADVANCED_FACE('',(#13543),#92533,.F.);
#98517=ADVANCED_FACE('',(#13544),#7487,.F.);
#98518=ADVANCED_FACE('',(#13545),#92534,.F.);
#98519=ADVANCED_FACE('',(#13546),#7488,.F.);
#98520=ADVANCED_FACE('',(#13547),#92535,.F.);
#98521=ADVANCED_FACE('',(#13548),#7489,.F.);
#98522=ADVANCED_FACE('',(#13549),#7490,.F.);
#98523=ADVANCED_FACE('',(#13550),#7491,.F.);
#98524=ADVANCED_FACE('',(#13551),#7492,.F.);
#98525=ADVANCED_FACE('',(#13552),#92536,.F.);
#98526=ADVANCED_FACE('',(#13553),#7493,.F.);
#98527=ADVANCED_FACE('',(#13554),#92537,.F.);
#98528=ADVANCED_FACE('',(#13555),#7494,.F.);
#98529=ADVANCED_FACE('',(#13556),#92538,.F.);
#98530=ADVANCED_FACE('',(#13557),#7495,.F.);
#98531=ADVANCED_FACE('',(#13558),#92539,.T.);
#98532=ADVANCED_FACE('',(#13559),#7496,.F.);
#98533=ADVANCED_FACE('',(#13560),#7497,.F.);
#98534=ADVANCED_FACE('',(#13561),#7498,.F.);
#98535=ADVANCED_FACE('',(#13562),#7499,.F.);
#98536=ADVANCED_FACE('',(#13563),#7500,.F.);
#98537=ADVANCED_FACE('',(#13564),#7501,.F.);
#98538=ADVANCED_FACE('',(#13565),#7502,.F.);
#98539=ADVANCED_FACE('',(#13566),#92540,.T.);
#98540=ADVANCED_FACE('',(#13567),#7503,.F.);
#98541=ADVANCED_FACE('',(#13568),#92541,.F.);
#98542=ADVANCED_FACE('',(#13569),#7504,.F.);
#98543=ADVANCED_FACE('',(#13570),#92542,.F.);
#98544=ADVANCED_FACE('',(#13571),#7505,.F.);
#98545=ADVANCED_FACE('',(#13572),#92543,.F.);
#98546=ADVANCED_FACE('',(#13573),#7506,.F.);
#98547=ADVANCED_FACE('',(#13574),#7507,.F.);
#98548=ADVANCED_FACE('',(#13575),#7508,.F.);
#98549=ADVANCED_FACE('',(#13576),#7509,.F.);
#98550=ADVANCED_FACE('',(#13577),#92544,.F.);
#98551=ADVANCED_FACE('',(#13578),#7510,.F.);
#98552=ADVANCED_FACE('',(#13579),#92545,.F.);
#98553=ADVANCED_FACE('',(#13580),#7511,.F.);
#98554=ADVANCED_FACE('',(#13581),#92546,.F.);
#98555=ADVANCED_FACE('',(#13582),#7512,.F.);
#98556=ADVANCED_FACE('',(#13583),#92547,.T.);
#98557=ADVANCED_FACE('',(#13584),#7513,.F.);
#98558=ADVANCED_FACE('',(#13585),#7514,.F.);
#98559=ADVANCED_FACE('',(#13586),#7515,.F.);
#98560=ADVANCED_FACE('',(#13587),#7516,.F.);
#98561=ADVANCED_FACE('',(#13588),#92548,.T.);
#98562=ADVANCED_FACE('',(#13589),#7517,.F.);
#98563=ADVANCED_FACE('',(#13590),#7518,.F.);
#98564=ADVANCED_FACE('',(#13591),#7519,.F.);
#98565=ADVANCED_FACE('',(#13592),#7520,.F.);
#98566=ADVANCED_FACE('',(#13593),#92549,.T.);
#98567=ADVANCED_FACE('',(#13594),#7521,.F.);
#98568=ADVANCED_FACE('',(#13595),#92550,.F.);
#98569=ADVANCED_FACE('',(#13596),#7522,.F.);
#98570=ADVANCED_FACE('',(#13597),#92551,.F.);
#98571=ADVANCED_FACE('',(#13598),#7523,.F.);
#98572=ADVANCED_FACE('',(#13599),#92552,.F.);
#98573=ADVANCED_FACE('',(#13600),#7524,.F.);
#98574=ADVANCED_FACE('',(#13601),#7525,.F.);
#98575=ADVANCED_FACE('',(#13602),#7526,.F.);
#98576=ADVANCED_FACE('',(#13603),#7527,.F.);
#98577=ADVANCED_FACE('',(#13604),#92553,.F.);
#98578=ADVANCED_FACE('',(#13605),#7528,.F.);
#98579=ADVANCED_FACE('',(#13606),#92554,.F.);
#98580=ADVANCED_FACE('',(#13607),#7529,.F.);
#98581=ADVANCED_FACE('',(#13608),#92555,.F.);
#98582=ADVANCED_FACE('',(#13609),#7530,.F.);
#98583=ADVANCED_FACE('',(#13610),#92556,.T.);
#98584=ADVANCED_FACE('',(#13611),#7531,.F.);
#98585=ADVANCED_FACE('',(#13612),#7532,.F.);
#98586=ADVANCED_FACE('',(#13613),#7533,.F.);
#98587=ADVANCED_FACE('',(#13614),#7534,.F.);
#98588=ADVANCED_FACE('',(#13615),#7535,.F.);
#98589=ADVANCED_FACE('',(#13616),#7536,.F.);
#98590=ADVANCED_FACE('',(#13617),#7537,.F.);
#98591=ADVANCED_FACE('',(#13618),#92557,.T.);
#98592=ADVANCED_FACE('',(#13619),#7538,.F.);
#98593=ADVANCED_FACE('',(#13620),#92558,.F.);
#98594=ADVANCED_FACE('',(#13621),#7539,.F.);
#98595=ADVANCED_FACE('',(#13622),#92559,.F.);
#98596=ADVANCED_FACE('',(#13623),#7540,.F.);
#98597=ADVANCED_FACE('',(#13624),#92560,.F.);
#98598=ADVANCED_FACE('',(#13625),#7541,.F.);
#98599=ADVANCED_FACE('',(#13626),#7542,.F.);
#98600=ADVANCED_FACE('',(#13627),#7543,.F.);
#98601=ADVANCED_FACE('',(#13628),#7544,.F.);
#98602=ADVANCED_FACE('',(#13629),#92561,.F.);
#98603=ADVANCED_FACE('',(#13630),#7545,.F.);
#98604=ADVANCED_FACE('',(#13631),#92562,.F.);
#98605=ADVANCED_FACE('',(#13632),#7546,.F.);
#98606=ADVANCED_FACE('',(#13633),#92563,.F.);
#98607=ADVANCED_FACE('',(#13634),#7547,.F.);
#98608=ADVANCED_FACE('',(#13635),#92564,.T.);
#98609=ADVANCED_FACE('',(#13636),#7548,.F.);
#98610=ADVANCED_FACE('',(#13637),#7549,.F.);
#98611=ADVANCED_FACE('',(#13638),#7550,.F.);
#98612=ADVANCED_FACE('',(#13639),#7551,.F.);
#98613=ADVANCED_FACE('',(#13640),#92565,.T.);
#98614=ADVANCED_FACE('',(#13641),#7552,.F.);
#98615=ADVANCED_FACE('',(#13642),#7553,.F.);
#98616=ADVANCED_FACE('',(#13643),#7554,.F.);
#98617=ADVANCED_FACE('',(#13644),#7555,.F.);
#98618=ADVANCED_FACE('',(#13645),#92566,.T.);
#98619=ADVANCED_FACE('',(#13646),#7556,.F.);
#98620=ADVANCED_FACE('',(#13647),#92567,.F.);
#98621=ADVANCED_FACE('',(#13648),#7557,.F.);
#98622=ADVANCED_FACE('',(#13649),#92568,.F.);
#98623=ADVANCED_FACE('',(#13650),#7558,.F.);
#98624=ADVANCED_FACE('',(#13651),#92569,.F.);
#98625=ADVANCED_FACE('',(#13652),#7559,.F.);
#98626=ADVANCED_FACE('',(#13653),#7560,.F.);
#98627=ADVANCED_FACE('',(#13654),#7561,.F.);
#98628=ADVANCED_FACE('',(#13655),#7562,.F.);
#98629=ADVANCED_FACE('',(#13656),#92570,.F.);
#98630=ADVANCED_FACE('',(#13657),#7563,.F.);
#98631=ADVANCED_FACE('',(#13658),#92571,.F.);
#98632=ADVANCED_FACE('',(#13659),#7564,.F.);
#98633=ADVANCED_FACE('',(#13660),#92572,.F.);
#98634=ADVANCED_FACE('',(#13661),#7565,.F.);
#98635=ADVANCED_FACE('',(#13662),#92573,.T.);
#98636=ADVANCED_FACE('',(#13663),#7566,.F.);
#98637=ADVANCED_FACE('',(#13664),#7567,.F.);
#98638=ADVANCED_FACE('',(#13665),#7568,.F.);
#98639=ADVANCED_FACE('',(#13666),#7569,.F.);
#98640=ADVANCED_FACE('',(#13667),#7570,.F.);
#98641=ADVANCED_FACE('',(#13668),#7571,.F.);
#98642=ADVANCED_FACE('',(#13669),#92574,.T.);
#98643=ADVANCED_FACE('',(#13670),#7572,.F.);
#98644=ADVANCED_FACE('',(#13671),#92575,.F.);
#98645=ADVANCED_FACE('',(#13672),#7573,.F.);
#98646=ADVANCED_FACE('',(#13673),#92576,.F.);
#98647=ADVANCED_FACE('',(#13674),#7574,.F.);
#98648=ADVANCED_FACE('',(#13675),#92577,.F.);
#98649=ADVANCED_FACE('',(#13676),#7575,.F.);
#98650=ADVANCED_FACE('',(#13677),#7576,.F.);
#98651=ADVANCED_FACE('',(#13678),#7577,.F.);
#98652=ADVANCED_FACE('',(#13679),#7578,.F.);
#98653=ADVANCED_FACE('',(#13680),#92578,.F.);
#98654=ADVANCED_FACE('',(#13681),#7579,.F.);
#98655=ADVANCED_FACE('',(#13682),#92579,.F.);
#98656=ADVANCED_FACE('',(#13683),#7580,.F.);
#98657=ADVANCED_FACE('',(#13684),#92580,.F.);
#98658=ADVANCED_FACE('',(#13685),#7581,.F.);
#98659=ADVANCED_FACE('',(#13686),#92581,.T.);
#98660=ADVANCED_FACE('',(#13687),#7582,.F.);
#98661=ADVANCED_FACE('',(#13688),#7583,.F.);
#98662=ADVANCED_FACE('',(#13689),#7584,.F.);
#98663=ADVANCED_FACE('',(#13690),#7585,.F.);
#98664=ADVANCED_FACE('',(#13691),#92582,.T.);
#98665=ADVANCED_FACE('',(#13692),#7586,.F.);
#98666=ADVANCED_FACE('',(#13693),#7587,.F.);
#98667=ADVANCED_FACE('',(#13694),#7588,.F.);
#98668=ADVANCED_FACE('',(#13695),#7589,.F.);
#98669=ADVANCED_FACE('',(#13696),#92583,.T.);
#98670=ADVANCED_FACE('',(#13697),#7590,.F.);
#98671=ADVANCED_FACE('',(#13698),#92584,.F.);
#98672=ADVANCED_FACE('',(#13699),#7591,.F.);
#98673=ADVANCED_FACE('',(#13700),#92585,.F.);
#98674=ADVANCED_FACE('',(#13701),#7592,.F.);
#98675=ADVANCED_FACE('',(#13702),#92586,.F.);
#98676=ADVANCED_FACE('',(#13703),#7593,.F.);
#98677=ADVANCED_FACE('',(#13704),#7594,.F.);
#98678=ADVANCED_FACE('',(#13705),#7595,.F.);
#98679=ADVANCED_FACE('',(#13706),#7596,.F.);
#98680=ADVANCED_FACE('',(#13707),#7597,.F.);
#98681=ADVANCED_FACE('',(#13708),#7598,.T.);
#98682=ADVANCED_FACE('',(#13709),#7599,.T.);
#98683=ADVANCED_FACE('',(#13710),#7600,.F.);
#98684=ADVANCED_FACE('',(#13711),#7601,.F.);
#98685=ADVANCED_FACE('',(#13712),#7602,.T.);
#98686=ADVANCED_FACE('',(#13713),#7603,.F.);
#98687=ADVANCED_FACE('',(#13714),#7604,.T.);
#98688=ADVANCED_FACE('',(#13715),#7605,.T.);
#98689=ADVANCED_FACE('',(#13716),#7606,.T.);
#98690=ADVANCED_FACE('',(#13717,#6444),#7607,.F.);
#98691=ADVANCED_FACE('',(#13718),#7608,.T.);
#98692=ADVANCED_FACE('',(#13719),#7609,.T.);
#98693=ADVANCED_FACE('',(#13720),#7610,.T.);
#98694=ADVANCED_FACE('',(#13721),#7611,.T.);
#98695=ADVANCED_FACE('',(#13722,#6445),#7612,.F.);
#98696=ADVANCED_FACE('',(#13723),#7613,.F.);
#98725=CLOSED_SHELL('',(#98297,#98298,#98299,#98300,#98301,#98302,#98303,
#98304,#98305,#98306,#98307,#98308,#98309,#98310,#98311,#98312,#98313,#98314));
#98726=CLOSED_SHELL('',(#98315,#98316,#98317,#98318,#98319,#98320,#98321,
#98322,#98323,#98324));
#98727=CLOSED_SHELL('',(#98325,#98326,#98327,#98328,#98329,#98330,#98331,
#98332,#98333,#98334,#98335,#98336,#98337,#98338,#98339,#98340,#98341,#98342,
#98343,#98344,#98345,#98346,#98347,#98348,#98349,#98350,#98351,#98352,#98353,
#98354,#98355,#98356,#98357,#98358,#98359,#98360,#98361,#98362,#98363,#98364,
#98365,#98366,#98367,#98368,#98369,#98370,#98371,#98372,#98373,#98374,#98375,
#98376,#98377,#98378,#98379,#98380,#98381,#98382));
#98728=CLOSED_SHELL('',(#98383,#98384,#98385,#98386,#98387,#98388,#98389,
#98390,#98391,#98392,#98393,#98394,#98395,#98396,#98397,#98398,#98399,#98400));
#98729=CLOSED_SHELL('',(#98401,#98402,#98403,#98404,#98405,#98406,#98407,
#98408,#98409,#98410));
#98730=CLOSED_SHELL('',(#98411,#98412,#98413,#98414,#98415,#98416,#98417,
#98418,#98419,#98420,#98421,#98422,#98423,#98424,#98425,#98426,#98427,#98428));
#98731=CLOSED_SHELL('',(#98429,#98430,#98431,#98432,#98433,#98434,#98435,
#98436,#98437,#98438));
#98732=CLOSED_SHELL('',(#98439,#98440,#98441,#98442,#98443,#98444,#98445,
#98446,#98447,#98448,#98449,#98450,#98451,#98452,#98453,#98454,#98455,#98456));
#98733=CLOSED_SHELL('',(#98457,#98458,#98459,#98460,#98461,#98462,#98463,
#98464,#98465,#98466));
#98734=CLOSED_SHELL('',(#98467,#98468,#98469,#98470,#98471,#98472,#98473,
#98474,#98475,#98476,#98477,#98478,#98479,#98480,#98481,#98482,#98483,#98484,
#98485,#98486,#98487,#98488,#98489,#98490,#98491,#98492,#98493,#98494,#98495,
#98496,#98497,#98498,#98499,#98500,#98501,#98502,#98503,#98504,#98505,#98506,
#98507,#98508,#98509,#98510,#98511,#98512,#98513,#98514,#98515,#98516,#98517,
#98518,#98519,#98520,#98521,#98522,#98523,#98524,#98525,#98526,#98527,#98528,
#98529,#98530,#98531,#98532,#98533,#98534,#98535,#98536,#98537,#98538,#98539,
#98540,#98541,#98542,#98543,#98544,#98545,#98546,#98547,#98548,#98549,#98550,
#98551,#98552,#98553,#98554,#98555,#98556,#98557,#98558,#98559,#98560,#98561,
#98562,#98563,#98564,#98565,#98566,#98567,#98568,#98569,#98570,#98571,#98572,
#98573,#98574,#98575,#98576,#98577,#98578,#98579,#98580,#98581,#98582,#98583,
#98584,#98585,#98586,#98587,#98588,#98589,#98590,#98591,#98592,#98593,#98594,
#98595,#98596,#98597,#98598,#98599,#98600,#98601,#98602,#98603,#98604,#98605,
#98606,#98607,#98608,#98609,#98610,#98611,#98612,#98613,#98614,#98615,#98616,
#98617,#98618,#98619,#98620,#98621,#98622,#98623,#98624,#98625,#98626,#98627,
#98628,#98629,#98630,#98631,#98632,#98633,#98634,#98635,#98636,#98637,#98638,
#98639,#98640,#98641,#98642,#98643,#98644,#98645,#98646,#98647,#98648,#98649,
#98650,#98651,#98652,#98653,#98654,#98655,#98656,#98657,#98658,#98659,#98660,
#98661,#98662,#98663,#98664,#98665,#98666,#98667,#98668,#98669,#98670,#98671,
#98672,#98673,#98674,#98675,#98676,#98677,#98678,#98679,#98680,#98681,#98682,
#98683,#98684,#98685,#98686,#98687,#98688,#98689,#98690,#98691,#98692,#98693,
#98694,#98695,#98696));
#110986=AXIS2_PLACEMENT_3D('',#274150,#140414,#140415);
#110987=AXIS2_PLACEMENT_3D('',#274151,#140416,#140417);
#110988=AXIS2_PLACEMENT_3D('',#274154,#140418,#140419);
#110989=AXIS2_PLACEMENT_3D('',#274158,#140421,#140422);
#110990=AXIS2_PLACEMENT_3D('',#274160,#140424,#140425);
#110991=AXIS2_PLACEMENT_3D('',#274163,#140426,#140427);
#110992=AXIS2_PLACEMENT_3D('',#274167,#140429,#140430);
#110993=AXIS2_PLACEMENT_3D('',#274171,#140432,#140433);
#110994=AXIS2_PLACEMENT_3D('',#274175,#140435,#140436);
#110995=AXIS2_PLACEMENT_3D('',#274179,#140438,#140439);
#110996=AXIS2_PLACEMENT_3D('',#274183,#140441,#140442);
#110997=AXIS2_PLACEMENT_3D('',#274187,#140444,#140445);
#110998=AXIS2_PLACEMENT_3D('',#274190,#140448,#140449);
#110999=AXIS2_PLACEMENT_3D('',#274194,#140452,#140453);
#111000=AXIS2_PLACEMENT_3D('',#274198,#140456,#140457);
#111001=AXIS2_PLACEMENT_3D('',#274201,#140459,#140460);
#111002=AXIS2_PLACEMENT_3D('',#274202,#140461,#140462);
#111003=AXIS2_PLACEMENT_3D('',#274206,#140465,#140466);
#111004=AXIS2_PLACEMENT_3D('',#274209,#140468,#140469);
#111005=AXIS2_PLACEMENT_3D('',#274210,#140470,#140471);
#111006=AXIS2_PLACEMENT_3D('',#274214,#140474,#140475);
#111007=AXIS2_PLACEMENT_3D('',#274217,#140477,#140478);
#111008=AXIS2_PLACEMENT_3D('',#274218,#140479,#140480);
#111009=AXIS2_PLACEMENT_3D('',#274222,#140483,#140484);
#111010=AXIS2_PLACEMENT_3D('',#274225,#140486,#140487);
#111011=AXIS2_PLACEMENT_3D('',#274226,#140488,#140489);
#111012=AXIS2_PLACEMENT_3D('',#274230,#140492,#140493);
#111013=AXIS2_PLACEMENT_3D('',#274233,#140495,#140496);
#111014=AXIS2_PLACEMENT_3D('',#274234,#140497,#140498);
#111015=AXIS2_PLACEMENT_3D('',#274238,#140501,#140502);
#111016=AXIS2_PLACEMENT_3D('',#274241,#140504,#140505);
#111017=AXIS2_PLACEMENT_3D('',#274242,#140506,#140507);
#111018=AXIS2_PLACEMENT_3D('',#274246,#140510,#140511);
#111019=AXIS2_PLACEMENT_3D('',#274247,#140512,#140513);
#111020=AXIS2_PLACEMENT_3D('',#274248,#140514,#140515);
#111021=AXIS2_PLACEMENT_3D('',#274249,#140516,#140517);
#111022=AXIS2_PLACEMENT_3D('',#274252,#140518,#140519);
#111023=AXIS2_PLACEMENT_3D('',#274256,#140521,#140522);
#111024=AXIS2_PLACEMENT_3D('',#274260,#140524,#140525);
#111025=AXIS2_PLACEMENT_3D('',#274264,#140527,#140528);
#111026=AXIS2_PLACEMENT_3D('',#274266,#140530,#140531);
#111027=AXIS2_PLACEMENT_3D('',#274272,#140535,#140536);
#111028=AXIS2_PLACEMENT_3D('',#274275,#140538,#140539);
#111029=AXIS2_PLACEMENT_3D('',#274276,#140540,#140541);
#111030=AXIS2_PLACEMENT_3D('',#274280,#140544,#140545);
#111031=AXIS2_PLACEMENT_3D('',#274283,#140547,#140548);
#111032=AXIS2_PLACEMENT_3D('',#274284,#140549,#140550);
#111033=AXIS2_PLACEMENT_3D('',#274288,#140553,#140554);
#111034=AXIS2_PLACEMENT_3D('',#274291,#140556,#140557);
#111035=AXIS2_PLACEMENT_3D('',#274292,#140558,#140559);
#111036=AXIS2_PLACEMENT_3D('',#274296,#140562,#140563);
#111037=AXIS2_PLACEMENT_3D('',#274297,#140564,#140565);
#111038=AXIS2_PLACEMENT_3D('',#274298,#140566,#140567);
#111039=AXIS2_PLACEMENT_3D('',#274299,#140568,#140569);
#111040=AXIS2_PLACEMENT_3D('',#274302,#140570,#140571);
#111041=AXIS2_PLACEMENT_3D('',#274306,#140573,#140574);
#111042=AXIS2_PLACEMENT_3D('',#274310,#140576,#140577);
#111043=AXIS2_PLACEMENT_3D('',#274314,#140579,#140580);
#111044=AXIS2_PLACEMENT_3D('',#274322,#140584,#140585);
#111045=AXIS2_PLACEMENT_3D('',#274326,#140587,#140588);
#111046=AXIS2_PLACEMENT_3D('',#274330,#140590,#140591);
#111047=AXIS2_PLACEMENT_3D('',#274334,#140593,#140594);
#111048=AXIS2_PLACEMENT_3D('',#274338,#140596,#140597);
#111049=AXIS2_PLACEMENT_3D('',#274342,#140599,#140600);
#111050=AXIS2_PLACEMENT_3D('',#274350,#140604,#140605);
#111051=AXIS2_PLACEMENT_3D('',#274354,#140607,#140608);
#111052=AXIS2_PLACEMENT_3D('',#274358,#140610,#140611);
#111053=AXIS2_PLACEMENT_3D('',#274362,#140613,#140614);
#111054=AXIS2_PLACEMENT_3D('',#274366,#140616,#140617);
#111055=AXIS2_PLACEMENT_3D('',#274370,#140619,#140620);
#111056=AXIS2_PLACEMENT_3D('',#274378,#140624,#140625);
#111057=AXIS2_PLACEMENT_3D('',#274382,#140627,#140628);
#111058=AXIS2_PLACEMENT_3D('',#274386,#140630,#140631);
#111059=AXIS2_PLACEMENT_3D('',#274390,#140633,#140634);
#111060=AXIS2_PLACEMENT_3D('',#274394,#140636,#140637);
#111061=AXIS2_PLACEMENT_3D('',#274398,#140639,#140640);
#111062=AXIS2_PLACEMENT_3D('',#274406,#140644,#140645);
#111063=AXIS2_PLACEMENT_3D('',#274410,#140647,#140648);
#111064=AXIS2_PLACEMENT_3D('',#274412,#140650,#140651);
#111065=AXIS2_PLACEMENT_3D('',#274415,#140652,#140653);
#111066=AXIS2_PLACEMENT_3D('',#274419,#140655,#140656);
#111067=AXIS2_PLACEMENT_3D('',#274423,#140658,#140659);
#111068=AXIS2_PLACEMENT_3D('',#274427,#140661,#140662);
#111069=AXIS2_PLACEMENT_3D('',#274435,#140666,#140667);
#111070=AXIS2_PLACEMENT_3D('',#274439,#140669,#140670);
#111071=AXIS2_PLACEMENT_3D('',#274443,#140672,#140673);
#111072=AXIS2_PLACEMENT_3D('',#274447,#140675,#140676);
#111073=AXIS2_PLACEMENT_3D('',#274451,#140678,#140679);
#111074=AXIS2_PLACEMENT_3D('',#274455,#140681,#140682);
#111075=AXIS2_PLACEMENT_3D('',#274463,#140686,#140687);
#111076=AXIS2_PLACEMENT_3D('',#274467,#140689,#140690);
#111077=AXIS2_PLACEMENT_3D('',#274471,#140692,#140693);
#111078=AXIS2_PLACEMENT_3D('',#274475,#140695,#140696);
#111079=AXIS2_PLACEMENT_3D('',#274479,#140698,#140699);
#111080=AXIS2_PLACEMENT_3D('',#274483,#140701,#140702);
#111081=AXIS2_PLACEMENT_3D('',#274491,#140706,#140707);
#111082=AXIS2_PLACEMENT_3D('',#274495,#140709,#140710);
#111083=AXIS2_PLACEMENT_3D('',#274499,#140712,#140713);
#111084=AXIS2_PLACEMENT_3D('',#274503,#140715,#140716);
#111085=AXIS2_PLACEMENT_3D('',#274507,#140718,#140719);
#111086=AXIS2_PLACEMENT_3D('',#274511,#140721,#140722);
#111087=AXIS2_PLACEMENT_3D('',#274519,#140726,#140727);
#111088=AXIS2_PLACEMENT_3D('',#274523,#140729,#140730);
#111089=AXIS2_PLACEMENT_3D('',#274525,#140732,#140733);
#111090=AXIS2_PLACEMENT_3D('',#274528,#140736,#140737);
#111091=AXIS2_PLACEMENT_3D('',#274530,#140739,#140740);
#111092=AXIS2_PLACEMENT_3D('',#274532,#140742,#140743);
#111093=AXIS2_PLACEMENT_3D('',#274534,#140745,#140746);
#111094=AXIS2_PLACEMENT_3D('',#274536,#140748,#140749);
#111095=AXIS2_PLACEMENT_3D('',#274538,#140751,#140752);
#111096=AXIS2_PLACEMENT_3D('',#274540,#140754,#140755);
#111097=AXIS2_PLACEMENT_3D('',#274542,#140757,#140758);
#111098=AXIS2_PLACEMENT_3D('',#274544,#140760,#140761);
#111099=AXIS2_PLACEMENT_3D('',#274546,#140763,#140764);
#111100=AXIS2_PLACEMENT_3D('',#274548,#140766,#140767);
#111101=AXIS2_PLACEMENT_3D('',#274550,#140769,#140770);
#111102=AXIS2_PLACEMENT_3D('',#274552,#140772,#140773);
#111103=AXIS2_PLACEMENT_3D('',#274554,#140775,#140776);
#111104=AXIS2_PLACEMENT_3D('',#274556,#140778,#140779);
#111105=AXIS2_PLACEMENT_3D('',#274558,#140781,#140782);
#111106=AXIS2_PLACEMENT_3D('',#274560,#140784,#140785);
#111107=AXIS2_PLACEMENT_3D('',#274562,#140787,#140788);
#111108=AXIS2_PLACEMENT_3D('',#274564,#140790,#140791);
#111109=AXIS2_PLACEMENT_3D('',#274566,#140793,#140794);
#111110=AXIS2_PLACEMENT_3D('',#274568,#140796,#140797);
#111111=AXIS2_PLACEMENT_3D('',#274570,#140799,#140800);
#111112=AXIS2_PLACEMENT_3D('',#274572,#140802,#140803);
#111113=AXIS2_PLACEMENT_3D('',#274574,#140805,#140806);
#111114=AXIS2_PLACEMENT_3D('',#274576,#140808,#140809);
#111115=AXIS2_PLACEMENT_3D('',#274578,#140811,#140812);
#111116=AXIS2_PLACEMENT_3D('',#274580,#140814,#140815);
#111117=AXIS2_PLACEMENT_3D('',#274582,#140817,#140818);
#111118=AXIS2_PLACEMENT_3D('',#274584,#140820,#140821);
#111119=AXIS2_PLACEMENT_3D('',#274586,#140823,#140824);
#111120=AXIS2_PLACEMENT_3D('',#274588,#140826,#140827);
#111121=AXIS2_PLACEMENT_3D('',#274590,#140829,#140830);
#111122=AXIS2_PLACEMENT_3D('',#274592,#140832,#140833);
#111123=AXIS2_PLACEMENT_3D('',#274594,#140835,#140836);
#111124=AXIS2_PLACEMENT_3D('',#274596,#140838,#140839);
#111125=AXIS2_PLACEMENT_3D('',#274598,#140841,#140842);
#111126=AXIS2_PLACEMENT_3D('',#274600,#140844,#140845);
#111127=AXIS2_PLACEMENT_3D('',#274602,#140847,#140848);
#111128=AXIS2_PLACEMENT_3D('',#274604,#140850,#140851);
#111129=AXIS2_PLACEMENT_3D('',#274606,#140853,#140854);
#111130=AXIS2_PLACEMENT_3D('',#274608,#140856,#140857);
#111131=AXIS2_PLACEMENT_3D('',#274610,#140859,#140860);
#111132=AXIS2_PLACEMENT_3D('',#274612,#140862,#140863);
#111133=AXIS2_PLACEMENT_3D('',#274614,#140865,#140866);
#111134=AXIS2_PLACEMENT_3D('',#274616,#140868,#140869);
#111135=AXIS2_PLACEMENT_3D('',#274618,#140871,#140872);
#111136=AXIS2_PLACEMENT_3D('',#274620,#140874,#140875);
#111137=AXIS2_PLACEMENT_3D('',#274622,#140877,#140878);
#111138=AXIS2_PLACEMENT_3D('',#274624,#140880,#140881);
#111139=AXIS2_PLACEMENT_3D('',#274626,#140883,#140884);
#111140=AXIS2_PLACEMENT_3D('',#274628,#140886,#140887);
#111141=AXIS2_PLACEMENT_3D('',#274630,#140889,#140890);
#111142=AXIS2_PLACEMENT_3D('',#274632,#140892,#140893);
#111143=AXIS2_PLACEMENT_3D('',#274634,#140895,#140896);
#111144=AXIS2_PLACEMENT_3D('',#274636,#140898,#140899);
#111145=AXIS2_PLACEMENT_3D('',#274637,#140900,#140901);
#111146=AXIS2_PLACEMENT_3D('',#274640,#140902,#140903);
#111147=AXIS2_PLACEMENT_3D('',#274644,#140905,#140906);
#111148=AXIS2_PLACEMENT_3D('',#274646,#140908,#140909);
#111149=AXIS2_PLACEMENT_3D('',#274649,#140910,#140911);
#111150=AXIS2_PLACEMENT_3D('',#274653,#140913,#140914);
#111151=AXIS2_PLACEMENT_3D('',#274657,#140916,#140917);
#111152=AXIS2_PLACEMENT_3D('',#274662,#140920,#140921);
#111153=AXIS2_PLACEMENT_3D('',#274666,#140923,#140924);
#111154=AXIS2_PLACEMENT_3D('',#274670,#140926,#140927);
#111155=AXIS2_PLACEMENT_3D('',#274674,#140929,#140930);
#111156=AXIS2_PLACEMENT_3D('',#274676,#140932,#140933);
#111157=AXIS2_PLACEMENT_3D('',#274682,#140937,#140938);
#111158=AXIS2_PLACEMENT_3D('',#274685,#140940,#140941);
#111159=AXIS2_PLACEMENT_3D('',#274686,#140942,#140943);
#111160=AXIS2_PLACEMENT_3D('',#274690,#140946,#140947);
#111161=AXIS2_PLACEMENT_3D('',#274693,#140949,#140950);
#111162=AXIS2_PLACEMENT_3D('',#274694,#140951,#140952);
#111163=AXIS2_PLACEMENT_3D('',#274698,#140955,#140956);
#111164=AXIS2_PLACEMENT_3D('',#274701,#140958,#140959);
#111165=AXIS2_PLACEMENT_3D('',#274702,#140960,#140961);
#111166=AXIS2_PLACEMENT_3D('',#274706,#140964,#140965);
#111167=AXIS2_PLACEMENT_3D('',#274709,#140967,#140968);
#111168=AXIS2_PLACEMENT_3D('',#274710,#140969,#140970);
#111169=AXIS2_PLACEMENT_3D('',#274712,#140972,#140973);
#111170=AXIS2_PLACEMENT_3D('',#274716,#140976,#140977);
#111171=AXIS2_PLACEMENT_3D('',#274719,#140979,#140980);
#111172=AXIS2_PLACEMENT_3D('',#274720,#140981,#140982);
#111173=AXIS2_PLACEMENT_3D('',#274724,#140985,#140986);
#111174=AXIS2_PLACEMENT_3D('',#274727,#140988,#140989);
#111175=AXIS2_PLACEMENT_3D('',#274728,#140990,#140991);
#111176=AXIS2_PLACEMENT_3D('',#274732,#140994,#140995);
#111177=AXIS2_PLACEMENT_3D('',#274733,#140996,#140997);
#111178=AXIS2_PLACEMENT_3D('',#274734,#140998,#140999);
#111179=AXIS2_PLACEMENT_3D('',#274735,#141000,#141001);
#111180=AXIS2_PLACEMENT_3D('',#274738,#141002,#141003);
#111181=AXIS2_PLACEMENT_3D('',#274742,#141005,#141006);
#111182=AXIS2_PLACEMENT_3D('',#274746,#141008,#141009);
#111183=AXIS2_PLACEMENT_3D('',#274750,#141011,#141012);
#111184=AXIS2_PLACEMENT_3D('',#274752,#141014,#141015);
#111185=AXIS2_PLACEMENT_3D('',#274758,#141019,#141020);
#111186=AXIS2_PLACEMENT_3D('',#274761,#141022,#141023);
#111187=AXIS2_PLACEMENT_3D('',#274762,#141024,#141025);
#111188=AXIS2_PLACEMENT_3D('',#274766,#141028,#141029);
#111189=AXIS2_PLACEMENT_3D('',#274769,#141031,#141032);
#111190=AXIS2_PLACEMENT_3D('',#274770,#141033,#141034);
#111191=AXIS2_PLACEMENT_3D('',#274774,#141037,#141038);
#111192=AXIS2_PLACEMENT_3D('',#274777,#141040,#141041);
#111193=AXIS2_PLACEMENT_3D('',#274778,#141042,#141043);
#111194=AXIS2_PLACEMENT_3D('',#274782,#141046,#141047);
#111195=AXIS2_PLACEMENT_3D('',#274783,#141048,#141049);
#111196=AXIS2_PLACEMENT_3D('',#274784,#141050,#141051);
#111197=AXIS2_PLACEMENT_3D('',#274785,#141052,#141053);
#111198=AXIS2_PLACEMENT_3D('',#274788,#141054,#141055);
#111199=AXIS2_PLACEMENT_3D('',#274792,#141057,#141058);
#111200=AXIS2_PLACEMENT_3D('',#274794,#141060,#141061);
#111201=AXIS2_PLACEMENT_3D('',#274797,#141062,#141063);
#111202=AXIS2_PLACEMENT_3D('',#274802,#141066,#141067);
#111203=AXIS2_PLACEMENT_3D('',#274806,#141069,#141070);
#111204=AXIS2_PLACEMENT_3D('',#274810,#141072,#141073);
#111205=AXIS2_PLACEMENT_3D('',#274814,#141075,#141076);
#111206=AXIS2_PLACEMENT_3D('',#274818,#141078,#141079);
#111207=AXIS2_PLACEMENT_3D('',#274822,#141081,#141082);
#111208=AXIS2_PLACEMENT_3D('',#274824,#141084,#141085);
#111209=AXIS2_PLACEMENT_3D('',#274830,#141089,#141090);
#111210=AXIS2_PLACEMENT_3D('',#274833,#141092,#141093);
#111211=AXIS2_PLACEMENT_3D('',#274834,#141094,#141095);
#111212=AXIS2_PLACEMENT_3D('',#274838,#141098,#141099);
#111213=AXIS2_PLACEMENT_3D('',#274841,#141101,#141102);
#111214=AXIS2_PLACEMENT_3D('',#274842,#141103,#141104);
#111215=AXIS2_PLACEMENT_3D('',#274846,#141107,#141108);
#111216=AXIS2_PLACEMENT_3D('',#274849,#141110,#141111);
#111217=AXIS2_PLACEMENT_3D('',#274850,#141112,#141113);
#111218=AXIS2_PLACEMENT_3D('',#274854,#141116,#141117);
#111219=AXIS2_PLACEMENT_3D('',#274857,#141119,#141120);
#111220=AXIS2_PLACEMENT_3D('',#274858,#141121,#141122);
#111221=AXIS2_PLACEMENT_3D('',#274862,#141125,#141126);
#111222=AXIS2_PLACEMENT_3D('',#274865,#141128,#141129);
#111223=AXIS2_PLACEMENT_3D('',#274866,#141130,#141131);
#111224=AXIS2_PLACEMENT_3D('',#274870,#141134,#141135);
#111225=AXIS2_PLACEMENT_3D('',#274873,#141137,#141138);
#111226=AXIS2_PLACEMENT_3D('',#274874,#141139,#141140);
#111227=AXIS2_PLACEMENT_3D('',#274876,#141142,#141143);
#111228=AXIS2_PLACEMENT_3D('',#274880,#141146,#141147);
#111229=AXIS2_PLACEMENT_3D('',#274881,#141148,#141149);
#111230=AXIS2_PLACEMENT_3D('',#274882,#141150,#141151);
#111231=AXIS2_PLACEMENT_3D('',#274883,#141152,#141153);
#111232=AXIS2_PLACEMENT_3D('',#274886,#141154,#141155);
#111233=AXIS2_PLACEMENT_3D('',#274890,#141157,#141158);
#111234=AXIS2_PLACEMENT_3D('',#274894,#141160,#141161);
#111235=AXIS2_PLACEMENT_3D('',#274898,#141163,#141164);
#111236=AXIS2_PLACEMENT_3D('',#274900,#141166,#141167);
#111237=AXIS2_PLACEMENT_3D('',#274906,#141171,#141172);
#111238=AXIS2_PLACEMENT_3D('',#274909,#141174,#141175);
#111239=AXIS2_PLACEMENT_3D('',#274910,#141176,#141177);
#111240=AXIS2_PLACEMENT_3D('',#274914,#141180,#141181);
#111241=AXIS2_PLACEMENT_3D('',#274917,#141183,#141184);
#111242=AXIS2_PLACEMENT_3D('',#274918,#141185,#141186);
#111243=AXIS2_PLACEMENT_3D('',#274922,#141189,#141190);
#111244=AXIS2_PLACEMENT_3D('',#274925,#141192,#141193);
#111245=AXIS2_PLACEMENT_3D('',#274926,#141194,#141195);
#111246=AXIS2_PLACEMENT_3D('',#274930,#141198,#141199);
#111247=AXIS2_PLACEMENT_3D('',#274931,#141200,#141201);
#111248=AXIS2_PLACEMENT_3D('',#274932,#141202,#141203);
#111249=AXIS2_PLACEMENT_3D('',#274933,#141204,#141205);
#111250=AXIS2_PLACEMENT_3D('',#274936,#141206,#141207);
#111251=AXIS2_PLACEMENT_3D('',#274940,#141209,#141210);
#111252=AXIS2_PLACEMENT_3D('',#274942,#141212,#141213);
#111253=AXIS2_PLACEMENT_3D('',#274945,#141214,#141215);
#111254=AXIS2_PLACEMENT_3D('',#274950,#141218,#141219);
#111255=AXIS2_PLACEMENT_3D('',#274954,#141221,#141222);
#111256=AXIS2_PLACEMENT_3D('',#274958,#141224,#141225);
#111257=AXIS2_PLACEMENT_3D('',#274962,#141227,#141228);
#111258=AXIS2_PLACEMENT_3D('',#274966,#141230,#141231);
#111259=AXIS2_PLACEMENT_3D('',#274970,#141233,#141234);
#111260=AXIS2_PLACEMENT_3D('',#274972,#141236,#141237);
#111261=AXIS2_PLACEMENT_3D('',#274978,#141241,#141242);
#111262=AXIS2_PLACEMENT_3D('',#274981,#141244,#141245);
#111263=AXIS2_PLACEMENT_3D('',#274982,#141246,#141247);
#111264=AXIS2_PLACEMENT_3D('',#274986,#141250,#141251);
#111265=AXIS2_PLACEMENT_3D('',#274989,#141253,#141254);
#111266=AXIS2_PLACEMENT_3D('',#274990,#141255,#141256);
#111267=AXIS2_PLACEMENT_3D('',#274994,#141259,#141260);
#111268=AXIS2_PLACEMENT_3D('',#274997,#141262,#141263);
#111269=AXIS2_PLACEMENT_3D('',#274998,#141264,#141265);
#111270=AXIS2_PLACEMENT_3D('',#275002,#141268,#141269);
#111271=AXIS2_PLACEMENT_3D('',#275005,#141271,#141272);
#111272=AXIS2_PLACEMENT_3D('',#275006,#141273,#141274);
#111273=AXIS2_PLACEMENT_3D('',#275010,#141277,#141278);
#111274=AXIS2_PLACEMENT_3D('',#275013,#141280,#141281);
#111275=AXIS2_PLACEMENT_3D('',#275014,#141282,#141283);
#111276=AXIS2_PLACEMENT_3D('',#275018,#141286,#141287);
#111277=AXIS2_PLACEMENT_3D('',#275021,#141289,#141290);
#111278=AXIS2_PLACEMENT_3D('',#275022,#141291,#141292);
#111279=AXIS2_PLACEMENT_3D('',#275024,#141294,#141295);
#111280=AXIS2_PLACEMENT_3D('',#275028,#141298,#141299);
#111281=AXIS2_PLACEMENT_3D('',#275029,#141300,#141301);
#111282=AXIS2_PLACEMENT_3D('',#275030,#141302,#141303);
#111283=AXIS2_PLACEMENT_3D('',#275031,#141304,#141305);
#111284=AXIS2_PLACEMENT_3D('',#275034,#141306,#141307);
#111285=AXIS2_PLACEMENT_3D('',#275038,#141309,#141310);
#111286=AXIS2_PLACEMENT_3D('',#275042,#141312,#141313);
#111287=AXIS2_PLACEMENT_3D('',#275046,#141315,#141316);
#111288=AXIS2_PLACEMENT_3D('',#275048,#141318,#141319);
#111289=AXIS2_PLACEMENT_3D('',#275054,#141323,#141324);
#111290=AXIS2_PLACEMENT_3D('',#275057,#141326,#141327);
#111291=AXIS2_PLACEMENT_3D('',#275058,#141328,#141329);
#111292=AXIS2_PLACEMENT_3D('',#275062,#141332,#141333);
#111293=AXIS2_PLACEMENT_3D('',#275065,#141335,#141336);
#111294=AXIS2_PLACEMENT_3D('',#275066,#141337,#141338);
#111295=AXIS2_PLACEMENT_3D('',#275070,#141341,#141342);
#111296=AXIS2_PLACEMENT_3D('',#275073,#141344,#141345);
#111297=AXIS2_PLACEMENT_3D('',#275074,#141346,#141347);
#111298=AXIS2_PLACEMENT_3D('',#275078,#141350,#141351);
#111299=AXIS2_PLACEMENT_3D('',#275079,#141352,#141353);
#111300=AXIS2_PLACEMENT_3D('',#275080,#141354,#141355);
#111301=AXIS2_PLACEMENT_3D('',#275081,#141356,#141357);
#111302=AXIS2_PLACEMENT_3D('',#275090,#141362,#141363);
#111303=AXIS2_PLACEMENT_3D('',#275099,#141368,#141369);
#111304=AXIS2_PLACEMENT_3D('',#275108,#141374,#141375);
#111305=AXIS2_PLACEMENT_3D('',#275114,#141379,#141380);
#111306=AXIS2_PLACEMENT_3D('',#275120,#141384,#141385);
#111307=AXIS2_PLACEMENT_3D('',#275122,#141386,#141387);
#111308=AXIS2_PLACEMENT_3D('',#275124,#141388,#141389);
#111309=AXIS2_PLACEMENT_3D('',#275126,#141391,#141392);
#111310=AXIS2_PLACEMENT_3D('',#275132,#141396,#141397);
#111311=AXIS2_PLACEMENT_3D('',#275134,#141398,#141399);
#111312=AXIS2_PLACEMENT_3D('',#275136,#141400,#141401);
#111313=AXIS2_PLACEMENT_3D('',#275138,#141403,#141404);
#111314=AXIS2_PLACEMENT_3D('',#275144,#141408,#141409);
#111315=AXIS2_PLACEMENT_3D('',#275146,#141410,#141411);
#111316=AXIS2_PLACEMENT_3D('',#275148,#141412,#141413);
#111317=AXIS2_PLACEMENT_3D('',#275150,#141415,#141416);
#111318=AXIS2_PLACEMENT_3D('',#275156,#141420,#141421);
#111319=AXIS2_PLACEMENT_3D('',#275158,#141422,#141423);
#111320=AXIS2_PLACEMENT_3D('',#275160,#141424,#141425);
#111321=AXIS2_PLACEMENT_3D('',#275162,#141427,#141428);
#111322=AXIS2_PLACEMENT_3D('',#275168,#141432,#141433);
#111323=AXIS2_PLACEMENT_3D('',#275174,#141437,#141438);
#111324=AXIS2_PLACEMENT_3D('',#275180,#141442,#141443);
#111325=AXIS2_PLACEMENT_3D('',#275186,#141447,#141448);
#111326=AXIS2_PLACEMENT_3D('',#275195,#141453,#141454);
#111327=AXIS2_PLACEMENT_3D('',#275201,#141458,#141459);
#111328=AXIS2_PLACEMENT_3D('',#275207,#141463,#141464);
#111329=AXIS2_PLACEMENT_3D('',#275213,#141468,#141469);
#111330=AXIS2_PLACEMENT_3D('',#275215,#141470,#141471);
#111331=AXIS2_PLACEMENT_3D('',#275217,#141472,#141473);
#111332=AXIS2_PLACEMENT_3D('',#275219,#141475,#141476);
#111333=AXIS2_PLACEMENT_3D('',#275225,#141480,#141481);
#111334=AXIS2_PLACEMENT_3D('',#275227,#141482,#141483);
#111335=AXIS2_PLACEMENT_3D('',#275229,#141484,#141485);
#111336=AXIS2_PLACEMENT_3D('',#275231,#141487,#141488);
#111337=AXIS2_PLACEMENT_3D('',#275237,#141492,#141493);
#111338=AXIS2_PLACEMENT_3D('',#275239,#141494,#141495);
#111339=AXIS2_PLACEMENT_3D('',#275241,#141496,#141497);
#111340=AXIS2_PLACEMENT_3D('',#275243,#141499,#141500);
#111341=AXIS2_PLACEMENT_3D('',#275249,#141504,#141505);
#111342=AXIS2_PLACEMENT_3D('',#275251,#141506,#141507);
#111343=AXIS2_PLACEMENT_3D('',#275253,#141508,#141509);
#111344=AXIS2_PLACEMENT_3D('',#275255,#141511,#141512);
#111345=AXIS2_PLACEMENT_3D('',#275261,#141516,#141517);
#111346=AXIS2_PLACEMENT_3D('',#275267,#141521,#141522);
#111347=AXIS2_PLACEMENT_3D('',#275273,#141526,#141527);
#111348=AXIS2_PLACEMENT_3D('',#275279,#141531,#141532);
#111349=AXIS2_PLACEMENT_3D('',#275281,#141533,#141534);
#111350=AXIS2_PLACEMENT_3D('',#275283,#141535,#141536);
#111351=AXIS2_PLACEMENT_3D('',#275285,#141538,#141539);
#111352=AXIS2_PLACEMENT_3D('',#275291,#141543,#141544);
#111353=AXIS2_PLACEMENT_3D('',#275293,#141545,#141546);
#111354=AXIS2_PLACEMENT_3D('',#275295,#141547,#141548);
#111355=AXIS2_PLACEMENT_3D('',#275297,#141550,#141551);
#111356=AXIS2_PLACEMENT_3D('',#275303,#141555,#141556);
#111357=AXIS2_PLACEMENT_3D('',#275304,#141557,#141558);
#111358=AXIS2_PLACEMENT_3D('',#275305,#141559,#141560);
#111359=AXIS2_PLACEMENT_3D('',#275306,#141561,#141562);
#111360=AXIS2_PLACEMENT_3D('',#275315,#141567,#141568);
#111361=AXIS2_PLACEMENT_3D('',#275317,#141569,#141570);
#111362=AXIS2_PLACEMENT_3D('',#275319,#141571,#141572);
#111363=AXIS2_PLACEMENT_3D('',#275321,#141574,#141575);
#111364=AXIS2_PLACEMENT_3D('',#275327,#141579,#141580);
#111365=AXIS2_PLACEMENT_3D('',#275333,#141584,#141585);
#111366=AXIS2_PLACEMENT_3D('',#275339,#141589,#141590);
#111367=AXIS2_PLACEMENT_3D('',#275345,#141594,#141595);
#111368=AXIS2_PLACEMENT_3D('',#275347,#141596,#141597);
#111369=AXIS2_PLACEMENT_3D('',#275349,#141598,#141599);
#111370=AXIS2_PLACEMENT_3D('',#275351,#141601,#141602);
#111371=AXIS2_PLACEMENT_3D('',#275357,#141606,#141607);
#111372=AXIS2_PLACEMENT_3D('',#275363,#141611,#141612);
#111373=AXIS2_PLACEMENT_3D('',#275369,#141616,#141617);
#111374=AXIS2_PLACEMENT_3D('',#275375,#141621,#141622);
#111375=AXIS2_PLACEMENT_3D('',#275377,#141623,#141624);
#111376=AXIS2_PLACEMENT_3D('',#275379,#141625,#141626);
#111377=AXIS2_PLACEMENT_3D('',#275381,#141628,#141629);
#111378=AXIS2_PLACEMENT_3D('',#275387,#141633,#141634);
#111379=AXIS2_PLACEMENT_3D('',#275389,#141635,#141636);
#111380=AXIS2_PLACEMENT_3D('',#275391,#141637,#141638);
#111381=AXIS2_PLACEMENT_3D('',#275393,#141640,#141641);
#111382=AXIS2_PLACEMENT_3D('',#275399,#141645,#141646);
#111383=AXIS2_PLACEMENT_3D('',#275401,#141647,#141648);
#111384=AXIS2_PLACEMENT_3D('',#275403,#141649,#141650);
#111385=AXIS2_PLACEMENT_3D('',#275405,#141652,#141653);
#111386=AXIS2_PLACEMENT_3D('',#275411,#141657,#141658);
#111387=AXIS2_PLACEMENT_3D('',#275413,#141659,#141660);
#111388=AXIS2_PLACEMENT_3D('',#275415,#141661,#141662);
#111389=AXIS2_PLACEMENT_3D('',#275417,#141664,#141665);
#111390=AXIS2_PLACEMENT_3D('',#275420,#141668,#141669);
#111391=AXIS2_PLACEMENT_3D('',#275429,#141674,#141675);
#111392=AXIS2_PLACEMENT_3D('',#275435,#141679,#141680);
#111393=AXIS2_PLACEMENT_3D('',#275441,#141684,#141685);
#111394=AXIS2_PLACEMENT_3D('',#275443,#141686,#141687);
#111395=AXIS2_PLACEMENT_3D('',#275445,#141688,#141689);
#111396=AXIS2_PLACEMENT_3D('',#275447,#141691,#141692);
#111397=AXIS2_PLACEMENT_3D('',#275453,#141696,#141697);
#111398=AXIS2_PLACEMENT_3D('',#275455,#141698,#141699);
#111399=AXIS2_PLACEMENT_3D('',#275457,#141700,#141701);
#111400=AXIS2_PLACEMENT_3D('',#275459,#141703,#141704);
#111401=AXIS2_PLACEMENT_3D('',#275465,#141708,#141709);
#111402=AXIS2_PLACEMENT_3D('',#275467,#141710,#141711);
#111403=AXIS2_PLACEMENT_3D('',#275469,#141712,#141713);
#111404=AXIS2_PLACEMENT_3D('',#275471,#141715,#141716);
#111405=AXIS2_PLACEMENT_3D('',#275477,#141720,#141721);
#111406=AXIS2_PLACEMENT_3D('',#275479,#141722,#141723);
#111407=AXIS2_PLACEMENT_3D('',#275481,#141724,#141725);
#111408=AXIS2_PLACEMENT_3D('',#275483,#141727,#141728);
#111409=AXIS2_PLACEMENT_3D('',#275489,#141732,#141733);
#111410=AXIS2_PLACEMENT_3D('',#275495,#141737,#141738);
#111411=AXIS2_PLACEMENT_3D('',#275498,#141741,#141742);
#111412=AXIS2_PLACEMENT_3D('',#275507,#141747,#141748);
#111413=AXIS2_PLACEMENT_3D('',#275513,#141752,#141753);
#111414=AXIS2_PLACEMENT_3D('',#275519,#141757,#141758);
#111415=AXIS2_PLACEMENT_3D('',#275525,#141762,#141763);
#111416=AXIS2_PLACEMENT_3D('',#275527,#141764,#141765);
#111417=AXIS2_PLACEMENT_3D('',#275529,#141766,#141767);
#111418=AXIS2_PLACEMENT_3D('',#275531,#141769,#141770);
#111419=AXIS2_PLACEMENT_3D('',#275537,#141774,#141775);
#111420=AXIS2_PLACEMENT_3D('',#275539,#141776,#141777);
#111421=AXIS2_PLACEMENT_3D('',#275541,#141778,#141779);
#111422=AXIS2_PLACEMENT_3D('',#275543,#141781,#141782);
#111423=AXIS2_PLACEMENT_3D('',#275549,#141786,#141787);
#111424=AXIS2_PLACEMENT_3D('',#275551,#141788,#141789);
#111425=AXIS2_PLACEMENT_3D('',#275553,#141790,#141791);
#111426=AXIS2_PLACEMENT_3D('',#275555,#141793,#141794);
#111427=AXIS2_PLACEMENT_3D('',#275561,#141798,#141799);
#111428=AXIS2_PLACEMENT_3D('',#275563,#141800,#141801);
#111429=AXIS2_PLACEMENT_3D('',#275565,#141802,#141803);
#111430=AXIS2_PLACEMENT_3D('',#275567,#141805,#141806);
#111431=AXIS2_PLACEMENT_3D('',#275573,#141810,#141811);
#111432=AXIS2_PLACEMENT_3D('',#275579,#141815,#141816);
#111433=AXIS2_PLACEMENT_3D('',#275585,#141820,#141821);
#111434=AXIS2_PLACEMENT_3D('',#275591,#141825,#141826);
#111435=AXIS2_PLACEMENT_3D('',#275593,#141827,#141828);
#111436=AXIS2_PLACEMENT_3D('',#275595,#141829,#141830);
#111437=AXIS2_PLACEMENT_3D('',#275597,#141832,#141833);
#111438=AXIS2_PLACEMENT_3D('',#275603,#141837,#141838);
#111439=AXIS2_PLACEMENT_3D('',#275605,#141839,#141840);
#111440=AXIS2_PLACEMENT_3D('',#275607,#141841,#141842);
#111441=AXIS2_PLACEMENT_3D('',#275609,#141844,#141845);
#111442=AXIS2_PLACEMENT_3D('',#275615,#141849,#141850);
#111443=AXIS2_PLACEMENT_3D('',#275617,#141851,#141852);
#111444=AXIS2_PLACEMENT_3D('',#275619,#141853,#141854);
#111445=AXIS2_PLACEMENT_3D('',#275621,#141856,#141857);
#111446=AXIS2_PLACEMENT_3D('',#275627,#141861,#141862);
#111447=AXIS2_PLACEMENT_3D('',#275629,#141863,#141864);
#111448=AXIS2_PLACEMENT_3D('',#275631,#141865,#141866);
#111449=AXIS2_PLACEMENT_3D('',#275633,#141868,#141869);
#111450=AXIS2_PLACEMENT_3D('',#275639,#141873,#141874);
#111451=AXIS2_PLACEMENT_3D('',#275645,#141878,#141879);
#111452=AXIS2_PLACEMENT_3D('',#275651,#141883,#141884);
#111453=AXIS2_PLACEMENT_3D('',#275657,#141888,#141889);
#111454=AXIS2_PLACEMENT_3D('',#275659,#141890,#141891);
#111455=AXIS2_PLACEMENT_3D('',#275661,#141892,#141893);
#111456=AXIS2_PLACEMENT_3D('',#275663,#141895,#141896);
#111457=AXIS2_PLACEMENT_3D('',#275669,#141900,#141901);
#111458=AXIS2_PLACEMENT_3D('',#275675,#141905,#141906);
#111459=AXIS2_PLACEMENT_3D('',#275681,#141910,#141911);
#111460=AXIS2_PLACEMENT_3D('',#275687,#141915,#141916);
#111461=AXIS2_PLACEMENT_3D('',#275689,#141917,#141918);
#111462=AXIS2_PLACEMENT_3D('',#275691,#141919,#141920);
#111463=AXIS2_PLACEMENT_3D('',#275693,#141922,#141923);
#111464=AXIS2_PLACEMENT_3D('',#275699,#141927,#141928);
#111465=AXIS2_PLACEMENT_3D('',#275701,#141929,#141930);
#111466=AXIS2_PLACEMENT_3D('',#275703,#141931,#141932);
#111467=AXIS2_PLACEMENT_3D('',#275705,#141934,#141935);
#111468=AXIS2_PLACEMENT_3D('',#275711,#141939,#141940);
#111469=AXIS2_PLACEMENT_3D('',#275713,#141941,#141942);
#111470=AXIS2_PLACEMENT_3D('',#275715,#141943,#141944);
#111471=AXIS2_PLACEMENT_3D('',#275717,#141946,#141947);
#111472=AXIS2_PLACEMENT_3D('',#275723,#141951,#141952);
#111473=AXIS2_PLACEMENT_3D('',#275725,#141953,#141954);
#111474=AXIS2_PLACEMENT_3D('',#275727,#141955,#141956);
#111475=AXIS2_PLACEMENT_3D('',#275729,#141958,#141959);
#111476=AXIS2_PLACEMENT_3D('',#275732,#141962,#141963);
#111477=AXIS2_PLACEMENT_3D('',#275741,#141968,#141969);
#111478=AXIS2_PLACEMENT_3D('',#275747,#141973,#141974);
#111479=AXIS2_PLACEMENT_3D('',#275753,#141978,#141979);
#111480=AXIS2_PLACEMENT_3D('',#275755,#141980,#141981);
#111481=AXIS2_PLACEMENT_3D('',#275757,#141982,#141983);
#111482=AXIS2_PLACEMENT_3D('',#275759,#141985,#141986);
#111483=AXIS2_PLACEMENT_3D('',#275765,#141990,#141991);
#111484=AXIS2_PLACEMENT_3D('',#275767,#141992,#141993);
#111485=AXIS2_PLACEMENT_3D('',#275769,#141994,#141995);
#111486=AXIS2_PLACEMENT_3D('',#275771,#141997,#141998);
#111487=AXIS2_PLACEMENT_3D('',#275777,#142002,#142003);
#111488=AXIS2_PLACEMENT_3D('',#275779,#142004,#142005);
#111489=AXIS2_PLACEMENT_3D('',#275781,#142006,#142007);
#111490=AXIS2_PLACEMENT_3D('',#275783,#142009,#142010);
#111491=AXIS2_PLACEMENT_3D('',#275789,#142014,#142015);
#111492=AXIS2_PLACEMENT_3D('',#275791,#142016,#142017);
#111493=AXIS2_PLACEMENT_3D('',#275793,#142018,#142019);
#111494=AXIS2_PLACEMENT_3D('',#275795,#142021,#142022);
#111495=AXIS2_PLACEMENT_3D('',#275801,#142026,#142027);
#111496=AXIS2_PLACEMENT_3D('',#275807,#142031,#142032);
#111497=AXIS2_PLACEMENT_3D('',#275810,#142035,#142036);
#111498=AXIS2_PLACEMENT_3D('',#275819,#142041,#142042);
#111499=AXIS2_PLACEMENT_3D('',#275825,#142046,#142047);
#111500=AXIS2_PLACEMENT_3D('',#275831,#142051,#142052);
#111501=AXIS2_PLACEMENT_3D('',#275837,#142056,#142057);
#111502=AXIS2_PLACEMENT_3D('',#275839,#142058,#142059);
#111503=AXIS2_PLACEMENT_3D('',#275841,#142060,#142061);
#111504=AXIS2_PLACEMENT_3D('',#275843,#142063,#142064);
#111505=AXIS2_PLACEMENT_3D('',#275849,#142068,#142069);
#111506=AXIS2_PLACEMENT_3D('',#275851,#142070,#142071);
#111507=AXIS2_PLACEMENT_3D('',#275853,#142072,#142073);
#111508=AXIS2_PLACEMENT_3D('',#275855,#142075,#142076);
#111509=AXIS2_PLACEMENT_3D('',#275861,#142080,#142081);
#111510=AXIS2_PLACEMENT_3D('',#275863,#142082,#142083);
#111511=AXIS2_PLACEMENT_3D('',#275865,#142084,#142085);
#111512=AXIS2_PLACEMENT_3D('',#275867,#142087,#142088);
#111513=AXIS2_PLACEMENT_3D('',#275873,#142092,#142093);
#111514=AXIS2_PLACEMENT_3D('',#275875,#142094,#142095);
#111515=AXIS2_PLACEMENT_3D('',#275877,#142096,#142097);
#111516=AXIS2_PLACEMENT_3D('',#275879,#142099,#142100);
#111517=AXIS2_PLACEMENT_3D('',#275885,#142104,#142105);
#111518=AXIS2_PLACEMENT_3D('',#275891,#142109,#142110);
#111519=AXIS2_PLACEMENT_3D('',#275897,#142114,#142115);
#111520=AXIS2_PLACEMENT_3D('',#275903,#142119,#142120);
#111521=AXIS2_PLACEMENT_3D('',#275905,#142121,#142122);
#111522=AXIS2_PLACEMENT_3D('',#275907,#142123,#142124);
#111523=AXIS2_PLACEMENT_3D('',#275909,#142126,#142127);
#111524=AXIS2_PLACEMENT_3D('',#275915,#142131,#142132);
#111525=AXIS2_PLACEMENT_3D('',#275917,#142133,#142134);
#111526=AXIS2_PLACEMENT_3D('',#275919,#142135,#142136);
#111527=AXIS2_PLACEMENT_3D('',#275921,#142138,#142139);
#111528=AXIS2_PLACEMENT_3D('',#275927,#142143,#142144);
#111529=AXIS2_PLACEMENT_3D('',#275929,#142145,#142146);
#111530=AXIS2_PLACEMENT_3D('',#275931,#142147,#142148);
#111531=AXIS2_PLACEMENT_3D('',#275933,#142150,#142151);
#111532=AXIS2_PLACEMENT_3D('',#275939,#142155,#142156);
#111533=AXIS2_PLACEMENT_3D('',#275941,#142157,#142158);
#111534=AXIS2_PLACEMENT_3D('',#275943,#142159,#142160);
#111535=AXIS2_PLACEMENT_3D('',#275945,#142162,#142163);
#111536=AXIS2_PLACEMENT_3D('',#275951,#142167,#142168);
#111537=AXIS2_PLACEMENT_3D('',#275957,#142172,#142173);
#111538=AXIS2_PLACEMENT_3D('',#275963,#142177,#142178);
#111539=AXIS2_PLACEMENT_3D('',#275969,#142182,#142183);
#111540=AXIS2_PLACEMENT_3D('',#275971,#142184,#142185);
#111541=AXIS2_PLACEMENT_3D('',#275973,#142186,#142187);
#111542=AXIS2_PLACEMENT_3D('',#275975,#142189,#142190);
#111543=AXIS2_PLACEMENT_3D('',#275981,#142194,#142195);
#111544=AXIS2_PLACEMENT_3D('',#275987,#142199,#142200);
#111545=AXIS2_PLACEMENT_3D('',#275993,#142204,#142205);
#111546=AXIS2_PLACEMENT_3D('',#275999,#142209,#142210);
#111547=AXIS2_PLACEMENT_3D('',#276001,#142211,#142212);
#111548=AXIS2_PLACEMENT_3D('',#276003,#142213,#142214);
#111549=AXIS2_PLACEMENT_3D('',#276005,#142216,#142217);
#111550=AXIS2_PLACEMENT_3D('',#276011,#142221,#142222);
#111551=AXIS2_PLACEMENT_3D('',#276013,#142223,#142224);
#111552=AXIS2_PLACEMENT_3D('',#276015,#142225,#142226);
#111553=AXIS2_PLACEMENT_3D('',#276017,#142228,#142229);
#111554=AXIS2_PLACEMENT_3D('',#276023,#142233,#142234);
#111555=AXIS2_PLACEMENT_3D('',#276025,#142235,#142236);
#111556=AXIS2_PLACEMENT_3D('',#276027,#142237,#142238);
#111557=AXIS2_PLACEMENT_3D('',#276029,#142240,#142241);
#111558=AXIS2_PLACEMENT_3D('',#276035,#142245,#142246);
#111559=AXIS2_PLACEMENT_3D('',#276037,#142247,#142248);
#111560=AXIS2_PLACEMENT_3D('',#276039,#142249,#142250);
#111561=AXIS2_PLACEMENT_3D('',#276041,#142252,#142253);
#111562=AXIS2_PLACEMENT_3D('',#276044,#142256,#142257);
#111563=AXIS2_PLACEMENT_3D('',#276053,#142262,#142263);
#111564=AXIS2_PLACEMENT_3D('',#276059,#142267,#142268);
#111565=AXIS2_PLACEMENT_3D('',#276065,#142272,#142273);
#111566=AXIS2_PLACEMENT_3D('',#276067,#142274,#142275);
#111567=AXIS2_PLACEMENT_3D('',#276069,#142276,#142277);
#111568=AXIS2_PLACEMENT_3D('',#276071,#142279,#142280);
#111569=AXIS2_PLACEMENT_3D('',#276077,#142284,#142285);
#111570=AXIS2_PLACEMENT_3D('',#276079,#142286,#142287);
#111571=AXIS2_PLACEMENT_3D('',#276081,#142288,#142289);
#111572=AXIS2_PLACEMENT_3D('',#276083,#142291,#142292);
#111573=AXIS2_PLACEMENT_3D('',#276089,#142296,#142297);
#111574=AXIS2_PLACEMENT_3D('',#276091,#142298,#142299);
#111575=AXIS2_PLACEMENT_3D('',#276093,#142300,#142301);
#111576=AXIS2_PLACEMENT_3D('',#276095,#142303,#142304);
#111577=AXIS2_PLACEMENT_3D('',#276101,#142308,#142309);
#111578=AXIS2_PLACEMENT_3D('',#276103,#142310,#142311);
#111579=AXIS2_PLACEMENT_3D('',#276105,#142312,#142313);
#111580=AXIS2_PLACEMENT_3D('',#276107,#142315,#142316);
#111581=AXIS2_PLACEMENT_3D('',#276113,#142320,#142321);
#111582=AXIS2_PLACEMENT_3D('',#276119,#142325,#142326);
#111583=AXIS2_PLACEMENT_3D('',#276122,#142329,#142330);
#111584=AXIS2_PLACEMENT_3D('',#276128,#142334,#142335);
#111585=AXIS2_PLACEMENT_3D('',#276134,#142339,#142340);
#111586=AXIS2_PLACEMENT_3D('',#276140,#142344,#142345);
#111587=AXIS2_PLACEMENT_3D('',#276142,#142346,#142347);
#111588=AXIS2_PLACEMENT_3D('',#276144,#142348,#142349);
#111589=AXIS2_PLACEMENT_3D('',#276146,#142351,#142352);
#111590=AXIS2_PLACEMENT_3D('',#276152,#142356,#142357);
#111591=AXIS2_PLACEMENT_3D('',#276154,#142358,#142359);
#111592=AXIS2_PLACEMENT_3D('',#276156,#142360,#142361);
#111593=AXIS2_PLACEMENT_3D('',#276158,#142363,#142364);
#111594=AXIS2_PLACEMENT_3D('',#276164,#142368,#142369);
#111595=AXIS2_PLACEMENT_3D('',#276166,#142370,#142371);
#111596=AXIS2_PLACEMENT_3D('',#276168,#142372,#142373);
#111597=AXIS2_PLACEMENT_3D('',#276170,#142375,#142376);
#111598=AXIS2_PLACEMENT_3D('',#276176,#142380,#142381);
#111599=AXIS2_PLACEMENT_3D('',#276178,#142382,#142383);
#111600=AXIS2_PLACEMENT_3D('',#276180,#142384,#142385);
#111601=AXIS2_PLACEMENT_3D('',#276182,#142387,#142388);
#111602=AXIS2_PLACEMENT_3D('',#276188,#142392,#142393);
#111603=AXIS2_PLACEMENT_3D('',#276194,#142397,#142398);
#111604=AXIS2_PLACEMENT_3D('',#276200,#142402,#142403);
#111605=AXIS2_PLACEMENT_3D('',#276206,#142407,#142408);
#111606=AXIS2_PLACEMENT_3D('',#276208,#142409,#142410);
#111607=AXIS2_PLACEMENT_3D('',#276210,#142411,#142412);
#111608=AXIS2_PLACEMENT_3D('',#276212,#142414,#142415);
#111609=AXIS2_PLACEMENT_3D('',#276218,#142419,#142420);
#111610=AXIS2_PLACEMENT_3D('',#276220,#142421,#142422);
#111611=AXIS2_PLACEMENT_3D('',#276222,#142423,#142424);
#111612=AXIS2_PLACEMENT_3D('',#276224,#142426,#142427);
#111613=AXIS2_PLACEMENT_3D('',#276230,#142431,#142432);
#111614=AXIS2_PLACEMENT_3D('',#276232,#142433,#142434);
#111615=AXIS2_PLACEMENT_3D('',#276234,#142435,#142436);
#111616=AXIS2_PLACEMENT_3D('',#276236,#142438,#142439);
#111617=AXIS2_PLACEMENT_3D('',#276242,#142443,#142444);
#111618=AXIS2_PLACEMENT_3D('',#276244,#142445,#142446);
#111619=AXIS2_PLACEMENT_3D('',#276246,#142447,#142448);
#111620=AXIS2_PLACEMENT_3D('',#276248,#142450,#142451);
#111621=AXIS2_PLACEMENT_3D('',#276254,#142455,#142456);
#111622=AXIS2_PLACEMENT_3D('',#276260,#142460,#142461);
#111623=AXIS2_PLACEMENT_3D('',#276266,#142465,#142466);
#111624=AXIS2_PLACEMENT_3D('',#276272,#142470,#142471);
#111625=AXIS2_PLACEMENT_3D('',#276274,#142472,#142473);
#111626=AXIS2_PLACEMENT_3D('',#276276,#142474,#142475);
#111627=AXIS2_PLACEMENT_3D('',#276278,#142477,#142478);
#111628=AXIS2_PLACEMENT_3D('',#276284,#142482,#142483);
#111629=AXIS2_PLACEMENT_3D('',#276290,#142487,#142488);
#111630=AXIS2_PLACEMENT_3D('',#276296,#142492,#142493);
#111631=AXIS2_PLACEMENT_3D('',#276302,#142497,#142498);
#111632=AXIS2_PLACEMENT_3D('',#276304,#142499,#142500);
#111633=AXIS2_PLACEMENT_3D('',#276306,#142501,#142502);
#111634=AXIS2_PLACEMENT_3D('',#276308,#142504,#142505);
#111635=AXIS2_PLACEMENT_3D('',#276314,#142509,#142510);
#111636=AXIS2_PLACEMENT_3D('',#276316,#142511,#142512);
#111637=AXIS2_PLACEMENT_3D('',#276318,#142513,#142514);
#111638=AXIS2_PLACEMENT_3D('',#276320,#142516,#142517);
#111639=AXIS2_PLACEMENT_3D('',#276326,#142521,#142522);
#111640=AXIS2_PLACEMENT_3D('',#276328,#142523,#142524);
#111641=AXIS2_PLACEMENT_3D('',#276330,#142525,#142526);
#111642=AXIS2_PLACEMENT_3D('',#276332,#142528,#142529);
#111643=AXIS2_PLACEMENT_3D('',#276338,#142533,#142534);
#111644=AXIS2_PLACEMENT_3D('',#276340,#142535,#142536);
#111645=AXIS2_PLACEMENT_3D('',#276342,#142537,#142538);
#111646=AXIS2_PLACEMENT_3D('',#276344,#142540,#142541);
#111647=AXIS2_PLACEMENT_3D('',#276347,#142544,#142545);
#111648=AXIS2_PLACEMENT_3D('',#276353,#142549,#142550);
#111649=AXIS2_PLACEMENT_3D('',#276356,#142553,#142554);
#111650=AXIS2_PLACEMENT_3D('',#276362,#142558,#142559);
#111651=AXIS2_PLACEMENT_3D('',#276365,#142562,#142563);
#111652=AXIS2_PLACEMENT_3D('',#276382,#142572,#142573);
#111653=AXIS2_PLACEMENT_3D('',#276388,#142577,#142578);
#111654=AXIS2_PLACEMENT_3D('',#276392,#142581,#142582);
#111655=AXIS2_PLACEMENT_3D('',#276396,#142585,#142586);
#111656=AXIS2_PLACEMENT_3D('',#276400,#142589,#142590);
#111657=AXIS2_PLACEMENT_3D('',#276404,#142593,#142594);
#111658=AXIS2_PLACEMENT_3D('',#276408,#142597,#142598);
#111659=AXIS2_PLACEMENT_3D('',#276412,#142601,#142602);
#111660=AXIS2_PLACEMENT_3D('',#276414,#142604,#142605);
#111661=AXIS2_PLACEMENT_3D('',#276415,#142606,#142607);
#111662=AXIS2_PLACEMENT_3D('',#276424,#142612,#142613);
#111663=AXIS2_PLACEMENT_3D('',#276430,#142617,#142618);
#111664=AXIS2_PLACEMENT_3D('',#276436,#142622,#142623);
#111665=AXIS2_PLACEMENT_3D('',#276439,#142626,#142627);
#111666=AXIS2_PLACEMENT_3D('',#276440,#142628,#142629);
#140414=DIRECTION('axis',(0.,0.,1.));
#140415=DIRECTION('refdir',(1.,0.,0.));
#140416=DIRECTION('center_axis',(1.83697019872103E-16,1.83697019872101E-16,
-1.));
#140417=DIRECTION('ref_axis',(-1.,3.37445951098914E-32,-1.83697019872103E-16));
#140418=DIRECTION('center_axis',(0.,0.,1.));
#140419=DIRECTION('ref_axis',(1.,0.,0.));
#140420=DIRECTION('',(1.83697019872103E-16,1.83697019872101E-16,-1.));
#140421=DIRECTION('center_axis',(-1.83697019872103E-16,-1.83697019872101E-16,
1.));
#140422=DIRECTION('ref_axis',(1.04634114423998E-14,1.,1.83697019872103E-16));
#140423=DIRECTION('',(1.83697019872103E-16,1.83697019872101E-16,-1.));
#140424=DIRECTION('center_axis',(0.,0.,-1.));
#140425=DIRECTION('ref_axis',(-1.,0.,0.));
#140426=DIRECTION('center_axis',(-1.83697019872103E-16,-1.83697019872101E-16,
1.));
#140427=DIRECTION('ref_axis',(1.04905870583987E-14,1.,1.83697019872103E-16));
#140428=DIRECTION('',(0.767165151815313,0.641449631569141,2.58758337855511E-16));
#140429=DIRECTION('center_axis',(-1.83697019872103E-16,-1.83697019872101E-16,
1.));
#140430=DIRECTION('ref_axis',(-1.04634114423998E-14,-1.,-1.83697019872103E-16));
#140431=DIRECTION('',(0.7671651518153,-0.641449631569158,2.30935664208886E-17));
#140432=DIRECTION('center_axis',(-1.83697019872103E-16,-1.83697019872101E-16,
1.));
#140433=DIRECTION('ref_axis',(-1.04905870583987E-14,-1.,-1.83697019872103E-16));
#140434=DIRECTION('',(-0.641449631569148,0.767165151815307,2.30935664208889E-17));
#140435=DIRECTION('center_axis',(-1.83697019872103E-16,-1.83697019872101E-16,
1.));
#140436=DIRECTION('ref_axis',(-1.04634114423998E-14,-1.,-1.83697019872103E-16));
#140437=DIRECTION('',(0.641449631569153,0.767165151815304,2.58758337855511E-16));
#140438=DIRECTION('center_axis',(-1.83697019872103E-16,-1.83697019872101E-16,
1.));
#140439=DIRECTION('ref_axis',(-1.04905870583987E-14,-1.,-1.83697019872103E-16));
#140440=DIRECTION('',(-0.767165151815303,-0.641449631569154,-2.58758337855511E-16));
#140441=DIRECTION('center_axis',(-1.83697019872103E-16,-1.83697019872101E-16,
1.));
#140442=DIRECTION('ref_axis',(-1.04634114423998E-14,-1.,-1.83697019872103E-16));
#140443=DIRECTION('',(-0.767165151815289,0.64144963156917,-2.30935664208844E-17));
#140444=DIRECTION('center_axis',(-1.83697019872103E-16,-1.83697019872101E-16,
1.));
#140445=DIRECTION('ref_axis',(1.04905870583987E-14,1.,1.83697019872103E-16));
#140446=DIRECTION('',(0.641449631569137,-0.767165151815317,-2.3093566420893E-17));
#140447=DIRECTION('',(-0.641449631569165,-0.767165151815294,-2.58758337855512E-16));
#140448=DIRECTION('center_axis',(0.767165151815294,-0.641449631569165,2.30935664208862E-17));
#140449=DIRECTION('ref_axis',(0.641449631569165,0.767165151815294,6.40920668176173E-34));
#140450=DIRECTION('',(-0.641449631569165,-0.767165151815294,0.));
#140451=DIRECTION('',(1.83697019872103E-16,1.83697019872101E-16,-1.));
#140452=DIRECTION('center_axis',(0.767165151815317,0.641449631569137,2.58758337855511E-16));
#140453=DIRECTION('ref_axis',(-0.641449631569137,0.767165151815317,1.60642344084382E-32));
#140454=DIRECTION('',(1.83697019872103E-16,1.83697019872101E-16,-1.));
#140455=DIRECTION('',(0.641449631569137,-0.767165151815317,0.));
#140456=DIRECTION('center_axis',(1.83697019872103E-16,1.83697019872101E-16,
-1.));
#140457=DIRECTION('ref_axis',(-1.,3.37445951098915E-32,-1.83697019872103E-16));
#140458=DIRECTION('',(1.83697019872103E-16,1.83697019872101E-16,-1.));
#140459=DIRECTION('center_axis',(0.,0.,1.));
#140460=DIRECTION('ref_axis',(1.,0.,0.));
#140461=DIRECTION('center_axis',(-0.64144963156917,-0.76716515181529,-2.58758337855512E-16));
#140462=DIRECTION('ref_axis',(0.76716515181529,-0.64144963156917,1.85826510350639E-32));
#140463=DIRECTION('',(1.83697019872103E-16,1.83697019872101E-16,-1.));
#140464=DIRECTION('',(-0.767165151815289,0.64144963156917,0.));
#140465=DIRECTION('center_axis',(1.83697019872103E-16,1.83697019872101E-16,
-1.));
#140466=DIRECTION('ref_axis',(-1.,3.37445951098914E-32,-1.83697019872103E-16));
#140467=DIRECTION('',(1.83697019872103E-16,1.83697019872101E-16,-1.));
#140468=DIRECTION('center_axis',(0.,0.,1.));
#140469=DIRECTION('ref_axis',(1.,0.,0.));
#140470=DIRECTION('center_axis',(0.641449631569154,-0.767165151815303,-2.30935664208871E-17));
#140471=DIRECTION('ref_axis',(0.767165151815303,0.641449631569154,7.36235815021269E-34));
#140472=DIRECTION('',(1.83697019872103E-16,1.83697019872101E-16,-1.));
#140473=DIRECTION('',(-0.767165151815303,-0.641449631569154,0.));
#140474=DIRECTION('center_axis',(1.83697019872103E-16,1.83697019872101E-16,
-1.));
#140475=DIRECTION('ref_axis',(-1.,3.37445951098915E-32,-1.83697019872103E-16));
#140476=DIRECTION('',(1.83697019872103E-16,1.83697019872101E-16,-1.));
#140477=DIRECTION('center_axis',(0.,0.,1.));
#140478=DIRECTION('ref_axis',(1.,0.,0.));
#140479=DIRECTION('center_axis',(-0.767165151815304,0.641449631569153,-2.30935664208902E-17));
#140480=DIRECTION('ref_axis',(-0.641449631569153,-0.767165151815304,1.00176035722907E-34));
#140481=DIRECTION('',(1.83697019872103E-16,1.83697019872101E-16,-1.));
#140482=DIRECTION('',(0.641449631569153,0.767165151815304,0.));
#140483=DIRECTION('center_axis',(1.83697019872103E-16,1.83697019872101E-16,
-1.));
#140484=DIRECTION('ref_axis',(1.,-1.22464679914735E-16,1.83697019872103E-16));
#140485=DIRECTION('',(1.83697019872103E-16,1.83697019872101E-16,-1.));
#140486=DIRECTION('center_axis',(0.,0.,1.));
#140487=DIRECTION('ref_axis',(1.,0.,0.));
#140488=DIRECTION('center_axis',(-0.767165151815307,-0.641449631569149,
-2.58758337855511E-16));
#140489=DIRECTION('ref_axis',(0.641449631569149,-0.767165151815307,1.72189280676572E-33));
#140490=DIRECTION('',(1.83697019872103E-16,1.83697019872101E-16,-1.));
#140491=DIRECTION('',(-0.641449631569149,0.767165151815307,0.));
#140492=DIRECTION('center_axis',(1.83697019872103E-16,1.83697019872101E-16,
-1.));
#140493=DIRECTION('ref_axis',(-1.,3.37445951098915E-32,-1.83697019872103E-16));
#140494=DIRECTION('',(1.83697019872103E-16,1.83697019872101E-16,-1.));
#140495=DIRECTION('center_axis',(0.,0.,1.));
#140496=DIRECTION('ref_axis',(1.,0.,0.));
#140497=DIRECTION('center_axis',(0.641449631569158,0.7671651518153,2.58758337855511E-16));
#140498=DIRECTION('ref_axis',(-0.7671651518153,0.641449631569158,3.71248381684349E-33));
#140499=DIRECTION('',(1.83697019872103E-16,1.83697019872101E-16,-1.));
#140500=DIRECTION('',(0.7671651518153,-0.641449631569157,0.));
#140501=DIRECTION('center_axis',(1.83697019872103E-16,1.83697019872101E-16,
-1.));
#140502=DIRECTION('ref_axis',(-1.,3.37445951098914E-32,-1.83697019872103E-16));
#140503=DIRECTION('',(1.83697019872103E-16,1.83697019872101E-16,-1.));
#140504=DIRECTION('center_axis',(0.,0.,1.));
#140505=DIRECTION('ref_axis',(1.,0.,0.));
#140506=DIRECTION('center_axis',(-0.641449631569142,0.767165151815313,2.30935664208913E-17));
#140507=DIRECTION('ref_axis',(-0.767165151815313,-0.641449631569142,-1.08468999085769E-33));
#140508=DIRECTION('',(1.83697019872103E-16,1.83697019872101E-16,-1.));
#140509=DIRECTION('',(0.767165151815313,0.641449631569142,0.));
#140510=DIRECTION('center_axis',(1.83697019872103E-16,1.83697019872101E-16,
-1.));
#140511=DIRECTION('ref_axis',(-1.,3.37445951098914E-32,-1.83697019872103E-16));
#140512=DIRECTION('center_axis',(0.,0.,1.));
#140513=DIRECTION('ref_axis',(1.,0.,0.));
#140514=DIRECTION('center_axis',(0.,0.,1.));
#140515=DIRECTION('ref_axis',(1.,0.,0.));
#140516=DIRECTION('center_axis',(0.,0.,-1.));
#140517=DIRECTION('ref_axis',(-1.,0.,0.));
#140518=DIRECTION('center_axis',(-1.83697019872103E-16,-1.83697019872101E-16,
1.));
#140519=DIRECTION('ref_axis',(1.15648231731787E-14,1.,1.83697019872103E-16));
#140520=DIRECTION('',(1.04744440165294E-14,1.,1.83697019872103E-16));
#140521=DIRECTION('center_axis',(-1.83697019872103E-16,-1.83697019872101E-16,
1.));
#140522=DIRECTION('ref_axis',(1.15648231731787E-14,1.,1.83697019872103E-16));
#140523=DIRECTION('',(-1.,1.04744440165294E-14,-1.83697019872101E-16));
#140524=DIRECTION('center_axis',(-1.83697019872103E-16,-1.83697019872101E-16,
1.));
#140525=DIRECTION('ref_axis',(1.15648231731787E-14,1.,1.83697019872103E-16));
#140526=DIRECTION('',(-8.90384784090525E-15,-1.,-1.83697019872103E-16));
#140527=DIRECTION('center_axis',(-1.83697019872103E-16,-1.83697019872101E-16,
1.));
#140528=DIRECTION('ref_axis',(1.15648231731787E-14,1.,1.83697019872103E-16));
#140529=DIRECTION('',(1.,-1.04744440165294E-14,1.83697019872101E-16));
#140530=DIRECTION('center_axis',(1.04744440165294E-14,1.,1.83697019872103E-16));
#140531=DIRECTION('ref_axis',(-1.,1.04744440165294E-14,0.));
#140532=DIRECTION('',(1.83697019872103E-16,1.83697019872101E-16,-1.));
#140533=DIRECTION('',(1.,-1.04744440165294E-14,0.));
#140534=DIRECTION('',(1.83697019872103E-16,1.83697019872101E-16,-1.));
#140535=DIRECTION('center_axis',(1.83697019872103E-16,1.83697019872101E-16,
-1.));
#140536=DIRECTION('ref_axis',(-1.,3.37445951098915E-32,-1.83697019872103E-16));
#140537=DIRECTION('',(1.83697019872103E-16,1.83697019872101E-16,-1.));
#140538=DIRECTION('center_axis',(0.,0.,1.));
#140539=DIRECTION('ref_axis',(1.,0.,0.));
#140540=DIRECTION('center_axis',(1.,-8.90384784090525E-15,1.83697019872101E-16));
#140541=DIRECTION('ref_axis',(8.90384784090525E-15,1.,1.26229010772883E-47));
#140542=DIRECTION('',(1.83697019872103E-16,1.83697019872101E-16,-1.));
#140543=DIRECTION('',(-8.90384784090525E-15,-1.,0.));
#140544=DIRECTION('center_axis',(1.83697019872103E-16,1.83697019872101E-16,
-1.));
#140545=DIRECTION('ref_axis',(-1.,3.37445951098915E-32,-1.83697019872103E-16));
#140546=DIRECTION('',(1.83697019872103E-16,1.83697019872101E-16,-1.));
#140547=DIRECTION('center_axis',(0.,0.,1.));
#140548=DIRECTION('ref_axis',(1.,0.,0.));
#140549=DIRECTION('center_axis',(-1.04744440165294E-14,-1.,-1.83697019872103E-16));
#140550=DIRECTION('ref_axis',(1.,-1.04744440165294E-14,0.));
#140551=DIRECTION('',(1.83697019872103E-16,1.83697019872101E-16,-1.));
#140552=DIRECTION('',(-1.,1.04744440165294E-14,0.));
#140553=DIRECTION('center_axis',(1.83697019872103E-16,1.83697019872101E-16,
-1.));
#140554=DIRECTION('ref_axis',(-1.,3.37445951098915E-32,-1.83697019872103E-16));
#140555=DIRECTION('',(1.83697019872103E-16,1.83697019872101E-16,-1.));
#140556=DIRECTION('center_axis',(0.,0.,1.));
#140557=DIRECTION('ref_axis',(1.,0.,0.));
#140558=DIRECTION('center_axis',(-1.,1.04744440165294E-14,-1.83697019872101E-16));
#140559=DIRECTION('ref_axis',(-1.04744440165294E-14,-1.,-1.01856090860782E-46));
#140560=DIRECTION('',(1.83697019872103E-16,1.83697019872101E-16,-1.));
#140561=DIRECTION('',(1.04744440165294E-14,1.,0.));
#140562=DIRECTION('center_axis',(1.83697019872103E-16,1.83697019872101E-16,
-1.));
#140563=DIRECTION('ref_axis',(-1.,3.37445951098915E-32,-1.83697019872103E-16));
#140564=DIRECTION('center_axis',(0.,0.,1.));
#140565=DIRECTION('ref_axis',(1.,0.,0.));
#140566=DIRECTION('center_axis',(0.,0.,1.));
#140567=DIRECTION('ref_axis',(1.,0.,0.));
#140568=DIRECTION('center_axis',(0.,0.,1.));
#140569=DIRECTION('ref_axis',(1.,0.,0.));
#140570=DIRECTION('center_axis',(0.,0.,-1.));
#140571=DIRECTION('ref_axis',(1.,0.,0.));
#140572=DIRECTION('',(1.28023872765816E-15,1.,0.));
#140573=DIRECTION('center_axis',(0.,0.,-1.));
#140574=DIRECTION('ref_axis',(1.,0.,0.));
#140575=DIRECTION('',(1.,0.,0.));
#140576=DIRECTION('center_axis',(0.,0.,1.));
#140577=DIRECTION('ref_axis',(1.,0.,0.));
#140578=DIRECTION('',(0.707106781186549,0.707106781186546,0.));
#140579=DIRECTION('center_axis',(0.,0.,-1.));
#140580=DIRECTION('ref_axis',(1.,-5.13992141030166E-15,0.));
#140581=DIRECTION('',(1.,5.01365166467286E-16,0.));
#140582=DIRECTION('',(0.707106781186547,0.707106781186547,0.));
#140583=DIRECTION('',(7.80891617653129E-15,1.,0.));
#140584=DIRECTION('center_axis',(0.,0.,-1.));
#140585=DIRECTION('ref_axis',(1.,5.13992141030166E-15,0.));
#140586=DIRECTION('',(0.707106781186551,0.707106781186544,0.));
#140587=DIRECTION('center_axis',(0.,0.,1.));
#140588=DIRECTION('ref_axis',(1.,0.,0.));
#140589=DIRECTION('',(7.66554070360109E-15,1.,0.));
#140590=DIRECTION('center_axis',(0.,0.,-1.));
#140591=DIRECTION('ref_axis',(1.,0.,0.));
#140592=DIRECTION('',(1.,-5.12095491063264E-15,0.));
#140593=DIRECTION('center_axis',(0.,0.,-1.));
#140594=DIRECTION('ref_axis',(1.,1.54197642309049E-14,0.));
#140595=DIRECTION('',(-3.49148133884313E-15,-1.,0.));
#140596=DIRECTION('center_axis',(0.,0.,1.));
#140597=DIRECTION('ref_axis',(1.,0.,0.));
#140598=DIRECTION('',(0.707106781186544,-0.707106781186551,0.));
#140599=DIRECTION('center_axis',(0.,0.,-1.));
#140600=DIRECTION('ref_axis',(1.,-2.56996070515083E-15,0.));
#140601=DIRECTION('',(-2.99011617237585E-15,-1.,0.));
#140602=DIRECTION('',(0.707106781186545,-0.70710678118655,0.));
#140603=DIRECTION('',(1.,-1.13003975153744E-14,0.));
#140604=DIRECTION('center_axis',(0.,0.,-1.));
#140605=DIRECTION('ref_axis',(1.,3.85494105772625E-15,0.));
#140606=DIRECTION('',(0.707106781186541,-0.707106781186554,0.));
#140607=DIRECTION('center_axis',(0.,0.,1.));
#140608=DIRECTION('ref_axis',(1.,0.,0.));
#140609=DIRECTION('',(1.,-1.11570220424442E-14,0.));
#140610=DIRECTION('center_axis',(0.,0.,-1.));
#140611=DIRECTION('ref_axis',(1.,3.91919007535501E-14,0.));
#140612=DIRECTION('',(-8.61243624947577E-15,-1.,0.));
#140613=DIRECTION('center_axis',(0.,0.,-1.));
#140614=DIRECTION('ref_axis',(1.,0.,0.));
#140615=DIRECTION('',(-1.,0.,0.));
#140616=DIRECTION('center_axis',(0.,0.,1.));
#140617=DIRECTION('ref_axis',(1.,0.,0.));
#140618=DIRECTION('',(-0.707106781186549,-0.707106781186546,0.));
#140619=DIRECTION('center_axis',(0.,0.,-1.));
#140620=DIRECTION('ref_axis',(1.,6.42490176287708E-16,0.));
#140621=DIRECTION('',(-1.,-5.01365166467286E-16,0.));
#140622=DIRECTION('',(-0.707106781186547,-0.707106781186547,0.));
#140623=DIRECTION('',(-7.80891617653129E-15,-1.,0.));
#140624=DIRECTION('center_axis',(0.,0.,-1.));
#140625=DIRECTION('ref_axis',(1.,-1.02798428206033E-14,0.));
#140626=DIRECTION('',(-0.707106781186551,-0.707106781186544,0.));
#140627=DIRECTION('center_axis',(0.,0.,1.));
#140628=DIRECTION('ref_axis',(1.,0.,0.));
#140629=DIRECTION('',(-7.66554070360109E-15,-1.,0.));
#140630=DIRECTION('center_axis',(0.,0.,-1.));
#140631=DIRECTION('ref_axis',(1.,-7.70988211545247E-15,0.));
#140632=DIRECTION('',(-1.,5.12095491063264E-15,0.));
#140633=DIRECTION('center_axis',(0.,0.,-1.));
#140634=DIRECTION('ref_axis',(1.,0.,0.));
#140635=DIRECTION('',(1.04744440165294E-14,1.,0.));
#140636=DIRECTION('center_axis',(0.,0.,1.));
#140637=DIRECTION('ref_axis',(1.,0.,0.));
#140638=DIRECTION('',(-0.707106781186539,0.707106781186556,0.));
#140639=DIRECTION('center_axis',(0.,0.,-1.));
#140640=DIRECTION('ref_axis',(1.,2.56996070515083E-15,0.));
#140641=DIRECTION('',(9.97307885006211E-15,1.,0.));
#140642=DIRECTION('',(-0.70710678118654,0.707106781186555,0.));
#140643=DIRECTION('',(-1.,1.82833601930607E-14,0.));
#140644=DIRECTION('center_axis',(0.,0.,-1.));
#140645=DIRECTION('ref_axis',(1.,6.42490176287708E-16,0.));
#140646=DIRECTION('',(-0.707106781186536,0.707106781186559,0.));
#140647=DIRECTION('center_axis',(0.,0.,1.));
#140648=DIRECTION('ref_axis',(1.,0.,0.));
#140649=DIRECTION('',(-1.,1.81399847201305E-14,0.));
#140650=DIRECTION('center_axis',(0.,0.,-1.));
#140651=DIRECTION('ref_axis',(-1.,0.,0.));
#140652=DIRECTION('center_axis',(0.,0.,-1.));
#140653=DIRECTION('ref_axis',(-1.,0.,0.));
#140654=DIRECTION('',(1.28023872765816E-15,1.,0.));
#140655=DIRECTION('center_axis',(1.83697019872103E-16,1.83697019872101E-16,
-1.));
#140656=DIRECTION('ref_axis',(1.02798428206033E-14,1.,1.83697019872103E-16));
#140657=DIRECTION('',(-1.,1.81399847201305E-14,-1.836970198721E-16));
#140658=DIRECTION('center_axis',(-1.83697019872103E-16,-1.83697019872101E-16,
1.));
#140659=DIRECTION('ref_axis',(-1.02798428206033E-14,-1.,-1.83697019872103E-16));
#140660=DIRECTION('',(-0.707106781186536,0.707106781186559,2.81031697484985E-30));
#140661=DIRECTION('center_axis',(1.83697019872103E-16,1.83697019872101E-16,
-1.));
#140662=DIRECTION('ref_axis',(1.02798428206033E-14,1.,1.83697019872103E-16));
#140663=DIRECTION('',(-1.,1.82833601930607E-14,-1.836970198721E-16));
#140664=DIRECTION('',(-0.70710678118654,0.707106781186555,1.35585468084861E-30));
#140665=DIRECTION('',(9.97307885006212E-15,1.,1.83697019872103E-16));
#140666=DIRECTION('center_axis',(1.83697019872103E-16,1.83697019872101E-16,
-1.));
#140667=DIRECTION('ref_axis',(-1.02798428206033E-14,-1.,-1.83697019872103E-16));
#140668=DIRECTION('',(-0.707106781186539,0.707106781186556,1.75028513345912E-30));
#140669=DIRECTION('center_axis',(-1.83697019872103E-16,-1.83697019872101E-16,
1.));
#140670=DIRECTION('ref_axis',(1.02798428206033E-14,1.,1.83697019872103E-16));
#140671=DIRECTION('',(1.04744440165294E-14,1.,1.83697019872103E-16));
#140672=DIRECTION('center_axis',(1.83697019872103E-16,1.83697019872101E-16,
-1.));
#140673=DIRECTION('ref_axis',(-1.06010879087472E-14,-1.,-1.83697019872103E-16));
#140674=DIRECTION('',(-1.,5.12095491063264E-15,1.88140831196526E-30));
#140675=DIRECTION('center_axis',(0.,3.67394039744206E-16,-1.));
#140676=DIRECTION('ref_axis',(-1.,0.,0.));
#140677=DIRECTION('',(-7.6655407036011E-15,-1.,-3.67394039744206E-16));
#140678=DIRECTION('center_axis',(0.,-3.67394039744206E-16,1.));
#140679=DIRECTION('ref_axis',(1.,0.,0.));
#140680=DIRECTION('',(-0.707106781186551,-0.707106781186544,-2.59786816870647E-16));
#140681=DIRECTION('center_axis',(0.,3.67394039744206E-16,-1.));
#140682=DIRECTION('ref_axis',(-1.,0.,0.));
#140683=DIRECTION('',(-7.80891617653129E-15,-1.,-3.67394039744206E-16));
#140684=DIRECTION('',(-0.707106781186547,-0.707106781186547,-2.59786816870648E-16));
#140685=DIRECTION('',(-1.,-5.01365166467286E-16,-1.84198573895442E-31));
#140686=DIRECTION('center_axis',(0.,3.67394039744206E-16,-1.));
#140687=DIRECTION('ref_axis',(1.,0.,0.));
#140688=DIRECTION('',(-0.707106781186549,-0.707106781186546,-2.59786816870648E-16));
#140689=DIRECTION('center_axis',(0.,-3.67394039744206E-16,1.));
#140690=DIRECTION('ref_axis',(-1.,0.,0.));
#140691=DIRECTION('',(-1.,0.,0.));
#140692=DIRECTION('center_axis',(0.,3.67394039744206E-16,-1.));
#140693=DIRECTION('ref_axis',(1.,0.,0.));
#140694=DIRECTION('',(-8.61243624947577E-15,-1.,-1.83697019872102E-16));
#140695=DIRECTION('center_axis',(-1.83697019872103E-16,1.83697019872104E-16,
-1.));
#140696=DIRECTION('ref_axis',(-2.56996070515082E-15,-1.,-1.83697019872103E-16));
#140697=DIRECTION('',(1.,-1.11570220424442E-14,-1.83697019872105E-16));
#140698=DIRECTION('center_axis',(1.83697019872103E-16,-1.83697019872104E-16,
1.));
#140699=DIRECTION('ref_axis',(2.56996070515083E-15,1.,1.83697019872103E-16));
#140700=DIRECTION('',(0.707106781186541,-0.707106781186554,-2.59786816870648E-16));
#140701=DIRECTION('center_axis',(-1.83697019872103E-16,1.83697019872104E-16,
-1.));
#140702=DIRECTION('ref_axis',(-2.56996070515083E-15,-1.,-1.83697019872103E-16));
#140703=DIRECTION('',(1.,-1.13003975153744E-14,-1.83697019872105E-16));
#140704=DIRECTION('',(0.707106781186545,-0.70710678118655,-2.59786816870648E-16));
#140705=DIRECTION('',(-2.99011617237585E-15,-1.,-1.83697019872103E-16));
#140706=DIRECTION('center_axis',(-1.83697019872103E-16,1.83697019872104E-16,
-1.));
#140707=DIRECTION('ref_axis',(3.21245088143854E-15,1.,1.83697019872103E-16));
#140708=DIRECTION('',(0.707106781186544,-0.707106781186551,-2.59786816870649E-16));
#140709=DIRECTION('center_axis',(1.83697019872103E-16,-1.83697019872104E-16,
1.));
#140710=DIRECTION('ref_axis',(-3.21245088143853E-15,-1.,-1.83697019872103E-16));
#140711=DIRECTION('',(-3.49148133884313E-15,-1.,-1.83697019872103E-16));
#140712=DIRECTION('center_axis',(-1.83697019872103E-16,1.83697019872104E-16,
-1.));
#140713=DIRECTION('ref_axis',(3.53369596958238E-15,1.,1.83697019872103E-16));
#140714=DIRECTION('',(1.,-5.12095491063264E-15,0.));
#140715=DIRECTION('center_axis',(0.,0.,-1.));
#140716=DIRECTION('ref_axis',(1.,0.,0.));
#140717=DIRECTION('',(7.6655407036011E-15,1.,0.));
#140718=DIRECTION('center_axis',(0.,0.,1.));
#140719=DIRECTION('ref_axis',(-1.,0.,0.));
#140720=DIRECTION('',(0.707106781186551,0.707106781186544,0.));
#140721=DIRECTION('center_axis',(0.,0.,-1.));
#140722=DIRECTION('ref_axis',(1.,0.,0.));
#140723=DIRECTION('',(7.80891617653129E-15,1.,0.));
#140724=DIRECTION('',(0.707106781186547,0.707106781186547,0.));
#140725=DIRECTION('',(1.,5.01365166467286E-16,0.));
#140726=DIRECTION('center_axis',(0.,0.,-1.));
#140727=DIRECTION('ref_axis',(-1.,0.,0.));
#140728=DIRECTION('',(0.707106781186549,0.707106781186546,0.));
#140729=DIRECTION('center_axis',(0.,0.,1.));
#140730=DIRECTION('ref_axis',(1.,0.,0.));
#140731=DIRECTION('',(1.,0.,0.));
#140732=DIRECTION('center_axis',(1.83697019872103E-16,1.83697019872101E-16,
-1.));
#140733=DIRECTION('ref_axis',(-1.,3.37445951098915E-32,-1.83697019872103E-16));
#140734=DIRECTION('',(1.83697019872103E-16,1.83697019872101E-16,-1.));
#140735=DIRECTION('',(1.83697019872103E-16,1.83697019872101E-16,-1.));
#140736=DIRECTION('center_axis',(-1.81399847201305E-14,-1.,-1.83697019872104E-16));
#140737=DIRECTION('ref_axis',(1.,-1.81399847201305E-14,0.));
#140738=DIRECTION('',(1.83697019872103E-16,1.83697019872101E-16,-1.));
#140739=DIRECTION('center_axis',(1.83697019872103E-16,1.83697019872101E-16,
-1.));
#140740=DIRECTION('ref_axis',(-1.,3.37445951098915E-32,-1.83697019872103E-16));
#140741=DIRECTION('',(1.83697019872103E-16,1.83697019872101E-16,-1.));
#140742=DIRECTION('center_axis',(-0.707106781186559,-0.707106781186536,
-2.59786816870647E-16));
#140743=DIRECTION('ref_axis',(0.707106781186536,-0.707106781186559,-8.51191961352541E-33));
#140744=DIRECTION('',(1.83697019872103E-16,1.83697019872101E-16,-1.));
#140745=DIRECTION('center_axis',(1.83697019872103E-16,1.83697019872101E-16,
-1.));
#140746=DIRECTION('ref_axis',(-1.,3.37445951098915E-32,-1.83697019872103E-16));
#140747=DIRECTION('',(1.83697019872103E-16,1.83697019872101E-16,-1.));
#140748=DIRECTION('center_axis',(-1.82833601930607E-14,-1.,-1.83697019872104E-16));
#140749=DIRECTION('ref_axis',(1.,-1.82833601930607E-14,0.));
#140750=DIRECTION('',(1.83697019872103E-16,1.83697019872101E-16,-1.));
#140751=DIRECTION('center_axis',(-0.707106781186555,-0.70710678118654,-2.59786816870647E-16));
#140752=DIRECTION('ref_axis',(0.70710678118654,-0.707106781186555,3.77583739123461E-33));
#140753=DIRECTION('',(1.83697019872103E-16,1.83697019872101E-16,-1.));
#140754=DIRECTION('center_axis',(-1.,9.97307885006211E-15,-1.83697019872101E-16));
#140755=DIRECTION('ref_axis',(-9.97307885006211E-15,-1.,7.95933057668596E-47));
#140756=DIRECTION('',(1.83697019872103E-16,1.83697019872101E-16,-1.));
#140757=DIRECTION('center_axis',(1.83697019872103E-16,1.83697019872101E-16,
-1.));
#140758=DIRECTION('ref_axis',(-1.,3.37445951098915E-32,-1.83697019872103E-16));
#140759=DIRECTION('',(1.83697019872103E-16,1.83697019872101E-16,-1.));
#140760=DIRECTION('center_axis',(-0.707106781186556,-0.707106781186539,
-2.59786816870647E-16));
#140761=DIRECTION('ref_axis',(0.707106781186539,-0.707106781186556,1.19724503022165E-32));
#140762=DIRECTION('',(1.83697019872103E-16,1.83697019872101E-16,-1.));
#140763=DIRECTION('center_axis',(1.83697019872103E-16,1.83697019872101E-16,
-1.));
#140764=DIRECTION('ref_axis',(-1.,3.37445951098914E-32,-1.83697019872103E-16));
#140765=DIRECTION('',(1.83697019872103E-16,1.83697019872101E-16,-1.));
#140766=DIRECTION('center_axis',(-1.,1.04744440165294E-14,-1.83697019872101E-16));
#140767=DIRECTION('ref_axis',(-1.04744440165294E-14,-1.,-1.01856090860782E-46));
#140768=DIRECTION('',(1.83697019872103E-16,1.83697019872101E-16,-1.));
#140769=DIRECTION('center_axis',(1.83697019872103E-16,1.83697019872101E-16,
-1.));
#140770=DIRECTION('ref_axis',(-1.,3.37445951098915E-32,-1.83697019872103E-16));
#140771=DIRECTION('',(1.83697019872103E-16,1.83697019872101E-16,-1.));
#140772=DIRECTION('center_axis',(-5.12095491063264E-15,-1.,-3.67394039744206E-16));
#140773=DIRECTION('ref_axis',(1.,-5.12095491063264E-15,0.));
#140774=DIRECTION('',(0.,3.67394039744206E-16,-1.));
#140775=DIRECTION('center_axis',(0.,3.67394039744206E-16,-1.));
#140776=DIRECTION('ref_axis',(0.,1.,3.67394039744206E-16));
#140777=DIRECTION('',(0.,3.67394039744206E-16,-1.));
#140778=DIRECTION('center_axis',(1.,-7.66554070360109E-15,-2.81627396591965E-30));
#140779=DIRECTION('ref_axis',(7.66554070360109E-15,1.,1.20244003954024E-60));
#140780=DIRECTION('',(0.,3.67394039744206E-16,-1.));
#140781=DIRECTION('center_axis',(0.,3.67394039744206E-16,-1.));
#140782=DIRECTION('ref_axis',(0.,1.,3.67394039744206E-16));
#140783=DIRECTION('',(0.,3.67394039744206E-16,-1.));
#140784=DIRECTION('center_axis',(0.707106781186544,-0.707106781186552,-2.59786816870649E-16));
#140785=DIRECTION('ref_axis',(0.707106781186552,0.707106781186544,1.54452889108689E-32));
#140786=DIRECTION('',(0.,3.67394039744206E-16,-1.));
#140787=DIRECTION('center_axis',(0.,3.67394039744206E-16,-1.));
#140788=DIRECTION('ref_axis',(0.,1.,3.67394039744206E-16));
#140789=DIRECTION('',(0.,3.67394039744206E-16,-1.));
#140790=DIRECTION('center_axis',(1.,-7.80891617653129E-15,-2.86894926011971E-30));
#140791=DIRECTION('ref_axis',(7.80891617653129E-15,1.,1.38445973011545E-61));
#140792=DIRECTION('',(0.,3.67394039744206E-16,-1.));
#140793=DIRECTION('center_axis',(0.707106781186548,-0.707106781186548,-2.59786816870648E-16));
#140794=DIRECTION('ref_axis',(0.707106781186548,0.707106781186548,-1.22182752772918E-34));
#140795=DIRECTION('',(0.,3.67394039744206E-16,-1.));
#140796=DIRECTION('center_axis',(5.01365166467286E-16,-1.,-3.67394039744206E-16));
#140797=DIRECTION('ref_axis',(1.,5.01365166467286E-16,0.));
#140798=DIRECTION('',(0.,3.67394039744206E-16,-1.));
#140799=DIRECTION('center_axis',(0.,3.67394039744206E-16,-1.));
#140800=DIRECTION('ref_axis',(0.,1.,3.67394039744206E-16));
#140801=DIRECTION('',(0.,3.67394039744206E-16,-1.));
#140802=DIRECTION('center_axis',(0.707106781186546,-0.707106781186549,-2.59786816870648E-16));
#140803=DIRECTION('ref_axis',(0.707106781186549,0.707106781186546,3.35953521571076E-33));
#140804=DIRECTION('',(0.,3.67394039744206E-16,-1.));
#140805=DIRECTION('center_axis',(0.,3.67394039744206E-16,-1.));
#140806=DIRECTION('ref_axis',(0.,1.,3.67394039744206E-16));
#140807=DIRECTION('',(0.,3.67394039744206E-16,-1.));
#140808=DIRECTION('center_axis',(0.,-1.,-3.67394039744206E-16));
#140809=DIRECTION('ref_axis',(0.,3.67394039744206E-16,-1.));
#140810=DIRECTION('',(0.,3.67394039744206E-16,-1.));
#140811=DIRECTION('center_axis',(0.,3.67394039744206E-16,-1.));
#140812=DIRECTION('ref_axis',(0.,1.,3.67394039744206E-16));
#140813=DIRECTION('',(0.,3.67394039744206E-16,-1.));
#140814=DIRECTION('center_axis',(1.,-8.61243624947577E-15,-1.83697019872105E-16));
#140815=DIRECTION('ref_axis',(8.61243624947577E-15,1.,7.69347343280275E-47));
#140816=DIRECTION('',(-1.83697019872103E-16,1.83697019872104E-16,-1.));
#140817=DIRECTION('center_axis',(-1.83697019872103E-16,1.83697019872104E-16,
-1.));
#140818=DIRECTION('ref_axis',(3.37445951098919E-32,1.,1.83697019872104E-16));
#140819=DIRECTION('',(-1.83697019872103E-16,1.83697019872104E-16,-1.));
#140820=DIRECTION('center_axis',(1.11570220424442E-14,1.,1.83697019872102E-16));
#140821=DIRECTION('ref_axis',(-1.,1.11570220424442E-14,0.));
#140822=DIRECTION('',(-1.83697019872103E-16,1.83697019872104E-16,-1.));
#140823=DIRECTION('center_axis',(-1.83697019872103E-16,1.83697019872104E-16,
-1.));
#140824=DIRECTION('ref_axis',(3.37445951098919E-32,1.,1.83697019872104E-16));
#140825=DIRECTION('',(-1.83697019872103E-16,1.83697019872104E-16,-1.));
#140826=DIRECTION('center_axis',(0.707106781186554,0.707106781186541,-1.89630025293512E-30));
#140827=DIRECTION('ref_axis',(-0.707106781186541,0.707106781186554,6.79668681715311E-48));
#140828=DIRECTION('',(-1.83697019872103E-16,1.83697019872104E-16,-1.));
#140829=DIRECTION('center_axis',(-1.83697019872103E-16,1.83697019872104E-16,
-1.));
#140830=DIRECTION('ref_axis',(3.37445951098919E-32,1.,1.83697019872104E-16));
#140831=DIRECTION('',(-1.83697019872103E-16,1.83697019872104E-16,-1.));
#140832=DIRECTION('center_axis',(1.13003975153744E-14,1.,1.83697019872102E-16));
#140833=DIRECTION('ref_axis',(-1.,1.13003975153744E-14,0.));
#140834=DIRECTION('',(-1.83697019872103E-16,1.83697019872104E-16,-1.));
#140835=DIRECTION('center_axis',(0.70710678118655,0.707106781186545,-4.36149058175078E-31));
#140836=DIRECTION('ref_axis',(-0.707106781186545,0.70710678118655,-2.09609619079153E-48));
#140837=DIRECTION('',(-1.83697019872103E-16,1.83697019872104E-16,-1.));
#140838=DIRECTION('center_axis',(1.,-2.99011617237585E-15,-1.83697019872104E-16));
#140839=DIRECTION('ref_axis',(2.99011617237585E-15,1.,-2.91458608578564E-48));
#140840=DIRECTION('',(-1.83697019872103E-16,1.83697019872104E-16,-1.));
#140841=DIRECTION('center_axis',(-1.83697019872103E-16,1.83697019872104E-16,
-1.));
#140842=DIRECTION('ref_axis',(3.37445951098919E-32,1.,1.83697019872104E-16));
#140843=DIRECTION('',(-1.83697019872103E-16,1.83697019872104E-16,-1.));
#140844=DIRECTION('center_axis',(0.707106781186551,0.707106781186544,-8.34372111291455E-31));
#140845=DIRECTION('ref_axis',(-0.707106781186544,0.707106781186551,-4.97404528384751E-47));
#140846=DIRECTION('',(-1.83697019872103E-16,1.83697019872104E-16,-1.));
#140847=DIRECTION('center_axis',(-1.83697019872103E-16,1.83697019872104E-16,
-1.));
#140848=DIRECTION('ref_axis',(3.37445951098919E-32,1.,1.83697019872104E-16));
#140849=DIRECTION('',(-1.83697019872103E-16,1.83697019872104E-16,-1.));
#140850=DIRECTION('center_axis',(1.,-3.49148133884313E-15,-1.83697019872104E-16));
#140851=DIRECTION('ref_axis',(3.49148133884313E-15,1.,-1.78914547131776E-47));
#140852=DIRECTION('',(-1.83697019872103E-16,1.83697019872104E-16,-1.));
#140853=DIRECTION('center_axis',(-1.83697019872103E-16,1.83697019872104E-16,
-1.));
#140854=DIRECTION('ref_axis',(3.37445951098919E-32,1.,1.83697019872104E-16));
#140855=DIRECTION('',(-1.83697019872103E-16,1.83697019872104E-16,-1.));
#140856=DIRECTION('center_axis',(5.12095491063264E-15,1.,0.));
#140857=DIRECTION('ref_axis',(-1.,5.12095491063264E-15,0.));
#140858=DIRECTION('',(0.,0.,-1.));
#140859=DIRECTION('center_axis',(0.,0.,-1.));
#140860=DIRECTION('ref_axis',(-1.,0.,0.));
#140861=DIRECTION('',(0.,0.,-1.));
#140862=DIRECTION('center_axis',(-1.,7.66554070360109E-15,0.));
#140863=DIRECTION('ref_axis',(-7.66554070360109E-15,-1.,0.));
#140864=DIRECTION('',(0.,0.,-1.));
#140865=DIRECTION('center_axis',(0.,0.,-1.));
#140866=DIRECTION('ref_axis',(-1.,0.,0.));
#140867=DIRECTION('',(0.,0.,-1.));
#140868=DIRECTION('center_axis',(-0.707106781186544,0.707106781186552,0.));
#140869=DIRECTION('ref_axis',(-0.707106781186552,-0.707106781186544,0.));
#140870=DIRECTION('',(0.,0.,-1.));
#140871=DIRECTION('center_axis',(0.,0.,-1.));
#140872=DIRECTION('ref_axis',(-1.,0.,0.));
#140873=DIRECTION('',(0.,0.,-1.));
#140874=DIRECTION('center_axis',(-1.,7.80891617653129E-15,0.));
#140875=DIRECTION('ref_axis',(-7.80891617653129E-15,-1.,0.));
#140876=DIRECTION('',(0.,0.,-1.));
#140877=DIRECTION('center_axis',(-0.707106781186548,0.707106781186548,0.));
#140878=DIRECTION('ref_axis',(-0.707106781186548,-0.707106781186548,0.));
#140879=DIRECTION('',(0.,0.,-1.));
#140880=DIRECTION('center_axis',(-5.01365166467286E-16,1.,0.));
#140881=DIRECTION('ref_axis',(-1.,-5.01365166467286E-16,0.));
#140882=DIRECTION('',(0.,0.,-1.));
#140883=DIRECTION('center_axis',(0.,0.,-1.));
#140884=DIRECTION('ref_axis',(-1.,0.,0.));
#140885=DIRECTION('',(0.,0.,-1.));
#140886=DIRECTION('center_axis',(-0.707106781186546,0.707106781186549,0.));
#140887=DIRECTION('ref_axis',(-0.707106781186549,-0.707106781186546,0.));
#140888=DIRECTION('',(0.,0.,-1.));
#140889=DIRECTION('center_axis',(0.,0.,-1.));
#140890=DIRECTION('ref_axis',(-1.,0.,0.));
#140891=DIRECTION('',(0.,0.,-1.));
#140892=DIRECTION('center_axis',(0.,1.,0.));
#140893=DIRECTION('ref_axis',(0.,0.,1.));
#140894=DIRECTION('',(0.,0.,-1.));
#140895=DIRECTION('center_axis',(0.,0.,-1.));
#140896=DIRECTION('ref_axis',(-1.,0.,0.));
#140897=DIRECTION('',(0.,0.,-1.));
#140898=DIRECTION('center_axis',(-1.,1.28023872765816E-15,0.));
#140899=DIRECTION('ref_axis',(-1.28023872765816E-15,-1.,0.));
#140900=DIRECTION('center_axis',(0.,3.67394039744206E-16,-1.));
#140901=DIRECTION('ref_axis',(0.,1.,3.67394039744206E-16));
#140902=DIRECTION('center_axis',(0.,0.,1.));
#140903=DIRECTION('ref_axis',(1.,0.,0.));
#140904=DIRECTION('',(0.,3.67394039744206E-16,-1.));
#140905=DIRECTION('center_axis',(0.,-3.67394039744206E-16,1.));
#140906=DIRECTION('ref_axis',(1.,0.,0.));
#140907=DIRECTION('',(0.,3.67394039744206E-16,-1.));
#140908=DIRECTION('center_axis',(0.,0.,-1.));
#140909=DIRECTION('ref_axis',(-1.,0.,0.));
#140910=DIRECTION('center_axis',(0.,-3.67394039744206E-16,1.));
#140911=DIRECTION('ref_axis',(-1.,0.,0.));
#140912=DIRECTION('',(-0.64144963156915,0.767165151815307,2.81851904276403E-16));
#140913=DIRECTION('center_axis',(0.,-3.67394039744206E-16,1.));
#140914=DIRECTION('ref_axis',(1.,0.,0.));
#140915=DIRECTION('',(0.641449631569149,0.767165151815306,2.81851904276403E-16));
#140916=DIRECTION('center_axis',(0.,-3.67394039744206E-16,1.));
#140917=DIRECTION('ref_axis',(1.,0.,0.));
#140918=DIRECTION('',(-0.767165151815301,-0.641449631569157,-2.35664771434625E-16));
#140919=DIRECTION('',(-0.767165151815311,0.641449631569145,2.35664771434621E-16));
#140920=DIRECTION('center_axis',(0.,-3.67394039744206E-16,1.));
#140921=DIRECTION('ref_axis',(1.,0.,0.));
#140922=DIRECTION('',(0.641449631569162,-0.767165151815296,-2.81851904276399E-16));
#140923=DIRECTION('center_axis',(0.,-3.67394039744206E-16,1.));
#140924=DIRECTION('ref_axis',(1.,0.,0.));
#140925=DIRECTION('',(-0.641449631569162,-0.767165151815296,-2.81851904276399E-16));
#140926=DIRECTION('center_axis',(0.,-3.67394039744206E-16,1.));
#140927=DIRECTION('ref_axis',(-1.,0.,0.));
#140928=DIRECTION('',(0.767165151815311,0.641449631569145,2.35664771434621E-16));
#140929=DIRECTION('center_axis',(0.,-3.67394039744206E-16,1.));
#140930=DIRECTION('ref_axis',(-1.,0.,0.));
#140931=DIRECTION('',(0.767165151815301,-0.641449631569157,-2.35664771434625E-16));
#140932=DIRECTION('center_axis',(0.641449631569157,0.767165151815301,2.818519042764E-16));
#140933=DIRECTION('ref_axis',(-0.767165151815301,0.641449631569157,-1.55481997605168E-32));
#140934=DIRECTION('',(0.,3.67394039744206E-16,-1.));
#140935=DIRECTION('',(0.767165151815301,-0.641449631569157,0.));
#140936=DIRECTION('',(0.,3.67394039744206E-16,-1.));
#140937=DIRECTION('center_axis',(0.,3.67394039744206E-16,-1.));
#140938=DIRECTION('ref_axis',(-1.96623899133175E-14,-1.,-3.67394039744206E-16));
#140939=DIRECTION('',(0.,3.67394039744206E-16,-1.));
#140940=DIRECTION('center_axis',(0.,0.,1.));
#140941=DIRECTION('ref_axis',(1.,0.,0.));
#140942=DIRECTION('center_axis',(-0.641449631569145,0.767165151815311,2.81851904276404E-16));
#140943=DIRECTION('ref_axis',(-0.767165151815311,-0.641449631569145,-2.53982072604054E-32));
#140944=DIRECTION('',(0.,3.67394039744206E-16,-1.));
#140945=DIRECTION('',(0.767165151815311,0.641449631569145,0.));
#140946=DIRECTION('center_axis',(0.,3.67394039744206E-16,-1.));
#140947=DIRECTION('ref_axis',(0.,1.,3.67394039744206E-16));
#140948=DIRECTION('',(0.,3.67394039744206E-16,-1.));
#140949=DIRECTION('center_axis',(0.,0.,1.));
#140950=DIRECTION('ref_axis',(1.,0.,0.));
#140951=DIRECTION('center_axis',(0.767165151815296,-0.641449631569162,-2.35664771434627E-16));
#140952=DIRECTION('ref_axis',(0.641449631569162,0.767165151815296,-1.58791937441479E-33));
#140953=DIRECTION('',(0.,3.67394039744206E-16,-1.));
#140954=DIRECTION('',(-0.641449631569162,-0.767165151815296,0.));
#140955=DIRECTION('center_axis',(0.,3.67394039744206E-16,-1.));
#140956=DIRECTION('ref_axis',(0.,1.,3.67394039744206E-16));
#140957=DIRECTION('',(0.,3.67394039744206E-16,-1.));
#140958=DIRECTION('center_axis',(0.,0.,1.));
#140959=DIRECTION('ref_axis',(1.,0.,0.));
#140960=DIRECTION('center_axis',(0.767165151815296,0.641449631569162,2.35664771434627E-16));
#140961=DIRECTION('ref_axis',(-0.641449631569162,0.767165151815296,-1.58791937441479E-33));
#140962=DIRECTION('',(0.,3.67394039744206E-16,-1.));
#140963=DIRECTION('',(0.641449631569162,-0.767165151815296,0.));
#140964=DIRECTION('center_axis',(0.,3.67394039744206E-16,-1.));
#140965=DIRECTION('ref_axis',(0.,1.,3.67394039744206E-16));
#140966=DIRECTION('',(0.,3.67394039744206E-16,-1.));
#140967=DIRECTION('center_axis',(0.,0.,1.));
#140968=DIRECTION('ref_axis',(1.,0.,0.));
#140969=DIRECTION('center_axis',(-0.641449631569145,-0.767165151815311,
-2.81851904276404E-16));
#140970=DIRECTION('ref_axis',(0.767165151815311,-0.641449631569145,-2.53982072604054E-32));
#140971=DIRECTION('',(-0.767165151815311,0.641449631569145,0.));
#140972=DIRECTION('center_axis',(0.641449631569157,-0.767165151815301,-2.818519042764E-16));
#140973=DIRECTION('ref_axis',(0.767165151815301,0.641449631569157,-1.55481997605168E-32));
#140974=DIRECTION('',(0.,3.67394039744206E-16,-1.));
#140975=DIRECTION('',(-0.767165151815301,-0.641449631569157,0.));
#140976=DIRECTION('center_axis',(0.,3.67394039744206E-16,-1.));
#140977=DIRECTION('ref_axis',(0.,1.,3.67394039744206E-16));
#140978=DIRECTION('',(0.,3.67394039744206E-16,-1.));
#140979=DIRECTION('center_axis',(0.,0.,1.));
#140980=DIRECTION('ref_axis',(1.,0.,0.));
#140981=DIRECTION('center_axis',(-0.767165151815307,0.64144963156915,2.35664771434622E-16));
#140982=DIRECTION('ref_axis',(-0.64144963156915,-0.767165151815306,6.82549510605368E-34));
#140983=DIRECTION('',(0.,3.67394039744206E-16,-1.));
#140984=DIRECTION('',(0.641449631569149,0.767165151815306,0.));
#140985=DIRECTION('center_axis',(0.,3.67394039744206E-16,-1.));
#140986=DIRECTION('ref_axis',(0.,1.,3.67394039744206E-16));
#140987=DIRECTION('',(0.,3.67394039744206E-16,-1.));
#140988=DIRECTION('center_axis',(0.,0.,1.));
#140989=DIRECTION('ref_axis',(1.,0.,0.));
#140990=DIRECTION('center_axis',(-0.767165151815307,-0.64144963156915,-2.35664771434622E-16));
#140991=DIRECTION('ref_axis',(0.64144963156915,-0.767165151815306,6.82549510605368E-34));
#140992=DIRECTION('',(0.,3.67394039744206E-16,-1.));
#140993=DIRECTION('',(-0.641449631569149,0.767165151815306,0.));
#140994=DIRECTION('center_axis',(0.,3.67394039744206E-16,-1.));
#140995=DIRECTION('ref_axis',(0.,1.,3.67394039744206E-16));
#140996=DIRECTION('center_axis',(0.,0.,1.));
#140997=DIRECTION('ref_axis',(1.,0.,0.));
#140998=DIRECTION('center_axis',(0.,0.,1.));
#140999=DIRECTION('ref_axis',(1.,0.,0.));
#141000=DIRECTION('center_axis',(0.,0.,-1.));
#141001=DIRECTION('ref_axis',(-1.,0.,0.));
#141002=DIRECTION('center_axis',(0.,-3.67394039744206E-16,1.));
#141003=DIRECTION('ref_axis',(-1.,0.,0.));
#141004=DIRECTION('',(-1.,0.,0.));
#141005=DIRECTION('center_axis',(0.,-3.67394039744206E-16,1.));
#141006=DIRECTION('ref_axis',(-1.,0.,0.));
#141007=DIRECTION('',(0.,-1.,-3.67394039744206E-16));
#141008=DIRECTION('center_axis',(0.,-3.67394039744206E-16,1.));
#141009=DIRECTION('ref_axis',(-1.,0.,0.));
#141010=DIRECTION('',(1.,1.57059617562415E-15,5.77027673769358E-31));
#141011=DIRECTION('center_axis',(0.,-3.67394039744206E-16,1.));
#141012=DIRECTION('ref_axis',(-1.,0.,0.));
#141013=DIRECTION('',(0.,1.,3.67394039744206E-16));
#141014=DIRECTION('center_axis',(-1.,0.,0.));
#141015=DIRECTION('ref_axis',(0.,0.,1.));
#141016=DIRECTION('',(0.,3.67394039744206E-16,-1.));
#141017=DIRECTION('',(0.,1.,0.));
#141018=DIRECTION('',(0.,3.67394039744206E-16,-1.));
#141019=DIRECTION('center_axis',(0.,3.67394039744206E-16,-1.));
#141020=DIRECTION('ref_axis',(0.,1.,3.67394039744206E-16));
#141021=DIRECTION('',(0.,3.67394039744206E-16,-1.));
#141022=DIRECTION('center_axis',(0.,0.,1.));
#141023=DIRECTION('ref_axis',(1.,0.,0.));
#141024=DIRECTION('center_axis',(-1.57059617562415E-15,1.,3.67394039744206E-16));
#141025=DIRECTION('ref_axis',(-1.,-1.57059617562415E-15,0.));
#141026=DIRECTION('',(0.,3.67394039744206E-16,-1.));
#141027=DIRECTION('',(1.,1.57059617562415E-15,0.));
#141028=DIRECTION('center_axis',(0.,3.67394039744206E-16,-1.));
#141029=DIRECTION('ref_axis',(0.,1.,3.67394039744206E-16));
#141030=DIRECTION('',(0.,3.67394039744206E-16,-1.));
#141031=DIRECTION('center_axis',(0.,0.,1.));
#141032=DIRECTION('ref_axis',(1.,0.,0.));
#141033=DIRECTION('center_axis',(1.,0.,0.));
#141034=DIRECTION('ref_axis',(0.,0.,-1.));
#141035=DIRECTION('',(0.,3.67394039744206E-16,-1.));
#141036=DIRECTION('',(0.,-1.,0.));
#141037=DIRECTION('center_axis',(0.,3.67394039744206E-16,-1.));
#141038=DIRECTION('ref_axis',(0.,1.,3.67394039744206E-16));
#141039=DIRECTION('',(0.,3.67394039744206E-16,-1.));
#141040=DIRECTION('center_axis',(0.,0.,1.));
#141041=DIRECTION('ref_axis',(1.,0.,0.));
#141042=DIRECTION('center_axis',(0.,-1.,-3.67394039744206E-16));
#141043=DIRECTION('ref_axis',(0.,3.67394039744206E-16,-1.));
#141044=DIRECTION('',(0.,3.67394039744206E-16,-1.));
#141045=DIRECTION('',(-1.,0.,0.));
#141046=DIRECTION('center_axis',(0.,3.67394039744206E-16,-1.));
#141047=DIRECTION('ref_axis',(0.,1.,3.67394039744206E-16));
#141048=DIRECTION('center_axis',(0.,0.,1.));
#141049=DIRECTION('ref_axis',(1.,0.,0.));
#141050=DIRECTION('center_axis',(0.,0.,1.));
#141051=DIRECTION('ref_axis',(1.,0.,0.));
#141052=DIRECTION('center_axis',(-1.83697019872103E-16,1.83697019872104E-16,
-1.));
#141053=DIRECTION('ref_axis',(3.37445951098919E-32,1.,1.83697019872104E-16));
#141054=DIRECTION('center_axis',(0.,0.,1.));
#141055=DIRECTION('ref_axis',(1.,0.,0.));
#141056=DIRECTION('',(-1.83697019872103E-16,1.83697019872104E-16,-1.));
#141057=DIRECTION('center_axis',(1.83697019872103E-16,-1.83697019872104E-16,
1.));
#141058=DIRECTION('ref_axis',(3.30423519233678E-15,1.,1.83697019872103E-16));
#141059=DIRECTION('',(-1.83697019872103E-16,1.83697019872104E-16,-1.));
#141060=DIRECTION('center_axis',(0.,0.,-1.));
#141061=DIRECTION('ref_axis',(-1.,0.,0.));
#141062=DIRECTION('center_axis',(1.83697019872103E-16,-1.83697019872104E-16,
1.));
#141063=DIRECTION('ref_axis',(-3.49686235279956E-15,-1.,-1.83697019872103E-16));
#141064=DIRECTION('',(-0.767165151815309,-0.641449631569147,2.30935664208905E-17));
#141065=DIRECTION('',(-0.767165151815304,0.641449631569152,2.58758337855513E-16));
#141066=DIRECTION('center_axis',(1.83697019872103E-16,-1.83697019872104E-16,
1.));
#141067=DIRECTION('ref_axis',(3.49686235279957E-15,1.,1.83697019872103E-16));
#141068=DIRECTION('',(0.641449631569154,-0.767165151815303,-2.58758337855513E-16));
#141069=DIRECTION('center_axis',(1.83697019872103E-16,-1.83697019872104E-16,
1.));
#141070=DIRECTION('ref_axis',(3.30423519233678E-15,1.,1.83697019872103E-16));
#141071=DIRECTION('',(-0.641449631569147,-0.767165151815308,-2.30935664208913E-17));
#141072=DIRECTION('center_axis',(1.83697019872103E-16,-1.83697019872104E-16,
1.));
#141073=DIRECTION('ref_axis',(3.49686235279957E-15,1.,1.83697019872103E-16));
#141074=DIRECTION('',(0.767165151815299,0.641449631569159,-2.30935664208864E-17));
#141075=DIRECTION('center_axis',(1.83697019872103E-16,-1.83697019872104E-16,
1.));
#141076=DIRECTION('ref_axis',(3.30423519233678E-15,1.,1.83697019872103E-16));
#141077=DIRECTION('',(0.767165151815294,-0.641449631569164,-2.58758337855513E-16));
#141078=DIRECTION('center_axis',(1.83697019872103E-16,-1.83697019872104E-16,
1.));
#141079=DIRECTION('ref_axis',(-3.49686235279957E-15,-1.,-1.83697019872103E-16));
#141080=DIRECTION('',(-0.641449631569142,0.767165151815313,2.58758337855513E-16));
#141081=DIRECTION('center_axis',(1.83697019872103E-16,-1.83697019872104E-16,
1.));
#141082=DIRECTION('ref_axis',(-3.30423519233678E-15,-1.,-1.83697019872103E-16));
#141083=DIRECTION('',(0.641449631569159,0.767165151815299,2.30935664208873E-17));
#141084=DIRECTION('center_axis',(-0.767165151815299,0.641449631569159,2.58758337855513E-16));
#141085=DIRECTION('ref_axis',(-0.641449631569159,-0.767165151815298,2.46315430569441E-34));
#141086=DIRECTION('',(-1.83697019872103E-16,1.83697019872104E-16,-1.));
#141087=DIRECTION('',(0.641449631569159,0.767165151815299,0.));
#141088=DIRECTION('',(-1.83697019872103E-16,1.83697019872104E-16,-1.));
#141089=DIRECTION('center_axis',(-1.83697019872103E-16,1.83697019872104E-16,
-1.));
#141090=DIRECTION('ref_axis',(3.37445951098919E-32,1.,1.83697019872104E-16));
#141091=DIRECTION('',(-1.83697019872103E-16,1.83697019872104E-16,-1.));
#141092=DIRECTION('center_axis',(0.,0.,1.));
#141093=DIRECTION('ref_axis',(1.,0.,0.));
#141094=DIRECTION('center_axis',(-0.767165151815313,-0.641449631569142,
2.30935664208922E-17));
#141095=DIRECTION('ref_axis',(0.641449631569142,-0.767165151815313,1.8129589684176E-33));
#141096=DIRECTION('',(-1.83697019872103E-16,1.83697019872104E-16,-1.));
#141097=DIRECTION('',(-0.641449631569142,0.767165151815313,0.));
#141098=DIRECTION('center_axis',(-1.83697019872103E-16,1.83697019872104E-16,
-1.));
#141099=DIRECTION('ref_axis',(3.37445951098919E-32,1.,1.83697019872104E-16));
#141100=DIRECTION('',(-1.83697019872103E-16,1.83697019872104E-16,-1.));
#141101=DIRECTION('center_axis',(0.,0.,1.));
#141102=DIRECTION('ref_axis',(1.,0.,0.));
#141103=DIRECTION('center_axis',(0.641449631569165,0.767165151815294,2.30935664208855E-17));
#141104=DIRECTION('ref_axis',(-0.767165151815294,0.641449631569165,-3.14801159113747E-34));
#141105=DIRECTION('',(-1.83697019872103E-16,1.83697019872104E-16,-1.));
#141106=DIRECTION('',(0.767165151815294,-0.641449631569164,0.));
#141107=DIRECTION('center_axis',(-1.83697019872103E-16,1.83697019872104E-16,
-1.));
#141108=DIRECTION('ref_axis',(-2.23269251724179E-14,-1.,-1.836970198721E-16));
#141109=DIRECTION('',(-1.83697019872103E-16,1.83697019872104E-16,-1.));
#141110=DIRECTION('center_axis',(0.,0.,1.));
#141111=DIRECTION('ref_axis',(1.,0.,0.));
#141112=DIRECTION('center_axis',(-0.641449631569159,0.767165151815299,2.58758337855513E-16));
#141113=DIRECTION('ref_axis',(-0.767165151815298,-0.641449631569159,-9.84827031361874E-33));
#141114=DIRECTION('',(-1.83697019872103E-16,1.83697019872104E-16,-1.));
#141115=DIRECTION('',(0.767165151815299,0.641449631569159,0.));
#141116=DIRECTION('center_axis',(-1.83697019872103E-16,1.83697019872104E-16,
-1.));
#141117=DIRECTION('ref_axis',(3.37445951098919E-32,1.,1.83697019872104E-16));
#141118=DIRECTION('',(-1.83697019872103E-16,1.83697019872104E-16,-1.));
#141119=DIRECTION('center_axis',(0.,0.,1.));
#141120=DIRECTION('ref_axis',(1.,0.,0.));
#141121=DIRECTION('center_axis',(0.767165151815308,-0.641449631569147,-2.58758337855513E-16));
#141122=DIRECTION('ref_axis',(0.641449631569147,0.767165151815308,2.26488733284622E-32));
#141123=DIRECTION('',(-1.83697019872103E-16,1.83697019872104E-16,-1.));
#141124=DIRECTION('',(-0.641449631569147,-0.767165151815308,0.));
#141125=DIRECTION('center_axis',(-1.83697019872103E-16,1.83697019872104E-16,
-1.));
#141126=DIRECTION('ref_axis',(3.37445951098919E-32,1.,1.83697019872104E-16));
#141127=DIRECTION('',(-1.83697019872103E-16,1.83697019872104E-16,-1.));
#141128=DIRECTION('center_axis',(0.,0.,1.));
#141129=DIRECTION('ref_axis',(1.,0.,0.));
#141130=DIRECTION('center_axis',(0.767165151815303,0.641449631569154,-2.30935664208882E-17));
#141131=DIRECTION('ref_axis',(-0.641449631569154,0.767165151815303,4.78565540702031E-34));
#141132=DIRECTION('',(-1.83697019872103E-16,1.83697019872104E-16,-1.));
#141133=DIRECTION('',(0.641449631569154,-0.767165151815303,0.));
#141134=DIRECTION('center_axis',(-1.83697019872103E-16,1.83697019872104E-16,
-1.));
#141135=DIRECTION('ref_axis',(3.37445951098919E-32,1.,1.83697019872104E-16));
#141136=DIRECTION('',(-1.83697019872103E-16,1.83697019872104E-16,-1.));
#141137=DIRECTION('center_axis',(0.,0.,1.));
#141138=DIRECTION('ref_axis',(1.,0.,0.));
#141139=DIRECTION('center_axis',(-0.641449631569152,-0.767165151815304,
-2.30935664208896E-17));
#141140=DIRECTION('ref_axis',(0.767165151815304,-0.641449631569152,-1.89368129222539E-33));
#141141=DIRECTION('',(-0.767165151815304,0.641449631569152,0.));
#141142=DIRECTION('center_axis',(0.641449631569147,-0.767165151815309,-2.58758337855513E-16));
#141143=DIRECTION('ref_axis',(0.767165151815309,0.641449631569147,2.01792103840072E-32));
#141144=DIRECTION('',(-1.83697019872103E-16,1.83697019872104E-16,-1.));
#141145=DIRECTION('',(-0.767165151815309,-0.641449631569147,0.));
#141146=DIRECTION('center_axis',(-1.83697019872103E-16,1.83697019872104E-16,
-1.));
#141147=DIRECTION('ref_axis',(3.37445951098919E-32,1.,1.83697019872104E-16));
#141148=DIRECTION('center_axis',(0.,0.,1.));
#141149=DIRECTION('ref_axis',(1.,0.,0.));
#141150=DIRECTION('center_axis',(0.,0.,1.));
#141151=DIRECTION('ref_axis',(1.,0.,0.));
#141152=DIRECTION('center_axis',(0.,0.,-1.));
#141153=DIRECTION('ref_axis',(-1.,0.,0.));
#141154=DIRECTION('center_axis',(1.83697019872103E-16,-1.83697019872104E-16,
1.));
#141155=DIRECTION('ref_axis',(-3.85494105772625E-15,-1.,-1.83697019872103E-16));
#141156=DIRECTION('',(-3.49148133884313E-15,-1.,-1.83697019872103E-16));
#141157=DIRECTION('center_axis',(1.83697019872103E-16,-1.83697019872104E-16,
1.));
#141158=DIRECTION('ref_axis',(-3.85494105772625E-15,-1.,-1.83697019872103E-16));
#141159=DIRECTION('',(1.,-3.49148133884313E-15,-1.83697019872104E-16));
#141160=DIRECTION('center_axis',(1.83697019872103E-16,-1.83697019872104E-16,
1.));
#141161=DIRECTION('ref_axis',(-3.85494105772625E-15,-1.,-1.83697019872103E-16));
#141162=DIRECTION('',(1.92088516321898E-15,1.,1.83697019872103E-16));
#141163=DIRECTION('center_axis',(1.83697019872103E-16,-1.83697019872104E-16,
1.));
#141164=DIRECTION('ref_axis',(-3.85494105772623E-15,-1.,-1.83697019872103E-16));
#141165=DIRECTION('',(-1.,3.49148133884313E-15,1.83697019872104E-16));
#141166=DIRECTION('center_axis',(-3.49148133884313E-15,-1.,-1.83697019872103E-16));
#141167=DIRECTION('ref_axis',(1.,-3.49148133884313E-15,0.));
#141168=DIRECTION('',(-1.83697019872103E-16,1.83697019872104E-16,-1.));
#141169=DIRECTION('',(-1.,3.49148133884313E-15,0.));
#141170=DIRECTION('',(-1.83697019872103E-16,1.83697019872104E-16,-1.));
#141171=DIRECTION('center_axis',(-1.83697019872103E-16,1.83697019872104E-16,
-1.));
#141172=DIRECTION('ref_axis',(3.37445951098919E-32,1.,1.83697019872104E-16));
#141173=DIRECTION('',(-1.83697019872103E-16,1.83697019872104E-16,-1.));
#141174=DIRECTION('center_axis',(0.,0.,1.));
#141175=DIRECTION('ref_axis',(1.,0.,0.));
#141176=DIRECTION('center_axis',(-1.,1.92088516321898E-15,1.83697019872103E-16));
#141177=DIRECTION('ref_axis',(-1.92088516321898E-15,-1.,8.36251867343314E-49));
#141178=DIRECTION('',(-1.83697019872103E-16,1.83697019872104E-16,-1.));
#141179=DIRECTION('',(1.92088516321898E-15,1.,0.));
#141180=DIRECTION('center_axis',(-1.83697019872103E-16,1.83697019872104E-16,
-1.));
#141181=DIRECTION('ref_axis',(3.37445951098919E-32,1.,1.83697019872104E-16));
#141182=DIRECTION('',(-1.83697019872103E-16,1.83697019872104E-16,-1.));
#141183=DIRECTION('center_axis',(0.,0.,1.));
#141184=DIRECTION('ref_axis',(1.,0.,0.));
#141185=DIRECTION('center_axis',(3.49148133884313E-15,1.,1.83697019872103E-16));
#141186=DIRECTION('ref_axis',(-1.,3.49148133884313E-15,0.));
#141187=DIRECTION('',(-1.83697019872103E-16,1.83697019872104E-16,-1.));
#141188=DIRECTION('',(1.,-3.49148133884313E-15,0.));
#141189=DIRECTION('center_axis',(-1.83697019872103E-16,1.83697019872104E-16,
-1.));
#141190=DIRECTION('ref_axis',(3.37445951098919E-32,1.,1.83697019872104E-16));
#141191=DIRECTION('',(-1.83697019872103E-16,1.83697019872104E-16,-1.));
#141192=DIRECTION('center_axis',(0.,0.,1.));
#141193=DIRECTION('ref_axis',(1.,0.,0.));
#141194=DIRECTION('center_axis',(1.,-3.49148133884313E-15,-1.83697019872104E-16));
#141195=DIRECTION('ref_axis',(3.49148133884313E-15,1.,-1.78914547131776E-47));
#141196=DIRECTION('',(-1.83697019872103E-16,1.83697019872104E-16,-1.));
#141197=DIRECTION('',(-3.49148133884313E-15,-1.,0.));
#141198=DIRECTION('center_axis',(-1.83697019872103E-16,1.83697019872104E-16,
-1.));
#141199=DIRECTION('ref_axis',(3.37445951098919E-32,1.,1.83697019872104E-16));
#141200=DIRECTION('center_axis',(0.,0.,1.));
#141201=DIRECTION('ref_axis',(1.,0.,0.));
#141202=DIRECTION('center_axis',(0.,0.,1.));
#141203=DIRECTION('ref_axis',(1.,0.,0.));
#141204=DIRECTION('center_axis',(0.,0.,-1.));
#141205=DIRECTION('ref_axis',(-1.,0.,0.));
#141206=DIRECTION('center_axis',(0.,0.,1.));
#141207=DIRECTION('ref_axis',(1.,0.,0.));
#141208=DIRECTION('',(0.,0.,-1.));
#141209=DIRECTION('center_axis',(0.,0.,1.));
#141210=DIRECTION('ref_axis',(-1.,0.,0.));
#141211=DIRECTION('',(0.,0.,-1.));
#141212=DIRECTION('center_axis',(0.,0.,-1.));
#141213=DIRECTION('ref_axis',(-1.,0.,0.));
#141214=DIRECTION('center_axis',(0.,0.,1.));
#141215=DIRECTION('ref_axis',(1.,0.,0.));
#141216=DIRECTION('',(0.641449631569149,-0.767165151815306,0.));
#141217=DIRECTION('',(-0.641449631569149,-0.767165151815306,0.));
#141218=DIRECTION('center_axis',(0.,0.,1.));
#141219=DIRECTION('ref_axis',(-1.,0.,0.));
#141220=DIRECTION('',(0.767165151815301,0.641449631569157,0.));
#141221=DIRECTION('center_axis',(0.,0.,1.));
#141222=DIRECTION('ref_axis',(-1.,0.,0.));
#141223=DIRECTION('',(0.767165151815311,-0.641449631569145,0.));
#141224=DIRECTION('center_axis',(0.,0.,1.));
#141225=DIRECTION('ref_axis',(-1.,0.,0.));
#141226=DIRECTION('',(-0.641449631569162,0.767165151815296,0.));
#141227=DIRECTION('center_axis',(0.,0.,1.));
#141228=DIRECTION('ref_axis',(-1.,0.,0.));
#141229=DIRECTION('',(0.641449631569162,0.767165151815296,0.));
#141230=DIRECTION('center_axis',(0.,0.,1.));
#141231=DIRECTION('ref_axis',(1.,0.,0.));
#141232=DIRECTION('',(-0.767165151815311,-0.641449631569145,0.));
#141233=DIRECTION('center_axis',(0.,0.,1.));
#141234=DIRECTION('ref_axis',(1.,0.,0.));
#141235=DIRECTION('',(-0.767165151815301,0.641449631569157,0.));
#141236=DIRECTION('center_axis',(-0.641449631569157,-0.767165151815301,
0.));
#141237=DIRECTION('ref_axis',(0.767165151815301,-0.641449631569157,0.));
#141238=DIRECTION('',(0.,0.,-1.));
#141239=DIRECTION('',(-0.767165151815301,0.641449631569157,0.));
#141240=DIRECTION('',(0.,0.,-1.));
#141241=DIRECTION('center_axis',(0.,0.,-1.));
#141242=DIRECTION('ref_axis',(-1.,0.,0.));
#141243=DIRECTION('',(0.,0.,-1.));
#141244=DIRECTION('center_axis',(0.,0.,1.));
#141245=DIRECTION('ref_axis',(1.,0.,0.));
#141246=DIRECTION('center_axis',(0.641449631569145,-0.767165151815311,0.));
#141247=DIRECTION('ref_axis',(0.767165151815311,0.641449631569145,0.));
#141248=DIRECTION('',(0.,0.,-1.));
#141249=DIRECTION('',(-0.767165151815311,-0.641449631569145,0.));
#141250=DIRECTION('center_axis',(0.,0.,-1.));
#141251=DIRECTION('ref_axis',(-1.,0.,0.));
#141252=DIRECTION('',(0.,0.,-1.));
#141253=DIRECTION('center_axis',(0.,0.,1.));
#141254=DIRECTION('ref_axis',(1.,0.,0.));
#141255=DIRECTION('center_axis',(-0.767165151815296,0.641449631569162,0.));
#141256=DIRECTION('ref_axis',(-0.641449631569162,-0.767165151815296,0.));
#141257=DIRECTION('',(0.,0.,-1.));
#141258=DIRECTION('',(0.641449631569162,0.767165151815296,0.));
#141259=DIRECTION('center_axis',(0.,0.,-1.));
#141260=DIRECTION('ref_axis',(1.,7.6571373978539E-16,0.));
#141261=DIRECTION('',(0.,0.,-1.));
#141262=DIRECTION('center_axis',(0.,0.,1.));
#141263=DIRECTION('ref_axis',(1.,0.,0.));
#141264=DIRECTION('center_axis',(-0.767165151815296,-0.641449631569162,
0.));
#141265=DIRECTION('ref_axis',(0.641449631569162,-0.767165151815296,0.));
#141266=DIRECTION('',(0.,0.,-1.));
#141267=DIRECTION('',(-0.641449631569162,0.767165151815296,0.));
#141268=DIRECTION('center_axis',(0.,0.,-1.));
#141269=DIRECTION('ref_axis',(-1.,0.,0.));
#141270=DIRECTION('',(0.,0.,-1.));
#141271=DIRECTION('center_axis',(0.,0.,1.));
#141272=DIRECTION('ref_axis',(1.,0.,0.));
#141273=DIRECTION('center_axis',(0.641449631569145,0.767165151815311,0.));
#141274=DIRECTION('ref_axis',(-0.767165151815311,0.641449631569145,0.));
#141275=DIRECTION('',(0.,0.,-1.));
#141276=DIRECTION('',(0.767165151815311,-0.641449631569145,0.));
#141277=DIRECTION('center_axis',(0.,0.,-1.));
#141278=DIRECTION('ref_axis',(-1.,0.,0.));
#141279=DIRECTION('',(0.,0.,-1.));
#141280=DIRECTION('center_axis',(0.,0.,1.));
#141281=DIRECTION('ref_axis',(1.,0.,0.));
#141282=DIRECTION('center_axis',(-0.641449631569157,0.767165151815301,0.));
#141283=DIRECTION('ref_axis',(-0.767165151815301,-0.641449631569157,0.));
#141284=DIRECTION('',(0.,0.,-1.));
#141285=DIRECTION('',(0.767165151815301,0.641449631569157,0.));
#141286=DIRECTION('center_axis',(0.,0.,-1.));
#141287=DIRECTION('ref_axis',(-1.,0.,0.));
#141288=DIRECTION('',(0.,0.,-1.));
#141289=DIRECTION('center_axis',(0.,0.,1.));
#141290=DIRECTION('ref_axis',(1.,0.,0.));
#141291=DIRECTION('center_axis',(0.767165151815307,-0.64144963156915,0.));
#141292=DIRECTION('ref_axis',(0.64144963156915,0.767165151815306,0.));
#141293=DIRECTION('',(-0.641449631569149,-0.767165151815306,0.));
#141294=DIRECTION('center_axis',(0.767165151815307,0.64144963156915,0.));
#141295=DIRECTION('ref_axis',(-0.64144963156915,0.767165151815306,0.));
#141296=DIRECTION('',(0.,0.,-1.));
#141297=DIRECTION('',(0.641449631569149,-0.767165151815306,0.));
#141298=DIRECTION('center_axis',(0.,0.,-1.));
#141299=DIRECTION('ref_axis',(-1.,0.,0.));
#141300=DIRECTION('center_axis',(0.,0.,1.));
#141301=DIRECTION('ref_axis',(1.,0.,0.));
#141302=DIRECTION('center_axis',(0.,0.,1.));
#141303=DIRECTION('ref_axis',(1.,0.,0.));
#141304=DIRECTION('center_axis',(0.,0.,-1.));
#141305=DIRECTION('ref_axis',(-1.,0.,0.));
#141306=DIRECTION('center_axis',(0.,0.,1.));
#141307=DIRECTION('ref_axis',(1.,0.,0.));
#141308=DIRECTION('',(1.,0.,0.));
#141309=DIRECTION('center_axis',(0.,0.,1.));
#141310=DIRECTION('ref_axis',(1.,0.,0.));
#141311=DIRECTION('',(0.,1.,0.));
#141312=DIRECTION('center_axis',(0.,0.,1.));
#141313=DIRECTION('ref_axis',(1.,0.,0.));
#141314=DIRECTION('',(-1.,-1.57059617562415E-15,0.));
#141315=DIRECTION('center_axis',(0.,0.,1.));
#141316=DIRECTION('ref_axis',(1.,0.,0.));
#141317=DIRECTION('',(0.,-1.,0.));
#141318=DIRECTION('center_axis',(1.,0.,0.));
#141319=DIRECTION('ref_axis',(0.,0.,-1.));
#141320=DIRECTION('',(0.,0.,-1.));
#141321=DIRECTION('',(0.,-1.,0.));
#141322=DIRECTION('',(0.,0.,-1.));
#141323=DIRECTION('center_axis',(0.,0.,-1.));
#141324=DIRECTION('ref_axis',(-1.,0.,0.));
#141325=DIRECTION('',(0.,0.,-1.));
#141326=DIRECTION('center_axis',(0.,0.,1.));
#141327=DIRECTION('ref_axis',(1.,0.,0.));
#141328=DIRECTION('center_axis',(1.57059617562415E-15,-1.,0.));
#141329=DIRECTION('ref_axis',(1.,1.57059617562415E-15,0.));
#141330=DIRECTION('',(0.,0.,-1.));
#141331=DIRECTION('',(-1.,-1.57059617562415E-15,0.));
#141332=DIRECTION('center_axis',(0.,0.,-1.));
#141333=DIRECTION('ref_axis',(-1.,0.,0.));
#141334=DIRECTION('',(0.,0.,-1.));
#141335=DIRECTION('center_axis',(0.,0.,1.));
#141336=DIRECTION('ref_axis',(1.,0.,0.));
#141337=DIRECTION('center_axis',(-1.,0.,0.));
#141338=DIRECTION('ref_axis',(0.,0.,1.));
#141339=DIRECTION('',(0.,0.,-1.));
#141340=DIRECTION('',(0.,1.,0.));
#141341=DIRECTION('center_axis',(0.,0.,-1.));
#141342=DIRECTION('ref_axis',(-1.,0.,0.));
#141343=DIRECTION('',(0.,0.,-1.));
#141344=DIRECTION('center_axis',(0.,0.,1.));
#141345=DIRECTION('ref_axis',(1.,0.,0.));
#141346=DIRECTION('center_axis',(0.,1.,0.));
#141347=DIRECTION('ref_axis',(0.,0.,1.));
#141348=DIRECTION('',(0.,0.,-1.));
#141349=DIRECTION('',(1.,0.,0.));
#141350=DIRECTION('center_axis',(0.,0.,-1.));
#141351=DIRECTION('ref_axis',(-1.,0.,0.));
#141352=DIRECTION('center_axis',(0.,0.,1.));
#141353=DIRECTION('ref_axis',(1.,0.,0.));
#141354=DIRECTION('center_axis',(0.,0.,1.));
#141355=DIRECTION('ref_axis',(1.,0.,0.));
#141356=DIRECTION('center_axis',(-2.1350442781253E-15,1.,0.));
#141357=DIRECTION('ref_axis',(-1.,-2.1350442781253E-15,0.));
#141358=DIRECTION('',(1.,2.1350442781253E-15,0.));
#141359=DIRECTION('',(0.,0.,-1.));
#141360=DIRECTION('',(1.,2.1350442781253E-15,0.));
#141361=DIRECTION('',(0.,0.,1.));
#141362=DIRECTION('center_axis',(-1.,2.1350442781253E-15,0.));
#141363=DIRECTION('ref_axis',(-2.1350442781253E-15,-1.,0.));
#141364=DIRECTION('',(2.1350442781253E-15,1.,0.));
#141365=DIRECTION('',(0.,0.,-1.));
#141366=DIRECTION('',(2.1350442781253E-15,1.,0.));
#141367=DIRECTION('',(0.,0.,-1.));
#141368=DIRECTION('center_axis',(0.866025403784438,0.500000000000001,0.));
#141369=DIRECTION('ref_axis',(-0.500000000000001,0.866025403784438,0.));
#141370=DIRECTION('',(0.5,-0.866025403784438,0.));
#141371=DIRECTION('',(0.,0.,-1.));
#141372=DIRECTION('',(0.5,-0.866025403784438,0.));
#141373=DIRECTION('',(0.,0.,-1.));
#141374=DIRECTION('center_axis',(0.866025403784438,-0.500000000000002,0.));
#141375=DIRECTION('ref_axis',(0.500000000000002,0.866025403784437,0.));
#141376=DIRECTION('',(-0.500000000000002,-0.866025403784438,0.));
#141377=DIRECTION('',(-0.500000000000002,-0.866025403784438,0.));
#141378=DIRECTION('',(0.,0.,-1.));
#141379=DIRECTION('center_axis',(1.,0.,0.));
#141380=DIRECTION('ref_axis',(0.,0.,-1.));
#141381=DIRECTION('',(0.,-1.,0.));
#141382=DIRECTION('',(0.,-1.,0.));
#141383=DIRECTION('',(0.,0.,-1.));
#141384=DIRECTION('center_axis',(0.,0.,-1.));
#141385=DIRECTION('ref_axis',(-1.,0.,0.));
#141386=DIRECTION('center_axis',(0.,0.,-1.));
#141387=DIRECTION('ref_axis',(1.,0.,0.));
#141388=DIRECTION('center_axis',(0.,0.,-1.));
#141389=DIRECTION('ref_axis',(-1.,0.,0.));
#141390=DIRECTION('',(0.,0.,-1.));
#141391=DIRECTION('center_axis',(0.707106781186548,-0.707106781186548,0.));
#141392=DIRECTION('ref_axis',(0.707106781186548,0.707106781186548,0.));
#141393=DIRECTION('',(-0.707106781186548,-0.707106781186548,0.));
#141394=DIRECTION('',(-0.707106781186548,-0.707106781186548,0.));
#141395=DIRECTION('',(0.,0.,-1.));
#141396=DIRECTION('center_axis',(0.,0.,-1.));
#141397=DIRECTION('ref_axis',(-1.,0.,0.));
#141398=DIRECTION('center_axis',(0.,0.,-1.));
#141399=DIRECTION('ref_axis',(1.,-3.85494105772625E-15,0.));
#141400=DIRECTION('center_axis',(0.,0.,-1.));
#141401=DIRECTION('ref_axis',(-1.,0.,0.));
#141402=DIRECTION('',(0.,0.,-1.));
#141403=DIRECTION('center_axis',(1.6719208893717E-15,-1.,0.));
#141404=DIRECTION('ref_axis',(1.,1.6719208893717E-15,0.));
#141405=DIRECTION('',(-1.,-1.6719208893717E-15,0.));
#141406=DIRECTION('',(-1.,-1.6719208893717E-15,0.));
#141407=DIRECTION('',(0.,0.,-1.));
#141408=DIRECTION('center_axis',(0.,0.,-1.));
#141409=DIRECTION('ref_axis',(-1.,0.,0.));
#141410=DIRECTION('center_axis',(0.,0.,-1.));
#141411=DIRECTION('ref_axis',(1.,0.,0.));
#141412=DIRECTION('center_axis',(0.,0.,-1.));
#141413=DIRECTION('ref_axis',(-1.,0.,0.));
#141414=DIRECTION('',(0.,0.,-1.));
#141415=DIRECTION('center_axis',(-1.,-2.1350442781253E-15,0.));
#141416=DIRECTION('ref_axis',(2.1350442781253E-15,-1.,0.));
#141417=DIRECTION('',(-2.1350442781253E-15,1.,0.));
#141418=DIRECTION('',(-2.1350442781253E-15,1.,0.));
#141419=DIRECTION('',(0.,0.,-1.));
#141420=DIRECTION('center_axis',(0.,0.,-1.));
#141421=DIRECTION('ref_axis',(-1.,0.,0.));
#141422=DIRECTION('center_axis',(0.,0.,1.));
#141423=DIRECTION('ref_axis',(1.,0.,0.));
#141424=DIRECTION('center_axis',(0.,0.,1.));
#141425=DIRECTION('ref_axis',(-1.,0.,0.));
#141426=DIRECTION('',(0.,0.,-1.));
#141427=DIRECTION('center_axis',(3.01691039300315E-15,-1.,0.));
#141428=DIRECTION('ref_axis',(1.,3.01691039300315E-15,0.));
#141429=DIRECTION('',(-1.,-3.01691039300315E-15,0.));
#141430=DIRECTION('',(-1.,-3.01691039300315E-15,0.));
#141431=DIRECTION('',(0.,0.,-1.));
#141432=DIRECTION('center_axis',(1.,0.,0.));
#141433=DIRECTION('ref_axis',(0.,0.,-1.));
#141434=DIRECTION('',(0.,-1.,0.));
#141435=DIRECTION('',(0.,-1.,0.));
#141436=DIRECTION('',(0.,0.,-1.));
#141437=DIRECTION('center_axis',(0.,-1.,0.));
#141438=DIRECTION('ref_axis',(0.,0.,-1.));
#141439=DIRECTION('',(-1.,0.,0.));
#141440=DIRECTION('',(-1.,0.,0.));
#141441=DIRECTION('',(0.,0.,-1.));
#141442=DIRECTION('center_axis',(1.,0.,0.));
#141443=DIRECTION('ref_axis',(0.,0.,-1.));
#141444=DIRECTION('',(0.,-1.,0.));
#141445=DIRECTION('',(0.,-1.,0.));
#141446=DIRECTION('',(1.83697019872103E-16,1.83697019872101E-16,-1.));
#141447=DIRECTION('center_axis',(-7.30409884621813E-15,-1.,0.));
#141448=DIRECTION('ref_axis',(1.,-7.30409884621813E-15,0.));
#141449=DIRECTION('',(-1.,7.30409884621813E-15,0.));
#141450=DIRECTION('',(-1.83697019872103E-16,1.83697019872104E-16,-1.));
#141451=DIRECTION('',(-1.,7.30409884621813E-15,0.));
#141452=DIRECTION('',(0.,0.,-1.));
#141453=DIRECTION('center_axis',(1.,-1.26161707343766E-14,0.));
#141454=DIRECTION('ref_axis',(1.26161707343766E-14,1.,0.));
#141455=DIRECTION('',(-1.26161707343766E-14,-1.,0.));
#141456=DIRECTION('',(-1.26161707343766E-14,-1.,0.));
#141457=DIRECTION('',(0.,0.,-1.));
#141458=DIRECTION('center_axis',(-6.30808536718845E-15,-1.,0.));
#141459=DIRECTION('ref_axis',(1.,-6.30808536718845E-15,0.));
#141460=DIRECTION('',(-1.,6.30808536718845E-15,0.));
#141461=DIRECTION('',(-1.,6.30808536718845E-15,0.));
#141462=DIRECTION('',(0.,0.,-1.));
#141463=DIRECTION('center_axis',(1.,-9.05073117900944E-15,0.));
#141464=DIRECTION('ref_axis',(9.05073117900944E-15,1.,0.));
#141465=DIRECTION('',(-9.05073117900944E-15,-1.,0.));
#141466=DIRECTION('',(-9.05073117900944E-15,-1.,0.));
#141467=DIRECTION('',(0.,0.,-1.));
#141468=DIRECTION('center_axis',(0.,0.,-1.));
#141469=DIRECTION('ref_axis',(-1.,0.,0.));
#141470=DIRECTION('center_axis',(0.,0.,1.));
#141471=DIRECTION('ref_axis',(1.,0.,0.));
#141472=DIRECTION('center_axis',(0.,0.,1.));
#141473=DIRECTION('ref_axis',(1.,0.,0.));
#141474=DIRECTION('',(0.,0.,-1.));
#141475=DIRECTION('center_axis',(8.5401771125012E-15,1.,0.));
#141476=DIRECTION('ref_axis',(-1.,8.5401771125012E-15,0.));
#141477=DIRECTION('',(1.,-8.5401771125012E-15,0.));
#141478=DIRECTION('',(1.,-8.5401771125012E-15,0.));
#141479=DIRECTION('',(0.,0.,-1.));
#141480=DIRECTION('center_axis',(0.,0.,-1.));
#141481=DIRECTION('ref_axis',(-1.,0.,0.));
#141482=DIRECTION('center_axis',(0.,0.,-1.));
#141483=DIRECTION('ref_axis',(1.,2.31296463463574E-14,0.));
#141484=DIRECTION('center_axis',(0.,0.,-1.));
#141485=DIRECTION('ref_axis',(1.,0.,0.));
#141486=DIRECTION('',(0.,0.,-1.));
#141487=DIRECTION('center_axis',(1.,-8.3596044468585E-15,0.));
#141488=DIRECTION('ref_axis',(8.3596044468585E-15,1.,0.));
#141489=DIRECTION('',(-8.3596044468585E-15,-1.,0.));
#141490=DIRECTION('',(-8.3596044468585E-15,-1.,0.));
#141491=DIRECTION('',(0.,0.,-1.));
#141492=DIRECTION('center_axis',(0.,0.,-1.));
#141493=DIRECTION('ref_axis',(-1.,0.,0.));
#141494=DIRECTION('center_axis',(0.,0.,-1.));
#141495=DIRECTION('ref_axis',(1.,-7.70988211545251E-15,0.));
#141496=DIRECTION('center_axis',(0.,0.,-1.));
#141497=DIRECTION('ref_axis',(1.,0.,0.));
#141498=DIRECTION('',(0.,0.,-1.));
#141499=DIRECTION('center_axis',(0.707106781186542,-0.707106781186553,0.));
#141500=DIRECTION('ref_axis',(0.707106781186553,0.707106781186542,0.));
#141501=DIRECTION('',(-0.707106781186553,-0.707106781186542,0.));
#141502=DIRECTION('',(-0.707106781186553,-0.707106781186542,0.));
#141503=DIRECTION('',(0.,0.,-1.));
#141504=DIRECTION('center_axis',(0.,0.,-1.));
#141505=DIRECTION('ref_axis',(-1.,0.,0.));
#141506=DIRECTION('center_axis',(0.,0.,-1.));
#141507=DIRECTION('ref_axis',(1.,0.,0.));
#141508=DIRECTION('center_axis',(0.,0.,-1.));
#141509=DIRECTION('ref_axis',(1.,0.,0.));
#141510=DIRECTION('',(0.,0.,-1.));
#141511=DIRECTION('center_axis',(-8.7284827903955E-15,-1.,0.));
#141512=DIRECTION('ref_axis',(1.,-8.7284827903955E-15,0.));
#141513=DIRECTION('',(-1.,8.7284827903955E-15,0.));
#141514=DIRECTION('',(-1.,8.7284827903955E-15,0.));
#141515=DIRECTION('',(0.,0.,-1.));
#141516=DIRECTION('center_axis',(0.499999999999979,-0.866025403784451,0.));
#141517=DIRECTION('ref_axis',(0.866025403784451,0.499999999999979,0.));
#141518=DIRECTION('',(-0.866025403784451,-0.499999999999979,0.));
#141519=DIRECTION('',(-0.866025403784451,-0.499999999999979,0.));
#141520=DIRECTION('',(0.,0.,-1.));
#141521=DIRECTION('center_axis',(-0.500000000000004,-0.866025403784436,
0.));
#141522=DIRECTION('ref_axis',(0.866025403784436,-0.500000000000004,0.));
#141523=DIRECTION('',(-0.866025403784436,0.500000000000004,0.));
#141524=DIRECTION('',(-0.866025403784436,0.500000000000004,0.));
#141525=DIRECTION('',(0.,0.,-1.));
#141526=DIRECTION('center_axis',(0.,-1.,0.));
#141527=DIRECTION('ref_axis',(0.,0.,-1.));
#141528=DIRECTION('',(-1.,0.,0.));
#141529=DIRECTION('',(-1.,0.,0.));
#141530=DIRECTION('',(0.,0.,-1.));
#141531=DIRECTION('center_axis',(0.,0.,-1.));
#141532=DIRECTION('ref_axis',(-1.,0.,0.));
#141533=DIRECTION('center_axis',(0.,0.,-1.));
#141534=DIRECTION('ref_axis',(1.,-7.70988211545249E-15,0.));
#141535=DIRECTION('center_axis',(0.,0.,-1.));
#141536=DIRECTION('ref_axis',(1.,0.,0.));
#141537=DIRECTION('',(0.,0.,-1.));
#141538=DIRECTION('center_axis',(-0.707106781186548,-0.707106781186548,
0.));
#141539=DIRECTION('ref_axis',(0.707106781186548,-0.707106781186548,0.));
#141540=DIRECTION('',(-0.707106781186548,0.707106781186548,0.));
#141541=DIRECTION('',(-0.707106781186548,0.707106781186548,0.));
#141542=DIRECTION('',(0.,0.,-1.));
#141543=DIRECTION('center_axis',(0.,0.,-1.));
#141544=DIRECTION('ref_axis',(-1.,0.,0.));
#141545=DIRECTION('center_axis',(0.,0.,-1.));
#141546=DIRECTION('ref_axis',(1.,0.,0.));
#141547=DIRECTION('center_axis',(0.,0.,-1.));
#141548=DIRECTION('ref_axis',(1.,0.,0.));
#141549=DIRECTION('',(0.,0.,-1.));
#141550=DIRECTION('center_axis',(-1.,0.,0.));
#141551=DIRECTION('ref_axis',(0.,0.,1.));
#141552=DIRECTION('',(0.,1.,0.));
#141553=DIRECTION('',(0.,1.,0.));
#141554=DIRECTION('',(0.,0.,-1.));
#141555=DIRECTION('center_axis',(0.,0.,-1.));
#141556=DIRECTION('ref_axis',(-1.,0.,0.));
#141557=DIRECTION('center_axis',(0.,0.,-1.));
#141558=DIRECTION('ref_axis',(1.,0.,0.));
#141559=DIRECTION('center_axis',(0.,0.,-1.));
#141560=DIRECTION('ref_axis',(1.,0.,0.));
#141561=DIRECTION('center_axis',(-2.1350442781253E-15,1.,0.));
#141562=DIRECTION('ref_axis',(-1.,-2.1350442781253E-15,0.));
#141563=DIRECTION('',(1.,2.1350442781253E-15,0.));
#141564=DIRECTION('',(0.,0.,-1.));
#141565=DIRECTION('',(1.,2.1350442781253E-15,0.));
#141566=DIRECTION('',(0.,0.,-1.));
#141567=DIRECTION('center_axis',(0.,0.,-1.));
#141568=DIRECTION('ref_axis',(-1.,0.,0.));
#141569=DIRECTION('center_axis',(0.,0.,1.));
#141570=DIRECTION('ref_axis',(1.,0.,0.));
#141571=DIRECTION('center_axis',(0.,0.,1.));
#141572=DIRECTION('ref_axis',(1.,0.,0.));
#141573=DIRECTION('',(0.,0.,-1.));
#141574=DIRECTION('center_axis',(-1.,0.,0.));
#141575=DIRECTION('ref_axis',(0.,0.,1.));
#141576=DIRECTION('',(0.,1.,0.));
#141577=DIRECTION('',(0.,1.,0.));
#141578=DIRECTION('',(0.,0.,-1.));
#141579=DIRECTION('center_axis',(0.,-1.,0.));
#141580=DIRECTION('ref_axis',(0.,0.,-1.));
#141581=DIRECTION('',(-1.,0.,0.));
#141582=DIRECTION('',(-1.,0.,0.));
#141583=DIRECTION('',(0.,0.,-1.));
#141584=DIRECTION('center_axis',(-1.,0.,0.));
#141585=DIRECTION('ref_axis',(0.,0.,1.));
#141586=DIRECTION('',(0.,1.,0.));
#141587=DIRECTION('',(0.,1.,0.));
#141588=DIRECTION('',(0.,0.,-1.));
#141589=DIRECTION('center_axis',(0.,-1.,0.));
#141590=DIRECTION('ref_axis',(0.,0.,-1.));
#141591=DIRECTION('',(-1.,0.,0.));
#141592=DIRECTION('',(-1.,0.,0.));
#141593=DIRECTION('',(0.,0.,-1.));
#141594=DIRECTION('center_axis',(0.,0.,-1.));
#141595=DIRECTION('ref_axis',(-1.,0.,0.));
#141596=DIRECTION('center_axis',(0.,0.,1.));
#141597=DIRECTION('ref_axis',(1.,0.,0.));
#141598=DIRECTION('center_axis',(0.,0.,1.));
#141599=DIRECTION('ref_axis',(1.,0.,0.));
#141600=DIRECTION('',(0.,0.,-1.));
#141601=DIRECTION('center_axis',(1.,-4.12146228552343E-16,0.));
#141602=DIRECTION('ref_axis',(4.12146228552343E-16,1.,0.));
#141603=DIRECTION('',(-4.12146228552343E-16,-1.,0.));
#141604=DIRECTION('',(-4.12146228552343E-16,-1.,0.));
#141605=DIRECTION('',(0.,0.,-1.));
#141606=DIRECTION('center_axis',(0.,1.,0.));
#141607=DIRECTION('ref_axis',(0.,0.,1.));
#141608=DIRECTION('',(1.,0.,0.));
#141609=DIRECTION('',(1.,0.,0.));
#141610=DIRECTION('',(0.,0.,-1.));
#141611=DIRECTION('center_axis',(1.,0.,0.));
#141612=DIRECTION('ref_axis',(0.,0.,-1.));
#141613=DIRECTION('',(0.,-1.,0.));
#141614=DIRECTION('',(0.,-1.,0.));
#141615=DIRECTION('',(0.,0.,-1.));
#141616=DIRECTION('center_axis',(3.01691039300315E-15,1.,0.));
#141617=DIRECTION('ref_axis',(-1.,3.01691039300315E-15,0.));
#141618=DIRECTION('',(1.,-3.01691039300315E-15,0.));
#141619=DIRECTION('',(1.,-3.01691039300315E-15,0.));
#141620=DIRECTION('',(0.,0.,-1.));
#141621=DIRECTION('center_axis',(0.,0.,-1.));
#141622=DIRECTION('ref_axis',(-1.,0.,0.));
#141623=DIRECTION('center_axis',(0.,0.,1.));
#141624=DIRECTION('ref_axis',(1.,0.,0.));
#141625=DIRECTION('center_axis',(0.,0.,1.));
#141626=DIRECTION('ref_axis',(1.,0.,0.));
#141627=DIRECTION('',(0.,0.,-1.));
#141628=DIRECTION('center_axis',(-1.,2.1350442781253E-15,0.));
#141629=DIRECTION('ref_axis',(-2.1350442781253E-15,-1.,0.));
#141630=DIRECTION('',(2.1350442781253E-15,1.,0.));
#141631=DIRECTION('',(2.1350442781253E-15,1.,0.));
#141632=DIRECTION('',(0.,0.,1.));
#141633=DIRECTION('center_axis',(0.,0.,-1.));
#141634=DIRECTION('ref_axis',(-1.,0.,0.));
#141635=DIRECTION('center_axis',(0.,0.,-1.));
#141636=DIRECTION('ref_axis',(1.,0.,0.));
#141637=DIRECTION('center_axis',(0.,0.,-1.));
#141638=DIRECTION('ref_axis',(1.,0.,0.));
#141639=DIRECTION('',(0.,0.,-1.));
#141640=DIRECTION('center_axis',(1.6719208893717E-15,1.,0.));
#141641=DIRECTION('ref_axis',(-1.,1.6719208893717E-15,0.));
#141642=DIRECTION('',(1.,-1.6719208893717E-15,0.));
#141643=DIRECTION('',(1.,-1.6719208893717E-15,0.));
#141644=DIRECTION('',(0.,0.,-1.));
#141645=DIRECTION('center_axis',(0.,0.,-1.));
#141646=DIRECTION('ref_axis',(-1.,0.,0.));
#141647=DIRECTION('center_axis',(0.,0.,-1.));
#141648=DIRECTION('ref_axis',(1.,0.,0.));
#141649=DIRECTION('center_axis',(0.,0.,-1.));
#141650=DIRECTION('ref_axis',(1.,0.,0.));
#141651=DIRECTION('',(0.,0.,-1.));
#141652=DIRECTION('center_axis',(0.707106781186548,0.707106781186548,0.));
#141653=DIRECTION('ref_axis',(-0.707106781186548,0.707106781186548,0.));
#141654=DIRECTION('',(0.707106781186547,-0.707106781186547,0.));
#141655=DIRECTION('',(0.707106781186547,-0.707106781186547,0.));
#141656=DIRECTION('',(0.,0.,-1.));
#141657=DIRECTION('center_axis',(0.,0.,-1.));
#141658=DIRECTION('ref_axis',(-1.,0.,0.));
#141659=DIRECTION('center_axis',(0.,0.,-1.));
#141660=DIRECTION('ref_axis',(1.,4.6259292692715E-14,0.));
#141661=DIRECTION('center_axis',(0.,0.,-1.));
#141662=DIRECTION('ref_axis',(1.,0.,0.));
#141663=DIRECTION('',(0.,0.,-1.));
#141664=DIRECTION('center_axis',(1.,0.,0.));
#141665=DIRECTION('ref_axis',(0.,0.,-1.));
#141666=DIRECTION('',(0.,-1.,0.));
#141667=DIRECTION('',(0.,-1.,0.));
#141668=DIRECTION('center_axis',(0.499999999999997,-0.86602540378444,-2.50934795744788E-16));
#141669=DIRECTION('ref_axis',(0.86602540378444,0.499999999999997,1.16566443650333E-32));
#141670=DIRECTION('',(-0.86602540378444,-0.499999999999997,0.));
#141671=DIRECTION('',(-1.83697019872103E-16,1.83697019872104E-16,-1.));
#141672=DIRECTION('',(-0.86602540378444,-0.499999999999997,6.7237775872685E-17));
#141673=DIRECTION('',(-1.83697019872103E-16,1.83697019872104E-16,-1.));
#141674=DIRECTION('center_axis',(-0.500000000000005,-0.866025403784436,
-6.72377758726837E-17));
#141675=DIRECTION('ref_axis',(0.866025403784436,-0.500000000000005,6.17106363235252E-33));
#141676=DIRECTION('',(-0.866025403784436,0.500000000000005,0.));
#141677=DIRECTION('',(-0.866025403784436,0.500000000000005,2.50934795744788E-16));
#141678=DIRECTION('',(-1.83697019872103E-16,1.83697019872104E-16,-1.));
#141679=DIRECTION('center_axis',(-3.49148133884313E-15,-1.,-1.83697019872103E-16));
#141680=DIRECTION('ref_axis',(1.,-3.49148133884313E-15,0.));
#141681=DIRECTION('',(-1.,3.49148133884313E-15,0.));
#141682=DIRECTION('',(-1.,3.49148133884313E-15,1.83697019872104E-16));
#141683=DIRECTION('',(-1.83697019872103E-16,1.83697019872104E-16,-1.));
#141684=DIRECTION('center_axis',(-1.83697019872103E-16,1.83697019872104E-16,
-1.));
#141685=DIRECTION('ref_axis',(3.37445951098919E-32,1.,1.83697019872104E-16));
#141686=DIRECTION('center_axis',(0.,0.,-1.));
#141687=DIRECTION('ref_axis',(1.,0.,0.));
#141688=DIRECTION('center_axis',(-1.83697019872103E-16,1.83697019872104E-16,
-1.));
#141689=DIRECTION('ref_axis',(3.85494105772625E-15,1.,1.83697019872103E-16));
#141690=DIRECTION('',(-1.83697019872103E-16,1.83697019872104E-16,-1.));
#141691=DIRECTION('center_axis',(-0.70710678118655,-0.707106781186545,4.36149058175079E-31));
#141692=DIRECTION('ref_axis',(0.707106781186545,-0.70710678118655,2.77480222991945E-47));
#141693=DIRECTION('',(-0.707106781186545,0.70710678118655,0.));
#141694=DIRECTION('',(-0.707106781186545,0.70710678118655,2.59786816870648E-16));
#141695=DIRECTION('',(-1.83697019872103E-16,1.83697019872104E-16,-1.));
#141696=DIRECTION('center_axis',(-1.83697019872103E-16,1.83697019872104E-16,
-1.));
#141697=DIRECTION('ref_axis',(3.37445951098919E-32,1.,1.83697019872104E-16));
#141698=DIRECTION('center_axis',(0.,0.,-1.));
#141699=DIRECTION('ref_axis',(1.,0.,0.));
#141700=DIRECTION('center_axis',(-1.83697019872103E-16,1.83697019872104E-16,
-1.));
#141701=DIRECTION('ref_axis',(3.85494105772625E-15,1.,1.83697019872103E-16));
#141702=DIRECTION('',(-1.83697019872103E-16,1.83697019872104E-16,-1.));
#141703=DIRECTION('center_axis',(-1.,1.81956044947143E-15,1.83697019872103E-16));
#141704=DIRECTION('ref_axis',(-1.81956044947143E-15,-1.,1.5521017945049E-47));
#141705=DIRECTION('',(1.81956044947143E-15,1.,0.));
#141706=DIRECTION('',(1.81956044947143E-15,1.,1.83697019872103E-16));
#141707=DIRECTION('',(-1.83697019872103E-16,1.83697019872104E-16,-1.));
#141708=DIRECTION('center_axis',(-1.83697019872103E-16,1.83697019872104E-16,
-1.));
#141709=DIRECTION('ref_axis',(3.37445951098919E-32,1.,1.83697019872104E-16));
#141710=DIRECTION('center_axis',(0.,0.,-1.));
#141711=DIRECTION('ref_axis',(1.,0.,0.));
#141712=DIRECTION('center_axis',(-1.83697019872103E-16,1.83697019872104E-16,
-1.));
#141713=DIRECTION('ref_axis',(3.85494105772625E-15,1.,1.83697019872103E-16));
#141714=DIRECTION('',(-1.83697019872103E-16,1.83697019872104E-16,-1.));
#141715=DIRECTION('center_axis',(1.35643706071783E-15,1.,1.83697019872103E-16));
#141716=DIRECTION('ref_axis',(-1.,1.35643706071783E-15,0.));
#141717=DIRECTION('',(1.,-1.35643706071783E-15,0.));
#141718=DIRECTION('',(1.,-1.35643706071783E-15,-1.83697019872103E-16));
#141719=DIRECTION('',(-1.83697019872103E-16,1.83697019872104E-16,-1.));
#141720=DIRECTION('center_axis',(-1.83697019872103E-16,1.83697019872104E-16,
-1.));
#141721=DIRECTION('ref_axis',(3.37445951098919E-32,1.,1.83697019872104E-16));
#141722=DIRECTION('center_axis',(0.,0.,1.));
#141723=DIRECTION('ref_axis',(1.,0.,0.));
#141724=DIRECTION('center_axis',(1.83697019872103E-16,-1.83697019872104E-16,
1.));
#141725=DIRECTION('ref_axis',(3.85494105772628E-15,1.,1.83697019872103E-16));
#141726=DIRECTION('',(-1.83697019872103E-16,1.83697019872104E-16,-1.));
#141727=DIRECTION('center_axis',(-1.,4.74570945839986E-16,1.83697019872103E-16));
#141728=DIRECTION('ref_axis',(-4.74570945839986E-16,-1.,-8.94815989765196E-49));
#141729=DIRECTION('',(4.74570945839986E-16,1.,0.));
#141730=DIRECTION('',(4.74570945839986E-16,1.,1.83697019872104E-16));
#141731=DIRECTION('',(-1.83697019872103E-16,1.83697019872104E-16,-1.));
#141732=DIRECTION('center_axis',(-3.49148133884313E-15,-1.,-1.83697019872103E-16));
#141733=DIRECTION('ref_axis',(1.,-3.49148133884313E-15,0.));
#141734=DIRECTION('',(-1.,3.49148133884313E-15,0.));
#141735=DIRECTION('',(-1.,3.49148133884313E-15,1.83697019872104E-16));
#141736=DIRECTION('',(-1.83697019872103E-16,1.83697019872104E-16,-1.));
#141737=DIRECTION('center_axis',(-1.,3.49148133884313E-15,1.83697019872104E-16));
#141738=DIRECTION('ref_axis',(-3.49148133884313E-15,-1.,1.78914547131776E-47));
#141739=DIRECTION('',(3.49148133884313E-15,1.,0.));
#141740=DIRECTION('',(3.49148133884313E-15,1.,1.83697019872103E-16));
#141741=DIRECTION('center_axis',(-1.,1.07955801850613E-14,1.83697019872105E-16));
#141742=DIRECTION('ref_axis',(-1.07955801850613E-14,-1.,-1.3652856201189E-46));
#141743=DIRECTION('',(1.07955801850613E-14,1.,0.));
#141744=DIRECTION('',(0.,3.67394039744206E-16,-1.));
#141745=DIRECTION('',(1.07955801850613E-14,1.,1.83697019872102E-16));
#141746=DIRECTION('',(-1.83697019872103E-16,1.83697019872104E-16,-1.));
#141747=DIRECTION('center_axis',(-1.61076520732197E-14,-1.,-1.83697019872101E-16));
#141748=DIRECTION('ref_axis',(1.,-1.61076520732197E-14,0.));
#141749=DIRECTION('',(-1.,1.61076520732197E-14,0.));
#141750=DIRECTION('',(-1.,1.61076520732197E-14,1.83697019872106E-16));
#141751=DIRECTION('',(-1.83697019872103E-16,1.83697019872104E-16,-1.));
#141752=DIRECTION('center_axis',(-1.,9.79956670603158E-15,1.83697019872105E-16));
#141753=DIRECTION('ref_axis',(-9.79956670603158E-15,-1.,1.22009766052885E-46));
#141754=DIRECTION('',(9.79956670603158E-15,1.,0.));
#141755=DIRECTION('',(9.79956670603158E-15,1.,1.83697019872102E-16));
#141756=DIRECTION('',(-1.83697019872103E-16,1.83697019872104E-16,-1.));
#141757=DIRECTION('center_axis',(-1.25422125178526E-14,-1.,-1.83697019872101E-16));
#141758=DIRECTION('ref_axis',(1.,-1.25422125178526E-14,0.));
#141759=DIRECTION('',(-1.,1.25422125178526E-14,0.));
#141760=DIRECTION('',(-1.,1.25422125178526E-14,1.83697019872105E-16));
#141761=DIRECTION('',(-1.83697019872103E-16,1.83697019872104E-16,-1.));
#141762=DIRECTION('center_axis',(-1.83697019872103E-16,1.83697019872104E-16,
-1.));
#141763=DIRECTION('ref_axis',(3.37445951098919E-32,1.,1.83697019872104E-16));
#141764=DIRECTION('center_axis',(0.,0.,1.));
#141765=DIRECTION('ref_axis',(1.,0.,0.));
#141766=DIRECTION('center_axis',(1.83697019872103E-16,-1.83697019872104E-16,
1.));
#141767=DIRECTION('ref_axis',(-3.37445951098919E-32,-1.,-1.83697019872104E-16));
#141768=DIRECTION('',(-1.83697019872103E-16,1.83697019872104E-16,-1.));
#141769=DIRECTION('center_axis',(1.,-1.20316584513443E-14,-1.83697019872105E-16));
#141770=DIRECTION('ref_axis',(1.20316584513443E-14,1.,1.32485337866494E-46));
#141771=DIRECTION('',(-1.20316584513443E-14,-1.,0.));
#141772=DIRECTION('',(-1.20316584513443E-14,-1.,-1.83697019872101E-16));
#141773=DIRECTION('',(-1.83697019872103E-16,1.83697019872104E-16,-1.));
#141774=DIRECTION('center_axis',(-1.83697019872103E-16,1.83697019872104E-16,
-1.));
#141775=DIRECTION('ref_axis',(3.37445951098919E-32,1.,1.83697019872104E-16));
#141776=DIRECTION('center_axis',(0.,0.,-1.));
#141777=DIRECTION('ref_axis',(1.,-1.15648231731787E-14,0.));
#141778=DIRECTION('center_axis',(-1.83697019872103E-16,1.83697019872104E-16,
-1.));
#141779=DIRECTION('ref_axis',(-3.37445951098919E-32,-1.,-1.83697019872104E-16));
#141780=DIRECTION('',(-1.83697019872103E-16,1.83697019872104E-16,-1.));
#141781=DIRECTION('center_axis',(-1.18510857857016E-14,-1.,-1.83697019872101E-16));
#141782=DIRECTION('ref_axis',(1.,-1.18510857857016E-14,0.));
#141783=DIRECTION('',(-1.,1.18510857857016E-14,0.));
#141784=DIRECTION('',(-1.,1.18510857857016E-14,1.83697019872105E-16));
#141785=DIRECTION('',(-1.83697019872103E-16,1.83697019872104E-16,-1.));
#141786=DIRECTION('center_axis',(-1.83697019872103E-16,1.83697019872104E-16,
-1.));
#141787=DIRECTION('ref_axis',(3.37445951098919E-32,1.,1.83697019872104E-16));
#141788=DIRECTION('center_axis',(0.,0.,-1.));
#141789=DIRECTION('ref_axis',(1.,-1.92747052886312E-15,0.));
#141790=DIRECTION('center_axis',(-1.83697019872103E-16,1.83697019872104E-16,
-1.));
#141791=DIRECTION('ref_axis',(-3.37445951098919E-32,-1.,-1.83697019872104E-16));
#141792=DIRECTION('',(-1.83697019872103E-16,1.83697019872104E-16,-1.));
#141793=DIRECTION('center_axis',(-0.707106781186555,-0.70710678118654,2.38933831869826E-30));
#141794=DIRECTION('ref_axis',(0.70710678118654,-0.707106781186555,2.91705557987951E-47));
#141795=DIRECTION('',(-0.70710678118654,0.707106781186555,0.));
#141796=DIRECTION('',(-0.70710678118654,0.707106781186555,2.59786816870648E-16));
#141797=DIRECTION('',(-1.83697019872103E-16,1.83697019872104E-16,-1.));
#141798=DIRECTION('center_axis',(-1.83697019872103E-16,1.83697019872104E-16,
-1.));
#141799=DIRECTION('ref_axis',(3.37445951098919E-32,1.,1.83697019872104E-16));
#141800=DIRECTION('center_axis',(0.,0.,-1.));
#141801=DIRECTION('ref_axis',(1.,-1.15648231731787E-14,0.));
#141802=DIRECTION('center_axis',(-1.83697019872103E-16,1.83697019872104E-16,
-1.));
#141803=DIRECTION('ref_axis',(-3.37445951098919E-32,-1.,-1.83697019872104E-16));
#141804=DIRECTION('',(-1.83697019872103E-16,1.83697019872104E-16,-1.));
#141805=DIRECTION('center_axis',(-1.,1.22199641292386E-14,1.83697019872105E-16));
#141806=DIRECTION('ref_axis',(-1.22199641292386E-14,-1.,1.88282412675184E-47));
#141807=DIRECTION('',(1.22199641292386E-14,1.,0.));
#141808=DIRECTION('',(1.22199641292386E-14,1.,1.83697019872101E-16));
#141809=DIRECTION('',(-1.83697019872103E-16,1.83697019872104E-16,-1.));
#141810=DIRECTION('center_axis',(-0.866025403784453,-0.499999999999976,
6.72377758726913E-17));
#141811=DIRECTION('ref_axis',(0.499999999999976,-0.866025403784453,-1.39433958635012E-33));
#141812=DIRECTION('',(-0.499999999999976,0.866025403784453,0.));
#141813=DIRECTION('',(-0.499999999999976,0.866025403784453,2.50934795744786E-16));
#141814=DIRECTION('',(-1.83697019872103E-16,1.83697019872104E-16,-1.));
#141815=DIRECTION('center_axis',(-0.866025403784435,0.500000000000007,2.50934795744788E-16));
#141816=DIRECTION('ref_axis',(-0.500000000000007,-0.866025403784435,3.9034319157649E-33));
#141817=DIRECTION('',(0.500000000000007,0.866025403784435,0.));
#141818=DIRECTION('',(0.500000000000007,0.866025403784435,6.72377758726831E-17));
#141819=DIRECTION('',(-1.83697019872103E-16,1.83697019872104E-16,-1.));
#141820=DIRECTION('center_axis',(-1.,3.49148133884313E-15,1.83697019872104E-16));
#141821=DIRECTION('ref_axis',(-3.49148133884313E-15,-1.,1.78914547131776E-47));
#141822=DIRECTION('',(3.49148133884313E-15,1.,0.));
#141823=DIRECTION('',(3.49148133884313E-15,1.,1.83697019872103E-16));
#141824=DIRECTION('',(-1.83697019872103E-16,1.83697019872104E-16,-1.));
#141825=DIRECTION('center_axis',(-1.83697019872103E-16,1.83697019872104E-16,
-1.));
#141826=DIRECTION('ref_axis',(3.37445951098919E-32,1.,1.83697019872104E-16));
#141827=DIRECTION('center_axis',(0.,0.,-1.));
#141828=DIRECTION('ref_axis',(1.,-2.31296463463575E-14,0.));
#141829=DIRECTION('center_axis',(-1.83697019872103E-16,1.83697019872104E-16,
-1.));
#141830=DIRECTION('ref_axis',(-3.37445951098919E-32,-1.,-1.83697019872104E-16));
#141831=DIRECTION('',(-1.83697019872103E-16,1.83697019872104E-16,-1.));
#141832=DIRECTION('center_axis',(-0.707106781186545,0.70710678118655,2.59786816870649E-16));
#141833=DIRECTION('ref_axis',(-0.70710678118655,-0.707106781186545,-1.41173070057919E-32));
#141834=DIRECTION('',(0.70710678118655,0.707106781186545,0.));
#141835=DIRECTION('',(0.70710678118655,0.707106781186545,-4.68386162474976E-31));
#141836=DIRECTION('',(-1.83697019872103E-16,1.83697019872104E-16,-1.));
#141837=DIRECTION('center_axis',(-1.83697019872103E-16,1.83697019872104E-16,
-1.));
#141838=DIRECTION('ref_axis',(3.37445951098919E-32,1.,1.83697019872104E-16));
#141839=DIRECTION('center_axis',(0.,0.,-1.));
#141840=DIRECTION('ref_axis',(1.,0.,0.));
#141841=DIRECTION('center_axis',(-1.83697019872103E-16,1.83697019872104E-16,
-1.));
#141842=DIRECTION('ref_axis',(-3.37445951098919E-32,-1.,-1.83697019872104E-16));
#141843=DIRECTION('',(-1.83697019872103E-16,1.83697019872104E-16,-1.));
#141844=DIRECTION('center_axis',(3.49148133884313E-15,1.,1.83697019872103E-16));
#141845=DIRECTION('ref_axis',(-1.,3.49148133884313E-15,0.));
#141846=DIRECTION('',(1.,-3.49148133884313E-15,0.));
#141847=DIRECTION('',(1.,-3.49148133884313E-15,-1.83697019872104E-16));
#141848=DIRECTION('',(-1.83697019872103E-16,1.83697019872104E-16,-1.));
#141849=DIRECTION('center_axis',(-1.83697019872103E-16,1.83697019872104E-16,
-1.));
#141850=DIRECTION('ref_axis',(3.37445951098919E-32,1.,1.83697019872104E-16));
#141851=DIRECTION('center_axis',(0.,0.,-1.));
#141852=DIRECTION('ref_axis',(1.,2.31296463463577E-14,0.));
#141853=DIRECTION('center_axis',(-1.83697019872103E-16,1.83697019872104E-16,
-1.));
#141854=DIRECTION('ref_axis',(-3.37445951098919E-32,-1.,-1.83697019872104E-16));
#141855=DIRECTION('',(-1.83697019872103E-16,1.83697019872104E-16,-1.));
#141856=DIRECTION('center_axis',(1.,-1.35643706071783E-15,-1.83697019872103E-16));
#141857=DIRECTION('ref_axis',(1.35643706071783E-15,1.,8.4478697733554E-48));
#141858=DIRECTION('',(-1.35643706071783E-15,-1.,0.));
#141859=DIRECTION('',(-1.35643706071783E-15,-1.,-1.83697019872103E-16));
#141860=DIRECTION('',(-1.83697019872103E-16,1.83697019872104E-16,-1.));
#141861=DIRECTION('center_axis',(-1.83697019872103E-16,1.83697019872104E-16,
-1.));
#141862=DIRECTION('ref_axis',(3.37445951098919E-32,1.,1.83697019872104E-16));
#141863=DIRECTION('center_axis',(0.,0.,1.));
#141864=DIRECTION('ref_axis',(1.,0.,0.));
#141865=DIRECTION('center_axis',(1.83697019872103E-16,-1.83697019872104E-16,
1.));
#141866=DIRECTION('ref_axis',(-3.37445951098919E-32,-1.,-1.83697019872104E-16));
#141867=DIRECTION('',(-1.83697019872103E-16,1.83697019872104E-16,-1.));
#141868=DIRECTION('center_axis',(3.49148133884313E-15,1.,1.83697019872103E-16));
#141869=DIRECTION('ref_axis',(-1.,3.49148133884313E-15,0.));
#141870=DIRECTION('',(1.,-3.49148133884313E-15,0.));
#141871=DIRECTION('',(1.,-3.49148133884313E-15,-1.83697019872104E-16));
#141872=DIRECTION('',(-1.83697019872103E-16,1.83697019872104E-16,-1.));
#141873=DIRECTION('center_axis',(-1.,3.49148133884313E-15,1.83697019872104E-16));
#141874=DIRECTION('ref_axis',(-3.49148133884313E-15,-1.,1.78914547131776E-47));
#141875=DIRECTION('',(3.49148133884313E-15,1.,0.));
#141876=DIRECTION('',(3.49148133884313E-15,1.,1.83697019872103E-16));
#141877=DIRECTION('',(-1.83697019872103E-16,1.83697019872104E-16,-1.));
#141878=DIRECTION('center_axis',(3.49148133884313E-15,1.,1.83697019872103E-16));
#141879=DIRECTION('ref_axis',(-1.,3.49148133884313E-15,0.));
#141880=DIRECTION('',(1.,-3.49148133884313E-15,0.));
#141881=DIRECTION('',(1.,-3.49148133884313E-15,-1.83697019872104E-16));
#141882=DIRECTION('',(-1.83697019872103E-16,1.83697019872104E-16,-1.));
#141883=DIRECTION('center_axis',(-1.,3.49148133884313E-15,1.83697019872104E-16));
#141884=DIRECTION('ref_axis',(-3.49148133884313E-15,-1.,1.78914547131776E-47));
#141885=DIRECTION('',(3.49148133884313E-15,1.,0.));
#141886=DIRECTION('',(3.49148133884313E-15,1.,1.83697019872103E-16));
#141887=DIRECTION('',(-1.83697019872103E-16,1.83697019872104E-16,-1.));
#141888=DIRECTION('center_axis',(-1.83697019872103E-16,1.83697019872104E-16,
-1.));
#141889=DIRECTION('ref_axis',(3.37445951098919E-32,1.,1.83697019872104E-16));
#141890=DIRECTION('center_axis',(0.,0.,1.));
#141891=DIRECTION('ref_axis',(1.,0.,0.));
#141892=DIRECTION('center_axis',(1.83697019872103E-16,-1.83697019872104E-16,
1.));
#141893=DIRECTION('ref_axis',(-3.79423332453363E-15,-1.,-1.83697019872103E-16));
#141894=DIRECTION('',(-1.83697019872103E-16,1.83697019872104E-16,-1.));
#141895=DIRECTION('center_axis',(-3.90362756739548E-15,-1.,-1.83697019872103E-16));
#141896=DIRECTION('ref_axis',(1.,-3.90362756739548E-15,0.));
#141897=DIRECTION('',(-1.,3.90362756739548E-15,0.));
#141898=DIRECTION('',(-1.,3.90362756739548E-15,1.83697019872104E-16));
#141899=DIRECTION('',(-1.83697019872103E-16,1.83697019872104E-16,-1.));
#141900=DIRECTION('center_axis',(1.,-3.49148133884313E-15,-1.83697019872104E-16));
#141901=DIRECTION('ref_axis',(3.49148133884313E-15,1.,-1.78914547131776E-47));
#141902=DIRECTION('',(-3.49148133884313E-15,-1.,0.));
#141903=DIRECTION('',(-3.49148133884313E-15,-1.,-1.83697019872103E-16));
#141904=DIRECTION('',(-1.83697019872103E-16,1.83697019872104E-16,-1.));
#141905=DIRECTION('center_axis',(-3.49148133884313E-15,-1.,-1.83697019872103E-16));
#141906=DIRECTION('ref_axis',(1.,-3.49148133884313E-15,0.));
#141907=DIRECTION('',(-1.,3.49148133884313E-15,0.));
#141908=DIRECTION('',(-1.,3.49148133884313E-15,1.83697019872104E-16));
#141909=DIRECTION('',(-1.83697019872103E-16,1.83697019872104E-16,-1.));
#141910=DIRECTION('center_axis',(1.,-6.50839173184628E-15,-1.83697019872104E-16));
#141911=DIRECTION('ref_axis',(6.50839173184628E-15,1.,-4.21210294408139E-47));
#141912=DIRECTION('',(-6.50839173184628E-15,-1.,0.));
#141913=DIRECTION('',(-6.50839173184628E-15,-1.,-1.83697019872102E-16));
#141914=DIRECTION('',(-1.83697019872103E-16,1.83697019872104E-16,-1.));
#141915=DIRECTION('center_axis',(-1.83697019872103E-16,1.83697019872104E-16,
-1.));
#141916=DIRECTION('ref_axis',(3.37445951098919E-32,1.,1.83697019872104E-16));
#141917=DIRECTION('center_axis',(0.,0.,1.));
#141918=DIRECTION('ref_axis',(1.,0.,0.));
#141919=DIRECTION('center_axis',(1.83697019872103E-16,-1.83697019872104E-16,
1.));
#141920=DIRECTION('ref_axis',(-3.37445951098919E-32,-1.,-1.83697019872104E-16));
#141921=DIRECTION('',(-1.83697019872103E-16,1.83697019872104E-16,-1.));
#141922=DIRECTION('center_axis',(5.62652561696843E-15,1.,1.83697019872103E-16));
#141923=DIRECTION('ref_axis',(-1.,5.62652561696843E-15,0.));
#141924=DIRECTION('',(1.,-5.62652561696843E-15,0.));
#141925=DIRECTION('',(1.,-5.62652561696843E-15,-1.83697019872104E-16));
#141926=DIRECTION('',(-1.83697019872103E-16,1.83697019872104E-16,-1.));
#141927=DIRECTION('center_axis',(-1.83697019872103E-16,1.83697019872104E-16,
-1.));
#141928=DIRECTION('ref_axis',(3.37445951098919E-32,1.,1.83697019872104E-16));
#141929=DIRECTION('center_axis',(0.,0.,-1.));
#141930=DIRECTION('ref_axis',(1.,2.31296463463575E-14,0.));
#141931=DIRECTION('center_axis',(-1.83697019872103E-16,1.83697019872104E-16,
-1.));
#141932=DIRECTION('ref_axis',(-3.37445951098919E-32,-1.,-1.83697019872104E-16));
#141933=DIRECTION('',(-1.83697019872103E-16,1.83697019872104E-16,-1.));
#141934=DIRECTION('center_axis',(1.,-5.16340222821484E-15,-1.83697019872104E-16));
#141935=DIRECTION('ref_axis',(5.16340222821484E-15,1.,8.5317764086697E-47));
#141936=DIRECTION('',(-5.16340222821484E-15,-1.,0.));
#141937=DIRECTION('',(-5.16340222821484E-15,-1.,-1.83697019872103E-16));
#141938=DIRECTION('',(-1.83697019872103E-16,1.83697019872104E-16,-1.));
#141939=DIRECTION('center_axis',(-1.83697019872103E-16,1.83697019872104E-16,
-1.));
#141940=DIRECTION('ref_axis',(3.37445951098919E-32,1.,1.83697019872104E-16));
#141941=DIRECTION('center_axis',(0.,0.,-1.));
#141942=DIRECTION('ref_axis',(1.,0.,0.));
#141943=DIRECTION('center_axis',(-1.83697019872103E-16,1.83697019872104E-16,
-1.));
#141944=DIRECTION('ref_axis',(-3.37445951098919E-32,-1.,-1.83697019872104E-16));
#141945=DIRECTION('',(-1.83697019872103E-16,1.83697019872104E-16,-1.));
#141946=DIRECTION('center_axis',(0.707106781186545,-0.70710678118655,-2.59786816870649E-16));
#141947=DIRECTION('ref_axis',(0.70710678118655,0.707106781186545,1.41173070057919E-32));
#141948=DIRECTION('',(-0.70710678118655,-0.707106781186545,0.));
#141949=DIRECTION('',(-0.70710678118655,-0.707106781186545,4.68386162474976E-31));
#141950=DIRECTION('',(-1.83697019872103E-16,1.83697019872104E-16,-1.));
#141951=DIRECTION('center_axis',(-1.83697019872103E-16,1.83697019872104E-16,
-1.));
#141952=DIRECTION('ref_axis',(3.37445951098919E-32,1.,1.83697019872104E-16));
#141953=DIRECTION('center_axis',(0.,0.,-1.));
#141954=DIRECTION('ref_axis',(1.,7.70988211545249E-15,0.));
#141955=DIRECTION('center_axis',(-1.83697019872103E-16,1.83697019872104E-16,
-1.));
#141956=DIRECTION('ref_axis',(-3.37445951098919E-32,-1.,-1.83697019872104E-16));
#141957=DIRECTION('',(-1.83697019872103E-16,1.83697019872104E-16,-1.));
#141958=DIRECTION('center_axis',(-3.49148133884313E-15,-1.,-1.83697019872103E-16));
#141959=DIRECTION('ref_axis',(1.,-3.49148133884313E-15,0.));
#141960=DIRECTION('',(-1.,3.49148133884313E-15,0.));
#141961=DIRECTION('',(-1.,3.49148133884313E-15,1.83697019872104E-16));
#141962=DIRECTION('center_axis',(-0.866025403784438,-0.500000000000001,
-1.83697019872103E-16));
#141963=DIRECTION('ref_axis',(0.500000000000001,-0.866025403784438,2.0289671949304E-33));
#141964=DIRECTION('',(-0.5,0.866025403784438,0.));
#141965=DIRECTION('',(0.,3.67394039744206E-16,-1.));
#141966=DIRECTION('',(-0.5,0.866025403784438,3.18172571617472E-16));
#141967=DIRECTION('',(0.,3.67394039744206E-16,-1.));
#141968=DIRECTION('center_axis',(-0.866025403784438,0.500000000000002,1.83697019872104E-16));
#141969=DIRECTION('ref_axis',(-0.500000000000002,-0.866025403784437,9.7694722305658E-33));
#141970=DIRECTION('',(0.500000000000002,0.866025403784438,0.));
#141971=DIRECTION('',(0.500000000000002,0.866025403784438,3.18172571617472E-16));
#141972=DIRECTION('',(0.,3.67394039744206E-16,-1.));
#141973=DIRECTION('center_axis',(-1.,0.,0.));
#141974=DIRECTION('ref_axis',(0.,0.,1.));
#141975=DIRECTION('',(0.,1.,0.));
#141976=DIRECTION('',(0.,1.,3.67394039744206E-16));
#141977=DIRECTION('',(0.,3.67394039744206E-16,-1.));
#141978=DIRECTION('center_axis',(0.,3.67394039744206E-16,-1.));
#141979=DIRECTION('ref_axis',(0.,1.,3.67394039744206E-16));
#141980=DIRECTION('center_axis',(0.,0.,-1.));
#141981=DIRECTION('ref_axis',(1.,1.15648231731787E-14,0.));
#141982=DIRECTION('center_axis',(0.,3.67394039744206E-16,-1.));
#141983=DIRECTION('ref_axis',(1.,0.,0.));
#141984=DIRECTION('',(0.,3.67394039744206E-16,-1.));
#141985=DIRECTION('center_axis',(-0.707106781186548,0.707106781186548,2.59786816870648E-16));
#141986=DIRECTION('ref_axis',(-0.707106781186548,-0.707106781186548,1.22182752772918E-34));
#141987=DIRECTION('',(0.707106781186547,0.707106781186547,0.));
#141988=DIRECTION('',(0.707106781186547,0.707106781186547,2.59786816870648E-16));
#141989=DIRECTION('',(0.,3.67394039744206E-16,-1.));
#141990=DIRECTION('center_axis',(0.,3.67394039744206E-16,-1.));
#141991=DIRECTION('ref_axis',(0.,1.,3.67394039744206E-16));
#141992=DIRECTION('center_axis',(0.,0.,-1.));
#141993=DIRECTION('ref_axis',(1.,-7.70988211545249E-15,0.));
#141994=DIRECTION('center_axis',(0.,3.67394039744206E-16,-1.));
#141995=DIRECTION('ref_axis',(1.,0.,0.));
#141996=DIRECTION('',(0.,3.67394039744206E-16,-1.));
#141997=DIRECTION('center_axis',(-1.6719208893717E-15,1.,3.67394039744206E-16));
#141998=DIRECTION('ref_axis',(-1.,-1.6719208893717E-15,0.));
#141999=DIRECTION('',(1.,1.6719208893717E-15,0.));
#142000=DIRECTION('',(1.,1.6719208893717E-15,6.14253769678996E-31));
#142001=DIRECTION('',(0.,3.67394039744206E-16,-1.));
#142002=DIRECTION('center_axis',(0.,3.67394039744206E-16,-1.));
#142003=DIRECTION('ref_axis',(0.,1.,3.67394039744206E-16));
#142004=DIRECTION('center_axis',(0.,0.,-1.));
#142005=DIRECTION('ref_axis',(1.,0.,0.));
#142006=DIRECTION('center_axis',(0.,3.67394039744206E-16,-1.));
#142007=DIRECTION('ref_axis',(1.,0.,0.));
#142008=DIRECTION('',(0.,3.67394039744206E-16,-1.));
#142009=DIRECTION('center_axis',(1.,2.1350442781253E-15,7.84402542373206E-31));
#142010=DIRECTION('ref_axis',(-2.1350442781253E-15,1.,5.68845695218989E-62));
#142011=DIRECTION('',(2.1350442781253E-15,-1.,0.));
#142012=DIRECTION('',(2.1350442781253E-15,-1.,-3.67394039744206E-16));
#142013=DIRECTION('',(0.,3.67394039744206E-16,-1.));
#142014=DIRECTION('center_axis',(0.,3.67394039744206E-16,-1.));
#142015=DIRECTION('ref_axis',(0.,1.,3.67394039744206E-16));
#142016=DIRECTION('center_axis',(0.,0.,1.));
#142017=DIRECTION('ref_axis',(1.,0.,0.));
#142018=DIRECTION('center_axis',(0.,-3.67394039744206E-16,1.));
#142019=DIRECTION('ref_axis',(1.,0.,0.));
#142020=DIRECTION('',(0.,3.67394039744206E-16,-1.));
#142021=DIRECTION('center_axis',(-3.01691039300315E-15,1.,3.67394039744206E-16));
#142022=DIRECTION('ref_axis',(-1.,-3.01691039300315E-15,0.));
#142023=DIRECTION('',(1.,3.01691039300315E-15,0.));
#142024=DIRECTION('',(1.,3.01691039300315E-15,1.10839489683171E-30));
#142025=DIRECTION('',(0.,3.67394039744206E-16,-1.));
#142026=DIRECTION('center_axis',(-1.,0.,0.));
#142027=DIRECTION('ref_axis',(0.,0.,1.));
#142028=DIRECTION('',(0.,1.,0.));
#142029=DIRECTION('',(0.,1.,3.67394039744206E-16));
#142030=DIRECTION('',(0.,3.67394039744206E-16,-1.));
#142031=DIRECTION('center_axis',(0.,1.,3.67394039744206E-16));
#142032=DIRECTION('ref_axis',(0.,-3.67394039744206E-16,1.));
#142033=DIRECTION('',(1.,0.,0.));
#142034=DIRECTION('',(1.,0.,0.));
#142035=DIRECTION('center_axis',(7.30409884621813E-15,1.,3.67394039744206E-16));
#142036=DIRECTION('ref_axis',(-1.,7.30409884621813E-15,0.));
#142037=DIRECTION('',(1.,-7.30409884621813E-15,0.));
#142038=DIRECTION('',(1.83697019872103E-16,1.83697019872101E-16,-1.));
#142039=DIRECTION('',(1.,-7.30409884621813E-15,-2.68348238180307E-30));
#142040=DIRECTION('',(0.,3.67394039744206E-16,-1.));
#142041=DIRECTION('center_axis',(-1.,1.26161707343766E-14,4.63510593220524E-30));
#142042=DIRECTION('ref_axis',(-1.26161707343766E-14,-1.,-3.84512883862554E-60));
#142043=DIRECTION('',(1.26161707343766E-14,1.,0.));
#142044=DIRECTION('',(1.26161707343766E-14,1.,3.67394039744206E-16));
#142045=DIRECTION('',(0.,3.67394039744206E-16,-1.));
#142046=DIRECTION('center_axis',(6.30808536718845E-15,1.,3.67394039744206E-16));
#142047=DIRECTION('ref_axis',(-1.,6.30808536718845E-15,0.));
#142048=DIRECTION('',(1.,-6.30808536718845E-15,0.));
#142049=DIRECTION('',(1.,-6.30808536718845E-15,-2.31755296610268E-30));
#142050=DIRECTION('',(0.,3.67394039744206E-16,-1.));
#142051=DIRECTION('center_axis',(-1.,9.05073117900944E-15,3.32518469049512E-30));
#142052=DIRECTION('ref_axis',(-9.05073117900944E-15,-1.,1.73421017874153E-60));
#142053=DIRECTION('',(9.05073117900944E-15,1.,0.));
#142054=DIRECTION('',(9.05073117900944E-15,1.,3.67394039744206E-16));
#142055=DIRECTION('',(0.,3.67394039744206E-16,-1.));
#142056=DIRECTION('center_axis',(0.,3.67394039744206E-16,-1.));
#142057=DIRECTION('ref_axis',(0.,1.,3.67394039744206E-16));
#142058=DIRECTION('center_axis',(0.,0.,1.));
#142059=DIRECTION('ref_axis',(1.,0.,0.));
#142060=DIRECTION('center_axis',(0.,-3.67394039744206E-16,1.));
#142061=DIRECTION('ref_axis',(-1.,0.,0.));
#142062=DIRECTION('',(0.,3.67394039744206E-16,-1.));
#142063=DIRECTION('center_axis',(-8.5401771125012E-15,-1.,-3.67394039744206E-16));
#142064=DIRECTION('ref_axis',(1.,-8.5401771125012E-15,0.));
#142065=DIRECTION('',(-1.,8.5401771125012E-15,0.));
#142066=DIRECTION('',(-1.,8.5401771125012E-15,3.13761016949282E-30));
#142067=DIRECTION('',(0.,3.67394039744206E-16,-1.));
#142068=DIRECTION('center_axis',(0.,3.67394039744206E-16,-1.));
#142069=DIRECTION('ref_axis',(0.,1.,3.67394039744206E-16));
#142070=DIRECTION('center_axis',(0.,0.,-1.));
#142071=DIRECTION('ref_axis',(1.,0.,0.));
#142072=DIRECTION('center_axis',(0.,3.67394039744206E-16,-1.));
#142073=DIRECTION('ref_axis',(-1.,0.,0.));
#142074=DIRECTION('',(0.,3.67394039744206E-16,-1.));
#142075=DIRECTION('center_axis',(-1.,8.3596044468585E-15,3.07126884839497E-30));
#142076=DIRECTION('ref_axis',(-8.3596044468585E-15,-1.,-3.49500060354943E-61));
#142077=DIRECTION('',(8.3596044468585E-15,1.,0.));
#142078=DIRECTION('',(8.3596044468585E-15,1.,3.67394039744206E-16));
#142079=DIRECTION('',(0.,3.67394039744206E-16,-1.));
#142080=DIRECTION('center_axis',(0.,3.67394039744206E-16,-1.));
#142081=DIRECTION('ref_axis',(0.,1.,3.67394039744206E-16));
#142082=DIRECTION('center_axis',(0.,0.,-1.));
#142083=DIRECTION('ref_axis',(1.,7.70988211545251E-15,0.));
#142084=DIRECTION('center_axis',(0.,3.67394039744206E-16,-1.));
#142085=DIRECTION('ref_axis',(-1.,0.,0.));
#142086=DIRECTION('',(0.,3.67394039744206E-16,-1.));
#142087=DIRECTION('center_axis',(-0.707106781186542,0.707106781186553,2.5978681687065E-16));
#142088=DIRECTION('ref_axis',(-0.707106781186553,-0.707106781186542,-1.42399511956761E-32));
#142089=DIRECTION('',(0.707106781186553,0.707106781186542,0.));
#142090=DIRECTION('',(0.707106781186553,0.707106781186542,2.59786816870646E-16));
#142091=DIRECTION('',(0.,3.67394039744206E-16,-1.));
#142092=DIRECTION('center_axis',(0.,3.67394039744206E-16,-1.));
#142093=DIRECTION('ref_axis',(0.,1.,3.67394039744206E-16));
#142094=DIRECTION('center_axis',(0.,0.,-1.));
#142095=DIRECTION('ref_axis',(1.,-3.083952846181E-14,0.));
#142096=DIRECTION('center_axis',(0.,3.67394039744206E-16,-1.));
#142097=DIRECTION('ref_axis',(-1.,0.,0.));
#142098=DIRECTION('',(0.,3.67394039744206E-16,-1.));
#142099=DIRECTION('center_axis',(8.7284827903955E-15,1.,3.67394039744206E-16));
#142100=DIRECTION('ref_axis',(-1.,8.7284827903955E-15,0.));
#142101=DIRECTION('',(1.,-8.7284827903955E-15,0.));
#142102=DIRECTION('',(1.,-8.7284827903955E-15,-3.20679255320118E-30));
#142103=DIRECTION('',(0.,3.67394039744206E-16,-1.));
#142104=DIRECTION('center_axis',(-0.499999999999979,0.866025403784451,3.18172571617477E-16));
#142105=DIRECTION('ref_axis',(-0.866025403784451,-0.499999999999979,-4.69885821425642E-34));
#142106=DIRECTION('',(0.866025403784451,0.499999999999979,0.));
#142107=DIRECTION('',(0.866025403784451,0.499999999999979,1.83697019872095E-16));
#142108=DIRECTION('',(0.,3.67394039744206E-16,-1.));
#142109=DIRECTION('center_axis',(0.500000000000004,0.866025403784436,3.18172571617471E-16));
#142110=DIRECTION('ref_axis',(-0.866025403784436,0.500000000000004,-8.27337693045638E-33));
#142111=DIRECTION('',(0.866025403784436,-0.500000000000004,0.));
#142112=DIRECTION('',(0.866025403784436,-0.500000000000004,-1.83697019872104E-16));
#142113=DIRECTION('',(0.,3.67394039744206E-16,-1.));
#142114=DIRECTION('center_axis',(0.,1.,3.67394039744206E-16));
#142115=DIRECTION('ref_axis',(0.,-3.67394039744206E-16,1.));
#142116=DIRECTION('',(1.,0.,0.));
#142117=DIRECTION('',(1.,0.,0.));
#142118=DIRECTION('',(0.,3.67394039744206E-16,-1.));
#142119=DIRECTION('center_axis',(0.,3.67394039744206E-16,-1.));
#142120=DIRECTION('ref_axis',(0.,1.,3.67394039744206E-16));
#142121=DIRECTION('center_axis',(0.,0.,-1.));
#142122=DIRECTION('ref_axis',(1.,0.,0.));
#142123=DIRECTION('center_axis',(0.,3.67394039744206E-16,-1.));
#142124=DIRECTION('ref_axis',(-1.,0.,0.));
#142125=DIRECTION('',(0.,3.67394039744206E-16,-1.));
#142126=DIRECTION('center_axis',(0.707106781186548,0.707106781186548,2.59786816870648E-16));
#142127=DIRECTION('ref_axis',(-0.707106781186548,0.707106781186548,-1.22182752772918E-34));
#142128=DIRECTION('',(0.707106781186547,-0.707106781186547,0.));
#142129=DIRECTION('',(0.707106781186547,-0.707106781186547,-2.59786816870648E-16));
#142130=DIRECTION('',(0.,3.67394039744206E-16,-1.));
#142131=DIRECTION('center_axis',(0.,3.67394039744206E-16,-1.));
#142132=DIRECTION('ref_axis',(0.,1.,3.67394039744206E-16));
#142133=DIRECTION('center_axis',(0.,0.,-1.));
#142134=DIRECTION('ref_axis',(1.,0.,0.));
#142135=DIRECTION('center_axis',(0.,3.67394039744206E-16,-1.));
#142136=DIRECTION('ref_axis',(-1.,0.,0.));
#142137=DIRECTION('',(0.,3.67394039744206E-16,-1.));
#142138=DIRECTION('center_axis',(1.,0.,0.));
#142139=DIRECTION('ref_axis',(0.,0.,-1.));
#142140=DIRECTION('',(0.,-1.,0.));
#142141=DIRECTION('',(0.,-1.,-3.67394039744206E-16));
#142142=DIRECTION('',(0.,3.67394039744206E-16,-1.));
#142143=DIRECTION('center_axis',(0.,3.67394039744206E-16,-1.));
#142144=DIRECTION('ref_axis',(0.,1.,3.67394039744206E-16));
#142145=DIRECTION('center_axis',(0.,0.,-1.));
#142146=DIRECTION('ref_axis',(1.,0.,0.));
#142147=DIRECTION('center_axis',(0.,3.67394039744206E-16,-1.));
#142148=DIRECTION('ref_axis',(-1.,0.,0.));
#142149=DIRECTION('',(0.,3.67394039744206E-16,-1.));
#142150=DIRECTION('center_axis',(2.1350442781253E-15,-1.,-3.67394039744206E-16));
#142151=DIRECTION('ref_axis',(1.,2.1350442781253E-15,0.));
#142152=DIRECTION('',(-1.,-2.1350442781253E-15,0.));
#142153=DIRECTION('',(-1.,-2.1350442781253E-15,-7.84402542373207E-31));
#142154=DIRECTION('',(0.,3.67394039744206E-16,-1.));
#142155=DIRECTION('center_axis',(0.,3.67394039744206E-16,-1.));
#142156=DIRECTION('ref_axis',(0.,1.,3.67394039744206E-16));
#142157=DIRECTION('center_axis',(0.,0.,1.));
#142158=DIRECTION('ref_axis',(1.,0.,0.));
#142159=DIRECTION('center_axis',(0.,-3.67394039744206E-16,1.));
#142160=DIRECTION('ref_axis',(-1.,0.,0.));
#142161=DIRECTION('',(0.,3.67394039744206E-16,-1.));
#142162=DIRECTION('center_axis',(1.,0.,0.));
#142163=DIRECTION('ref_axis',(0.,0.,-1.));
#142164=DIRECTION('',(0.,-1.,0.));
#142165=DIRECTION('',(0.,-1.,-3.67394039744206E-16));
#142166=DIRECTION('',(0.,3.67394039744206E-16,-1.));
#142167=DIRECTION('center_axis',(0.,1.,3.67394039744206E-16));
#142168=DIRECTION('ref_axis',(0.,-3.67394039744206E-16,1.));
#142169=DIRECTION('',(1.,0.,0.));
#142170=DIRECTION('',(1.,0.,0.));
#142171=DIRECTION('',(0.,3.67394039744206E-16,-1.));
#142172=DIRECTION('center_axis',(1.,0.,0.));
#142173=DIRECTION('ref_axis',(0.,0.,-1.));
#142174=DIRECTION('',(0.,-1.,0.));
#142175=DIRECTION('',(0.,-1.,-3.67394039744206E-16));
#142176=DIRECTION('',(0.,3.67394039744206E-16,-1.));
#142177=DIRECTION('center_axis',(0.,1.,3.67394039744206E-16));
#142178=DIRECTION('ref_axis',(0.,-3.67394039744206E-16,1.));
#142179=DIRECTION('',(1.,0.,0.));
#142180=DIRECTION('',(1.,0.,0.));
#142181=DIRECTION('',(0.,3.67394039744206E-16,-1.));
#142182=DIRECTION('center_axis',(0.,3.67394039744206E-16,-1.));
#142183=DIRECTION('ref_axis',(0.,1.,3.67394039744206E-16));
#142184=DIRECTION('center_axis',(0.,0.,1.));
#142185=DIRECTION('ref_axis',(1.,0.,0.));
#142186=DIRECTION('center_axis',(0.,-3.67394039744206E-16,1.));
#142187=DIRECTION('ref_axis',(-1.,0.,0.));
#142188=DIRECTION('',(0.,3.67394039744206E-16,-1.));
#142189=DIRECTION('center_axis',(-1.,4.12146228552343E-16,1.51420067873184E-31));
#142190=DIRECTION('ref_axis',(-4.12146228552343E-16,-1.,5.13958017849863E-64));
#142191=DIRECTION('',(4.12146228552343E-16,1.,0.));
#142192=DIRECTION('',(4.12146228552343E-16,1.,3.67394039744206E-16));
#142193=DIRECTION('',(0.,3.67394039744206E-16,-1.));
#142194=DIRECTION('center_axis',(0.,-1.,-3.67394039744206E-16));
#142195=DIRECTION('ref_axis',(0.,3.67394039744206E-16,-1.));
#142196=DIRECTION('',(-1.,0.,0.));
#142197=DIRECTION('',(-1.,0.,0.));
#142198=DIRECTION('',(0.,3.67394039744206E-16,-1.));
#142199=DIRECTION('center_axis',(-1.,0.,0.));
#142200=DIRECTION('ref_axis',(0.,0.,1.));
#142201=DIRECTION('',(0.,1.,0.));
#142202=DIRECTION('',(0.,1.,3.67394039744206E-16));
#142203=DIRECTION('',(0.,3.67394039744206E-16,-1.));
#142204=DIRECTION('center_axis',(-3.01691039300315E-15,-1.,-3.67394039744206E-16));
#142205=DIRECTION('ref_axis',(1.,-3.01691039300315E-15,0.));
#142206=DIRECTION('',(-1.,3.01691039300315E-15,0.));
#142207=DIRECTION('',(-1.,3.01691039300315E-15,1.10839489683171E-30));
#142208=DIRECTION('',(0.,3.67394039744206E-16,-1.));
#142209=DIRECTION('center_axis',(0.,3.67394039744206E-16,-1.));
#142210=DIRECTION('ref_axis',(0.,1.,3.67394039744206E-16));
#142211=DIRECTION('center_axis',(0.,0.,1.));
#142212=DIRECTION('ref_axis',(1.,0.,0.));
#142213=DIRECTION('center_axis',(0.,-3.67394039744206E-16,1.));
#142214=DIRECTION('ref_axis',(-1.,0.,0.));
#142215=DIRECTION('',(0.,3.67394039744206E-16,-1.));
#142216=DIRECTION('center_axis',(1.,-2.1350442781253E-15,-7.84402542373206E-31));
#142217=DIRECTION('ref_axis',(2.1350442781253E-15,1.,5.68845695218989E-62));
#142218=DIRECTION('',(-2.1350442781253E-15,-1.,0.));
#142219=DIRECTION('',(-2.1350442781253E-15,-1.,-3.67394039744206E-16));
#142220=DIRECTION('',(0.,3.67394039744206E-16,-1.));
#142221=DIRECTION('center_axis',(0.,3.67394039744206E-16,-1.));
#142222=DIRECTION('ref_axis',(0.,1.,3.67394039744206E-16));
#142223=DIRECTION('center_axis',(0.,0.,-1.));
#142224=DIRECTION('ref_axis',(1.,0.,0.));
#142225=DIRECTION('center_axis',(0.,3.67394039744206E-16,-1.));
#142226=DIRECTION('ref_axis',(-1.,0.,0.));
#142227=DIRECTION('',(0.,3.67394039744206E-16,-1.));
#142228=DIRECTION('center_axis',(-1.6719208893717E-15,-1.,-3.67394039744206E-16));
#142229=DIRECTION('ref_axis',(1.,-1.6719208893717E-15,0.));
#142230=DIRECTION('',(-1.,1.6719208893717E-15,0.));
#142231=DIRECTION('',(-1.,1.6719208893717E-15,6.14253769678996E-31));
#142232=DIRECTION('',(0.,3.67394039744206E-16,-1.));
#142233=DIRECTION('center_axis',(0.,3.67394039744206E-16,-1.));
#142234=DIRECTION('ref_axis',(0.,1.,3.67394039744206E-16));
#142235=DIRECTION('center_axis',(0.,0.,-1.));
#142236=DIRECTION('ref_axis',(1.,0.,0.));
#142237=DIRECTION('center_axis',(0.,3.67394039744206E-16,-1.));
#142238=DIRECTION('ref_axis',(-1.,0.,0.));
#142239=DIRECTION('',(0.,3.67394039744206E-16,-1.));
#142240=DIRECTION('center_axis',(-0.707106781186548,-0.707106781186548,
-2.59786816870648E-16));
#142241=DIRECTION('ref_axis',(0.707106781186548,-0.707106781186548,1.22182752772918E-34));
#142242=DIRECTION('',(-0.707106781186547,0.707106781186547,0.));
#142243=DIRECTION('',(-0.707106781186547,0.707106781186547,2.59786816870648E-16));
#142244=DIRECTION('',(0.,3.67394039744206E-16,-1.));
#142245=DIRECTION('center_axis',(0.,3.67394039744206E-16,-1.));
#142246=DIRECTION('ref_axis',(0.,1.,3.67394039744206E-16));
#142247=DIRECTION('center_axis',(0.,0.,-1.));
#142248=DIRECTION('ref_axis',(1.,2.31296463463575E-14,0.));
#142249=DIRECTION('center_axis',(0.,3.67394039744206E-16,-1.));
#142250=DIRECTION('ref_axis',(-1.,0.,0.));
#142251=DIRECTION('',(0.,3.67394039744206E-16,-1.));
#142252=DIRECTION('center_axis',(-1.,0.,0.));
#142253=DIRECTION('ref_axis',(0.,0.,1.));
#142254=DIRECTION('',(0.,1.,0.));
#142255=DIRECTION('',(0.,1.,3.67394039744206E-16));
#142256=DIRECTION('center_axis',(-0.499999999999991,0.866025403784444,6.72377758726854E-17));
#142257=DIRECTION('ref_axis',(-0.866025403784444,-0.499999999999991,1.27198190524785E-33));
#142258=DIRECTION('',(0.866025403784444,0.499999999999991,0.));
#142259=DIRECTION('',(1.83697019872103E-16,1.83697019872101E-16,-1.));
#142260=DIRECTION('',(0.866025403784444,0.499999999999991,2.50934795744786E-16));
#142261=DIRECTION('',(1.83697019872103E-16,1.83697019872101E-16,-1.));
#142262=DIRECTION('center_axis',(0.500000000000011,0.866025403784432,2.50934795744787E-16));
#142263=DIRECTION('ref_axis',(-0.866025403784432,0.500000000000011,-2.44665721671821E-33));
#142264=DIRECTION('',(0.866025403784432,-0.500000000000011,0.));
#142265=DIRECTION('',(0.866025403784432,-0.500000000000011,6.72377758726823E-17));
#142266=DIRECTION('',(1.83697019872103E-16,1.83697019872101E-16,-1.));
#142267=DIRECTION('center_axis',(1.04744440165294E-14,1.,1.83697019872103E-16));
#142268=DIRECTION('ref_axis',(-1.,1.04744440165294E-14,0.));
#142269=DIRECTION('',(1.,-1.04744440165294E-14,0.));
#142270=DIRECTION('',(1.,-1.04744440165294E-14,1.83697019872101E-16));
#142271=DIRECTION('',(1.83697019872103E-16,1.83697019872101E-16,-1.));
#142272=DIRECTION('center_axis',(1.83697019872103E-16,1.83697019872101E-16,
-1.));
#142273=DIRECTION('ref_axis',(-1.,3.37445951098915E-32,-1.83697019872103E-16));
#142274=DIRECTION('center_axis',(0.,0.,-1.));
#142275=DIRECTION('ref_axis',(1.,-1.5419764230905E-14,0.));
#142276=DIRECTION('center_axis',(1.83697019872103E-16,1.83697019872101E-16,
-1.));
#142277=DIRECTION('ref_axis',(-1.15648231731787E-14,-1.,-1.83697019872103E-16));
#142278=DIRECTION('',(1.83697019872103E-16,1.83697019872101E-16,-1.));
#142279=DIRECTION('center_axis',(0.707106781186555,0.70710678118654,2.59786816870647E-16));
#142280=DIRECTION('ref_axis',(-0.70710678118654,0.707106781186555,3.44453791271169E-33));
#142281=DIRECTION('',(0.70710678118654,-0.707106781186555,0.));
#142282=DIRECTION('',(0.70710678118654,-0.707106781186555,-1.35585468084861E-30));
#142283=DIRECTION('',(1.83697019872103E-16,1.83697019872101E-16,-1.));
#142284=DIRECTION('center_axis',(1.83697019872103E-16,1.83697019872101E-16,
-1.));
#142285=DIRECTION('ref_axis',(-1.,3.37445951098915E-32,-1.83697019872103E-16));
#142286=DIRECTION('center_axis',(0.,0.,-1.));
#142287=DIRECTION('ref_axis',(1.,8.48087032699776E-14,0.));
#142288=DIRECTION('center_axis',(1.83697019872103E-16,1.83697019872101E-16,
-1.));
#142289=DIRECTION('ref_axis',(-9.63735264431562E-15,-1.,-1.83697019872103E-16));
#142290=DIRECTION('',(1.83697019872103E-16,1.83697019872101E-16,-1.));
#142291=DIRECTION('center_axis',(1.,-8.8025231271577E-15,1.83697019872101E-16));
#142292=DIRECTION('ref_axis',(8.8025231271577E-15,1.,8.2224033292669E-47));
#142293=DIRECTION('',(-8.8025231271577E-15,-1.,0.));
#142294=DIRECTION('',(-8.8025231271577E-15,-1.,-1.83697019872103E-16));
#142295=DIRECTION('',(1.83697019872103E-16,1.83697019872101E-16,-1.));
#142296=DIRECTION('center_axis',(1.83697019872103E-16,1.83697019872101E-16,
-1.));
#142297=DIRECTION('ref_axis',(-1.,3.37445951098915E-32,-1.83697019872103E-16));
#142298=DIRECTION('center_axis',(0.,0.,-1.));
#142299=DIRECTION('ref_axis',(1.,-7.70988211545246E-15,0.));
#142300=DIRECTION('center_axis',(1.83697019872103E-16,1.83697019872101E-16,
-1.));
#142301=DIRECTION('ref_axis',(-9.63735264431562E-15,-1.,-1.83697019872103E-16));
#142302=DIRECTION('',(1.83697019872103E-16,1.83697019872101E-16,-1.));
#142303=DIRECTION('center_axis',(-8.3393997384041E-15,-1.,-1.83697019872103E-16));
#142304=DIRECTION('ref_axis',(1.,-8.3393997384041E-15,0.));
#142305=DIRECTION('',(-1.,8.3393997384041E-15,0.));
#142306=DIRECTION('',(-1.,8.3393997384041E-15,-1.83697019872101E-16));
#142307=DIRECTION('',(1.83697019872103E-16,1.83697019872101E-16,-1.));
#142308=DIRECTION('center_axis',(1.83697019872103E-16,1.83697019872101E-16,
-1.));
#142309=DIRECTION('ref_axis',(-1.,3.37445951098914E-32,-1.83697019872103E-16));
#142310=DIRECTION('center_axis',(0.,0.,1.));
#142311=DIRECTION('ref_axis',(1.,0.,0.));
#142312=DIRECTION('center_axis',(-1.83697019872103E-16,-1.83697019872101E-16,
1.));
#142313=DIRECTION('ref_axis',(-1.15648231731788E-14,-1.,-1.83697019872103E-16));
#142314=DIRECTION('',(1.83697019872103E-16,1.83697019872101E-16,-1.));
#142315=DIRECTION('center_axis',(1.,-7.45753362352625E-15,1.83697019872102E-16));
#142316=DIRECTION('ref_axis',(7.45753362352625E-15,1.,-6.66549012489188E-47));
#142317=DIRECTION('',(-7.45753362352626E-15,-1.,0.));
#142318=DIRECTION('',(-7.45753362352626E-15,-1.,-1.83697019872102E-16));
#142319=DIRECTION('',(1.83697019872103E-16,1.83697019872101E-16,-1.));
#142320=DIRECTION('center_axis',(1.04744440165294E-14,1.,1.83697019872103E-16));
#142321=DIRECTION('ref_axis',(-1.,1.04744440165294E-14,0.));
#142322=DIRECTION('',(1.,-1.04744440165294E-14,0.));
#142323=DIRECTION('',(1.,-1.04744440165294E-14,1.83697019872101E-16));
#142324=DIRECTION('',(1.83697019872103E-16,1.83697019872101E-16,-1.));
#142325=DIRECTION('center_axis',(1.,-1.04744440165294E-14,1.83697019872101E-16));
#142326=DIRECTION('ref_axis',(1.04744440165294E-14,1.,1.01856090860782E-46));
#142327=DIRECTION('',(-1.04744440165294E-14,-1.,0.));
#142328=DIRECTION('',(-1.04744440165294E-14,-1.,-1.83697019872103E-16));
#142329=DIRECTION('center_axis',(2.3090614750906E-14,1.,1.83697019872105E-16));
#142330=DIRECTION('ref_axis',(-1.,2.3090614750906E-14,0.));
#142331=DIRECTION('',(1.,-2.3090614750906E-14,0.));
#142332=DIRECTION('',(1.,-2.3090614750906E-14,1.83697019872099E-16));
#142333=DIRECTION('',(1.83697019872103E-16,1.83697019872101E-16,-1.));
#142334=DIRECTION('center_axis',(1.,-1.67825293837178E-14,1.836970198721E-16));
#142335=DIRECTION('ref_axis',(1.67825293837178E-14,1.,-3.45098319227062E-48));
#142336=DIRECTION('',(-1.67825293837178E-14,-1.,0.));
#142337=DIRECTION('',(-1.67825293837178E-14,-1.,-1.83697019872104E-16));
#142338=DIRECTION('',(1.83697019872103E-16,1.83697019872101E-16,-1.));
#142339=DIRECTION('center_axis',(1.95251751955388E-14,1.,1.83697019872105E-16));
#142340=DIRECTION('ref_axis',(-1.,1.95251751955388E-14,0.));
#142341=DIRECTION('',(1.,-1.95251751955388E-14,0.));
#142342=DIRECTION('',(1.,-1.95251751955388E-14,1.83697019872099E-16));
#142343=DIRECTION('',(1.83697019872103E-16,1.83697019872101E-16,-1.));
#142344=DIRECTION('center_axis',(1.83697019872103E-16,1.83697019872101E-16,
-1.));
#142345=DIRECTION('ref_axis',(-1.,3.37445951098914E-32,-1.83697019872103E-16));
#142346=DIRECTION('center_axis',(0.,0.,1.));
#142347=DIRECTION('ref_axis',(1.,0.,0.));
#142348=DIRECTION('center_axis',(-1.83697019872103E-16,-1.83697019872101E-16,
1.));
#142349=DIRECTION('ref_axis',(7.70988211545252E-15,1.,1.83697019872102E-16));
#142350=DIRECTION('',(1.83697019872103E-16,1.83697019872101E-16,-1.));
#142351=DIRECTION('center_axis',(-1.,1.90146211290306E-14,-1.836970198721E-16));
#142352=DIRECTION('ref_axis',(-1.90146211290306E-14,-1.,-5.41562530658295E-47));
#142353=DIRECTION('',(1.90146211290306E-14,1.,0.));
#142354=DIRECTION('',(1.90146211290306E-14,1.,1.83697019872105E-16));
#142355=DIRECTION('',(1.83697019872103E-16,1.83697019872101E-16,-1.));
#142356=DIRECTION('center_axis',(1.83697019872103E-16,1.83697019872101E-16,
-1.));
#142357=DIRECTION('ref_axis',(-1.,3.37445951098915E-32,-1.83697019872103E-16));
#142358=DIRECTION('center_axis',(0.,0.,-1.));
#142359=DIRECTION('ref_axis',(1.,0.,0.));
#142360=DIRECTION('center_axis',(1.83697019872103E-16,1.83697019872101E-16,
-1.));
#142361=DIRECTION('ref_axis',(7.70988211545246E-15,1.,1.83697019872102E-16));
#142362=DIRECTION('',(1.83697019872103E-16,1.83697019872101E-16,-1.));
#142363=DIRECTION('center_axis',(1.88340484633879E-14,1.,1.83697019872105E-16));
#142364=DIRECTION('ref_axis',(-1.,1.88340484633879E-14,0.));
#142365=DIRECTION('',(1.,-1.88340484633879E-14,0.));
#142366=DIRECTION('',(1.,-1.88340484633879E-14,1.836970198721E-16));
#142367=DIRECTION('',(1.83697019872103E-16,1.83697019872101E-16,-1.));
#142368=DIRECTION('center_axis',(1.83697019872103E-16,1.83697019872101E-16,
-1.));
#142369=DIRECTION('ref_axis',(-1.,3.37445951098915E-32,-1.83697019872103E-16));
#142370=DIRECTION('center_axis',(0.,0.,-1.));
#142371=DIRECTION('ref_axis',(1.,2.31296463463575E-14,0.));
#142372=DIRECTION('center_axis',(1.83697019872103E-16,1.83697019872101E-16,
-1.));
#142373=DIRECTION('ref_axis',(7.70988211545251E-15,1.,1.83697019872102E-16));
#142374=DIRECTION('',(1.83697019872103E-16,1.83697019872101E-16,-1.));
#142375=DIRECTION('center_axis',(0.70710678118656,0.707106781186535,2.59786816870647E-16));
#142376=DIRECTION('ref_axis',(-0.707106781186535,0.70710678118656,-1.00703162523782E-33));
#142377=DIRECTION('',(0.707106781186535,-0.70710678118656,0.));
#142378=DIRECTION('',(0.707106781186535,-0.70710678118656,-3.27870313732483E-30));
#142379=DIRECTION('',(1.83697019872103E-16,1.83697019872101E-16,-1.));
#142380=DIRECTION('center_axis',(1.83697019872103E-16,1.83697019872101E-16,
-1.));
#142381=DIRECTION('ref_axis',(-1.,3.37445951098915E-32,-1.83697019872103E-16));
#142382=DIRECTION('center_axis',(0.,0.,-1.));
#142383=DIRECTION('ref_axis',(1.,1.11793290674061E-13,0.));
#142384=DIRECTION('center_axis',(1.83697019872103E-16,1.83697019872101E-16,
-1.));
#142385=DIRECTION('ref_axis',(7.70988211545249E-15,1.,1.83697019872103E-16));
#142386=DIRECTION('',(1.83697019872103E-16,1.83697019872101E-16,-1.));
#142387=DIRECTION('center_axis',(1.,-1.92029268069249E-14,1.83697019872099E-16));
#142388=DIRECTION('ref_axis',(1.92029268069249E-14,1.,-2.4224977382315E-46));
#142389=DIRECTION('',(-1.92029268069249E-14,-1.,0.));
#142390=DIRECTION('',(-1.92029268069249E-14,-1.,-1.83697019872105E-16));
#142391=DIRECTION('',(1.83697019872103E-16,1.83697019872101E-16,-1.));
#142392=DIRECTION('center_axis',(0.866025403784456,0.49999999999997,2.50934795744784E-16));
#142393=DIRECTION('ref_axis',(-0.49999999999997,0.866025403784456,3.80143372866314E-33));
#142394=DIRECTION('',(0.49999999999997,-0.866025403784456,0.));
#142395=DIRECTION('',(0.49999999999997,-0.866025403784456,-6.72377758726917E-17));
#142396=DIRECTION('',(1.83697019872103E-16,1.83697019872101E-16,-1.));
#142397=DIRECTION('center_axis',(0.866025403784431,-0.500000000000013,6.72377758726818E-17));
#142398=DIRECTION('ref_axis',(0.500000000000013,0.866025403784431,-1.6659815170822E-33));
#142399=DIRECTION('',(-0.500000000000013,-0.866025403784431,0.));
#142400=DIRECTION('',(-0.500000000000013,-0.866025403784431,-2.50934795744787E-16));
#142401=DIRECTION('',(1.83697019872103E-16,1.83697019872101E-16,-1.));
#142402=DIRECTION('center_axis',(1.,-1.04744440165294E-14,1.83697019872101E-16));
#142403=DIRECTION('ref_axis',(1.04744440165294E-14,1.,1.01856090860782E-46));
#142404=DIRECTION('',(-1.04744440165294E-14,-1.,0.));
#142405=DIRECTION('',(-1.04744440165294E-14,-1.,-1.83697019872103E-16));
#142406=DIRECTION('',(1.83697019872103E-16,1.83697019872101E-16,-1.));
#142407=DIRECTION('center_axis',(1.83697019872103E-16,1.83697019872101E-16,
-1.));
#142408=DIRECTION('ref_axis',(-1.,3.37445951098915E-32,-1.83697019872103E-16));
#142409=DIRECTION('center_axis',(0.,0.,-1.));
#142410=DIRECTION('ref_axis',(1.,-7.70988211545249E-15,0.));
#142411=DIRECTION('center_axis',(1.83697019872103E-16,1.83697019872101E-16,
-1.));
#142412=DIRECTION('ref_axis',(7.70988211545249E-15,1.,1.83697019872103E-16));
#142413=DIRECTION('',(1.83697019872103E-16,1.83697019872101E-16,-1.));
#142414=DIRECTION('center_axis',(0.70710678118654,-0.707106781186555,-1.36533618211329E-30));
#142415=DIRECTION('ref_axis',(0.707106781186555,0.70710678118654,3.7321785051642E-47));
#142416=DIRECTION('',(-0.707106781186555,-0.70710678118654,0.));
#142417=DIRECTION('',(-0.707106781186555,-0.70710678118654,-2.59786816870647E-16));
#142418=DIRECTION('',(1.83697019872103E-16,1.83697019872101E-16,-1.));
#142419=DIRECTION('center_axis',(1.83697019872103E-16,1.83697019872101E-16,
-1.));
#142420=DIRECTION('ref_axis',(-1.,3.37445951098915E-32,-1.83697019872103E-16));
#142421=DIRECTION('center_axis',(0.,0.,-1.));
#142422=DIRECTION('ref_axis',(1.,0.,0.));
#142423=DIRECTION('center_axis',(1.83697019872103E-16,1.83697019872101E-16,
-1.));
#142424=DIRECTION('ref_axis',(7.70988211545249E-15,1.,1.83697019872103E-16));
#142425=DIRECTION('',(1.83697019872103E-16,1.83697019872101E-16,-1.));
#142426=DIRECTION('center_axis',(-1.04744440165294E-14,-1.,-1.83697019872103E-16));
#142427=DIRECTION('ref_axis',(1.,-1.04744440165294E-14,0.));
#142428=DIRECTION('',(-1.,1.04744440165294E-14,0.));
#142429=DIRECTION('',(-1.,1.04744440165294E-14,-1.83697019872101E-16));
#142430=DIRECTION('',(1.83697019872103E-16,1.83697019872101E-16,-1.));
#142431=DIRECTION('center_axis',(1.83697019872103E-16,1.83697019872101E-16,
-1.));
#142432=DIRECTION('ref_axis',(-1.,3.37445951098914E-32,-1.83697019872103E-16));
#142433=DIRECTION('center_axis',(0.,0.,-1.));
#142434=DIRECTION('ref_axis',(1.,0.,0.));
#142435=DIRECTION('center_axis',(1.83697019872103E-16,1.83697019872101E-16,
-1.));
#142436=DIRECTION('ref_axis',(7.70988211545255E-15,1.,1.83697019872102E-16));
#142437=DIRECTION('',(1.83697019872103E-16,1.83697019872101E-16,-1.));
#142438=DIRECTION('center_axis',(-1.,8.3393997384041E-15,-1.83697019872101E-16));
#142439=DIRECTION('ref_axis',(-8.3393997384041E-15,-1.,-6.10222580802198E-47));
#142440=DIRECTION('',(8.3393997384041E-15,1.,0.));
#142441=DIRECTION('',(8.3393997384041E-15,1.,1.83697019872103E-16));
#142442=DIRECTION('',(1.83697019872103E-16,1.83697019872101E-16,-1.));
#142443=DIRECTION('center_axis',(1.83697019872103E-16,1.83697019872101E-16,
-1.));
#142444=DIRECTION('ref_axis',(-1.,3.37445951098915E-32,-1.83697019872103E-16));
#142445=DIRECTION('center_axis',(0.,0.,1.));
#142446=DIRECTION('ref_axis',(1.,0.,0.));
#142447=DIRECTION('center_axis',(-1.83697019872103E-16,-1.83697019872101E-16,
1.));
#142448=DIRECTION('ref_axis',(7.70988211545249E-15,1.,1.83697019872103E-16));
#142449=DIRECTION('',(1.83697019872103E-16,1.83697019872101E-16,-1.));
#142450=DIRECTION('center_axis',(-1.04744440165294E-14,-1.,-1.83697019872103E-16));
#142451=DIRECTION('ref_axis',(1.,-1.04744440165294E-14,0.));
#142452=DIRECTION('',(-1.,1.04744440165294E-14,0.));
#142453=DIRECTION('',(-1.,1.04744440165294E-14,-1.83697019872101E-16));
#142454=DIRECTION('',(1.83697019872103E-16,1.83697019872101E-16,-1.));
#142455=DIRECTION('center_axis',(1.,-1.04744440165294E-14,1.83697019872101E-16));
#142456=DIRECTION('ref_axis',(1.04744440165294E-14,1.,1.01856090860782E-46));
#142457=DIRECTION('',(-1.04744440165294E-14,-1.,0.));
#142458=DIRECTION('',(-1.04744440165294E-14,-1.,-1.83697019872103E-16));
#142459=DIRECTION('',(1.83697019872103E-16,1.83697019872101E-16,-1.));
#142460=DIRECTION('center_axis',(-1.04744440165294E-14,-1.,-1.83697019872103E-16));
#142461=DIRECTION('ref_axis',(1.,-1.04744440165294E-14,0.));
#142462=DIRECTION('',(-1.,1.04744440165294E-14,0.));
#142463=DIRECTION('',(-1.,1.04744440165294E-14,-1.83697019872101E-16));
#142464=DIRECTION('',(1.83697019872103E-16,1.83697019872101E-16,-1.));
#142465=DIRECTION('center_axis',(1.,-1.04744440165294E-14,1.83697019872101E-16));
#142466=DIRECTION('ref_axis',(1.04744440165294E-14,1.,1.01856090860782E-46));
#142467=DIRECTION('',(-1.04744440165294E-14,-1.,0.));
#142468=DIRECTION('',(-1.04744440165294E-14,-1.,-1.83697019872103E-16));
#142469=DIRECTION('',(1.83697019872103E-16,1.83697019872101E-16,-1.));
#142470=DIRECTION('center_axis',(1.83697019872103E-16,1.83697019872101E-16,
-1.));
#142471=DIRECTION('ref_axis',(-1.,3.37445951098915E-32,-1.83697019872103E-16));
#142472=DIRECTION('center_axis',(0.,0.,1.));
#142473=DIRECTION('ref_axis',(1.,0.,0.));
#142474=DIRECTION('center_axis',(-1.83697019872103E-16,-1.83697019872101E-16,
1.));
#142475=DIRECTION('ref_axis',(1.13826999736009E-14,1.,1.83697019872103E-16));
#142476=DIRECTION('',(1.83697019872103E-16,1.83697019872101E-16,-1.));
#142477=DIRECTION('center_axis',(1.08865902450817E-14,1.,1.83697019872103E-16));
#142478=DIRECTION('ref_axis',(-1.,1.08865902450817E-14,0.));
#142479=DIRECTION('',(1.,-1.08865902450817E-14,0.));
#142480=DIRECTION('',(1.,-1.08865902450817E-14,1.83697019872101E-16));
#142481=DIRECTION('',(1.83697019872103E-16,1.83697019872101E-16,-1.));
#142482=DIRECTION('center_axis',(-1.,1.04744440165294E-14,-1.83697019872101E-16));
#142483=DIRECTION('ref_axis',(-1.04744440165294E-14,-1.,-1.01856090860782E-46));
#142484=DIRECTION('',(1.04744440165294E-14,1.,0.));
#142485=DIRECTION('',(1.04744440165294E-14,1.,1.83697019872103E-16));
#142486=DIRECTION('',(1.83697019872103E-16,1.83697019872101E-16,-1.));
#142487=DIRECTION('center_axis',(1.04744440165294E-14,1.,1.83697019872103E-16));
#142488=DIRECTION('ref_axis',(-1.,1.04744440165294E-14,0.));
#142489=DIRECTION('',(1.,-1.04744440165294E-14,0.));
#142490=DIRECTION('',(1.,-1.04744440165294E-14,1.83697019872101E-16));
#142491=DIRECTION('',(1.83697019872103E-16,1.83697019872101E-16,-1.));
#142492=DIRECTION('center_axis',(-1.,1.34913544095325E-14,-1.83697019872101E-16));
#142493=DIRECTION('ref_axis',(-1.34913544095325E-14,-1.,-1.3549484701482E-46));
#142494=DIRECTION('',(1.34913544095325E-14,1.,0.));
#142495=DIRECTION('',(1.34913544095325E-14,1.,1.83697019872104E-16));
#142496=DIRECTION('',(1.83697019872103E-16,1.83697019872101E-16,-1.));
#142497=DIRECTION('center_axis',(1.83697019872103E-16,1.83697019872101E-16,
-1.));
#142498=DIRECTION('ref_axis',(-1.,3.37445951098914E-32,-1.83697019872103E-16));
#142499=DIRECTION('center_axis',(0.,0.,1.));
#142500=DIRECTION('ref_axis',(1.,0.,0.));
#142501=DIRECTION('center_axis',(-1.83697019872103E-16,-1.83697019872101E-16,
1.));
#142502=DIRECTION('ref_axis',(7.70988211545255E-15,1.,1.83697019872102E-16));
#142503=DIRECTION('',(1.83697019872103E-16,1.83697019872101E-16,-1.));
#142504=DIRECTION('center_axis',(-1.26094882946547E-14,-1.,-1.83697019872103E-16));
#142505=DIRECTION('ref_axis',(1.,-1.26094882946547E-14,0.));
#142506=DIRECTION('',(-1.,1.26094882946547E-14,0.));
#142507=DIRECTION('',(-1.,1.26094882946547E-14,-1.83697019872101E-16));
#142508=DIRECTION('',(1.83697019872103E-16,1.83697019872101E-16,-1.));
#142509=DIRECTION('center_axis',(1.83697019872103E-16,1.83697019872101E-16,
-1.));
#142510=DIRECTION('ref_axis',(-1.,3.37445951098915E-32,-1.83697019872103E-16));
#142511=DIRECTION('center_axis',(0.,0.,-1.));
#142512=DIRECTION('ref_axis',(1.,0.,0.));
#142513=DIRECTION('center_axis',(1.83697019872103E-16,1.83697019872101E-16,
-1.));
#142514=DIRECTION('ref_axis',(7.70988211545249E-15,1.,1.83697019872103E-16));
#142515=DIRECTION('',(1.83697019872103E-16,1.83697019872101E-16,-1.));
#142516=DIRECTION('center_axis',(-1.,1.21463649059011E-14,-1.83697019872101E-16));
#142517=DIRECTION('ref_axis',(-1.21463649059011E-14,-1.,-1.73669008789231E-46));
#142518=DIRECTION('',(1.21463649059011E-14,1.,0.));
#142519=DIRECTION('',(1.21463649059011E-14,1.,1.83697019872103E-16));
#142520=DIRECTION('',(1.83697019872103E-16,1.83697019872101E-16,-1.));
#142521=DIRECTION('center_axis',(1.83697019872103E-16,1.83697019872101E-16,
-1.));
#142522=DIRECTION('ref_axis',(-1.,3.37445951098915E-32,-1.83697019872103E-16));
#142523=DIRECTION('center_axis',(0.,0.,-1.));
#142524=DIRECTION('ref_axis',(1.,0.,0.));
#142525=DIRECTION('center_axis',(1.83697019872103E-16,1.83697019872101E-16,
-1.));
#142526=DIRECTION('ref_axis',(7.70988211545249E-15,1.,1.83697019872103E-16));
#142527=DIRECTION('',(1.83697019872103E-16,1.83697019872101E-16,-1.));
#142528=DIRECTION('center_axis',(-0.70710678118654,0.707106781186555,1.36533618211329E-30));
#142529=DIRECTION('ref_axis',(-0.707106781186555,-0.70710678118654,-3.7321785051642E-47));
#142530=DIRECTION('',(0.707106781186555,0.70710678118654,0.));
#142531=DIRECTION('',(0.707106781186555,0.70710678118654,2.59786816870647E-16));
#142532=DIRECTION('',(1.83697019872103E-16,1.83697019872101E-16,-1.));
#142533=DIRECTION('center_axis',(1.83697019872103E-16,1.83697019872101E-16,
-1.));
#142534=DIRECTION('ref_axis',(-1.,3.37445951098915E-32,-1.83697019872103E-16));
#142535=DIRECTION('center_axis',(0.,0.,-1.));
#142536=DIRECTION('ref_axis',(1.,3.083952846181E-14,0.));
#142537=DIRECTION('center_axis',(1.83697019872103E-16,1.83697019872101E-16,
-1.));
#142538=DIRECTION('ref_axis',(7.70988211545249E-15,1.,1.83697019872103E-16));
#142539=DIRECTION('',(1.83697019872103E-16,1.83697019872101E-16,-1.));
#142540=DIRECTION('center_axis',(1.04744440165294E-14,1.,1.83697019872103E-16));
#142541=DIRECTION('ref_axis',(-1.,1.04744440165294E-14,0.));
#142542=DIRECTION('',(1.,-1.04744440165294E-14,0.));
#142543=DIRECTION('',(1.,-1.04744440165294E-14,1.83697019872101E-16));
#142544=DIRECTION('center_axis',(-0.707106781186542,0.707106781186553,0.));
#142545=DIRECTION('ref_axis',(-0.707106781186553,-0.707106781186542,0.));
#142546=DIRECTION('',(0.707106781186553,0.707106781186542,0.));
#142547=DIRECTION('',(0.,0.,1.));
#142548=DIRECTION('',(0.707106781186553,0.707106781186542,0.));
#142549=DIRECTION('center_axis',(-0.70710678118655,-0.707106781186545,0.));
#142550=DIRECTION('ref_axis',(0.707106781186545,-0.70710678118655,0.));
#142551=DIRECTION('',(-0.707106781186545,0.70710678118655,0.));
#142552=DIRECTION('',(-0.707106781186545,0.70710678118655,0.));
#142553=DIRECTION('center_axis',(-0.70710678118655,0.707106781186545,0.));
#142554=DIRECTION('ref_axis',(-0.707106781186545,-0.70710678118655,0.));
#142555=DIRECTION('',(0.707106781186545,0.70710678118655,0.));
#142556=DIRECTION('',(0.707106781186545,0.70710678118655,0.));
#142557=DIRECTION('',(0.,0.,1.));
#142558=DIRECTION('center_axis',(0.70710678118655,0.707106781186545,0.));
#142559=DIRECTION('ref_axis',(-0.707106781186545,0.70710678118655,0.));
#142560=DIRECTION('',(0.707106781186545,-0.70710678118655,0.));
#142561=DIRECTION('',(0.707106781186545,-0.70710678118655,0.));
#142562=DIRECTION('center_axis',(0.,0.,-1.));
#142563=DIRECTION('ref_axis',(-1.,0.,0.));
#142564=DIRECTION('',(0.,1.,0.));
#142565=DIRECTION('',(1.,-1.21430643318376E-16,0.));
#142566=DIRECTION('',(-3.25988935000123E-16,-1.,0.));
#142567=DIRECTION('',(1.,0.,0.));
#142568=DIRECTION('',(0.,1.,0.));
#142569=DIRECTION('',(1.,-1.21430643318376E-16,0.));
#142570=DIRECTION('',(0.,1.,0.));
#142571=DIRECTION('',(-1.,0.,0.));
#142572=DIRECTION('center_axis',(0.,1.,0.));
#142573=DIRECTION('ref_axis',(0.,0.,1.));
#142574=DIRECTION('',(-1.,0.,0.));
#142575=DIRECTION('',(0.,0.,1.));
#142576=DIRECTION('',(0.,0.,1.));
#142577=DIRECTION('center_axis',(1.,0.,0.));
#142578=DIRECTION('ref_axis',(0.,0.,-1.));
#142579=DIRECTION('',(0.,1.,0.));
#142580=DIRECTION('',(0.,0.,1.));
#142581=DIRECTION('center_axis',(-1.21430643318376E-16,-1.,0.));
#142582=DIRECTION('ref_axis',(1.,-1.21430643318376E-16,0.));
#142583=DIRECTION('',(1.,-1.21430643318376E-16,0.));
#142584=DIRECTION('',(0.,0.,1.));
#142585=DIRECTION('center_axis',(1.,0.,0.));
#142586=DIRECTION('ref_axis',(0.,0.,-1.));
#142587=DIRECTION('',(0.,1.,0.));
#142588=DIRECTION('',(0.,0.,1.));
#142589=DIRECTION('center_axis',(0.,-1.,0.));
#142590=DIRECTION('ref_axis',(0.,0.,-1.));
#142591=DIRECTION('',(1.,0.,0.));
#142592=DIRECTION('',(0.,0.,1.));
#142593=DIRECTION('center_axis',(-1.,3.25988935000123E-16,0.));
#142594=DIRECTION('ref_axis',(-3.25988935000123E-16,-1.,0.));
#142595=DIRECTION('',(-3.25988935000123E-16,-1.,0.));
#142596=DIRECTION('',(0.,0.,1.));
#142597=DIRECTION('center_axis',(-1.21430643318376E-16,-1.,0.));
#142598=DIRECTION('ref_axis',(1.,-1.21430643318376E-16,0.));
#142599=DIRECTION('',(1.,-1.21430643318376E-16,0.));
#142600=DIRECTION('',(0.,0.,1.));
#142601=DIRECTION('center_axis',(1.,0.,0.));
#142602=DIRECTION('ref_axis',(0.,0.,-1.));
#142603=DIRECTION('',(0.,1.,0.));
#142604=DIRECTION('center_axis',(0.,0.,-1.));
#142605=DIRECTION('ref_axis',(-1.,0.,0.));
#142606=DIRECTION('center_axis',(-1.60944926250024E-16,1.,0.));
#142607=DIRECTION('ref_axis',(-1.,-1.60944926250024E-16,0.));
#142608=DIRECTION('',(-1.,-1.60944926250024E-16,0.));
#142609=DIRECTION('',(0.,0.,1.));
#142610=DIRECTION('',(-1.,-1.60944926250024E-16,0.));
#142611=DIRECTION('',(0.,0.,1.));
#142612=DIRECTION('center_axis',(-1.,0.,0.));
#142613=DIRECTION('ref_axis',(0.,0.,1.));
#142614=DIRECTION('',(0.,-1.,0.));
#142615=DIRECTION('',(0.,-1.,0.));
#142616=DIRECTION('',(0.,0.,1.));
#142617=DIRECTION('center_axis',(0.,-1.,0.));
#142618=DIRECTION('ref_axis',(0.,0.,-1.));
#142619=DIRECTION('',(1.,0.,0.));
#142620=DIRECTION('',(1.,0.,0.));
#142621=DIRECTION('',(0.,0.,1.));
#142622=DIRECTION('center_axis',(1.,0.,0.));
#142623=DIRECTION('ref_axis',(0.,0.,-1.));
#142624=DIRECTION('',(0.,1.,0.));
#142625=DIRECTION('',(0.,1.,0.));
#142626=DIRECTION('center_axis',(0.,0.,1.));
#142627=DIRECTION('ref_axis',(1.,0.,0.));
#142628=DIRECTION('center_axis',(0.,0.,-1.));
#142629=DIRECTION('ref_axis',(-1.,0.,0.));
#274150=CARTESIAN_POINT('',(0.,0.,0.));
#274151=CARTESIAN_POINT('Origin',(-27.0086446004716,-26.9913553995289,910.));
#274152=CARTESIAN_POINT('',(-32.6729361631489,-24.2334937110131,1282.35584962783));
#274153=CARTESIAN_POINT('',(-32.6729361631488,-29.7492170880442,1282.35584962783));
#274154=CARTESIAN_POINT('Origin',(-27.0086446004717,-26.991355399529,1282.35584962783));
#274155=CARTESIAN_POINT('',(-32.6729361631488,-29.7492170880442,-260.));
#274156=CARTESIAN_POINT('',(-32.672936163149,-29.7492170880444,910.));
#274157=CARTESIAN_POINT('',(-32.6729361631487,-24.233493711013,-260.));
#274158=CARTESIAN_POINT('Origin',(-27.0086446004714,-26.9913553995287,-260.));
#274159=CARTESIAN_POINT('',(-32.6729361631489,-24.2334937110132,910.));
#274160=CARTESIAN_POINT('Origin',(0.,0.,-260.));
#274161=CARTESIAN_POINT('',(-35.1310673206098,-32.6891089669783,-260.));
#274162=CARTESIAN_POINT('',(-32.706398167921,-35.1137781196668,-260.));
#274163=CARTESIAN_POINT('Origin',(-27.0086446004714,-26.9913553995287,-260.));
#274164=CARTESIAN_POINT('',(-29.7665062889871,-32.655646962206,-260.));
#274165=CARTESIAN_POINT('',(-32.706398167921,-35.1137781196668,-260.));
#274166=CARTESIAN_POINT('',(-24.2507829119558,-32.6556469622061,-260.));
#274167=CARTESIAN_POINT('Origin',(-27.0086446004714,-26.9913553995287,-260.));
#274168=CARTESIAN_POINT('',(-21.3108910330219,-35.1137781196669,-260.));
#274169=CARTESIAN_POINT('',(-21.3108910330219,-35.1137781196669,-260.));
#274170=CARTESIAN_POINT('',(-18.8862218803333,-32.6891089669783,-260.));
#274171=CARTESIAN_POINT('Origin',(-27.0086446004714,-26.9913553995287,-260.));
#274172=CARTESIAN_POINT('',(-21.3443530377941,-29.7492170880443,-260.));
#274173=CARTESIAN_POINT('',(-18.8862218803333,-32.6891089669783,-260.));
#274174=CARTESIAN_POINT('',(-21.344353037794,-24.2334937110131,-260.));
#274175=CARTESIAN_POINT('Origin',(-27.0086446004714,-26.9913553995287,-260.));
#274176=CARTESIAN_POINT('',(-18.8862218803333,-21.2936018320792,-260.));
#274177=CARTESIAN_POINT('',(-18.8862218803333,-21.2936018320792,-260.));
#274178=CARTESIAN_POINT('',(-21.3108910330219,-18.8689326793906,-260.));
#274179=CARTESIAN_POINT('Origin',(-27.0086446004714,-26.9913553995287,-260.));
#274180=CARTESIAN_POINT('',(-24.2507829119558,-21.3270638368514,-260.));
#274181=CARTESIAN_POINT('',(-21.3108910330219,-18.8689326793906,-260.));
#274182=CARTESIAN_POINT('',(-29.7665062889869,-21.3270638368513,-260.));
#274183=CARTESIAN_POINT('Origin',(-27.0086446004714,-26.9913553995287,-260.));
#274184=CARTESIAN_POINT('',(-32.7063981679207,-18.8689326793905,-260.));
#274185=CARTESIAN_POINT('',(-32.7063981679207,-18.8689326793905,-260.));
#274186=CARTESIAN_POINT('',(-35.1310673206094,-21.293601832079,-260.));
#274187=CARTESIAN_POINT('Origin',(-27.0086446004714,-26.9913553995287,-260.));
#274188=CARTESIAN_POINT('',(-35.1310673206094,-21.293601832079,-260.));
#274189=CARTESIAN_POINT('',(-35.1310673206096,-32.6891089669781,-260.));
#274190=CARTESIAN_POINT('Origin',(-35.1310673206098,-32.6891089669783,910.));
#274191=CARTESIAN_POINT('',(-35.1310673206099,-32.6891089669784,1282.35584962783));
#274192=CARTESIAN_POINT('',(-35.1310673206098,-32.6891089669783,1282.35584962783));
#274193=CARTESIAN_POINT('',(-35.1310673206098,-32.6891089669783,910.));
#274194=CARTESIAN_POINT('Origin',(-35.1310673206096,-21.2936018320792,910.));
#274195=CARTESIAN_POINT('',(-35.1310673206099,-21.293601832079,1282.35584962783));
#274196=CARTESIAN_POINT('',(-35.1310673206096,-21.2936018320792,910.));
#274197=CARTESIAN_POINT('',(-35.1310673206097,-21.2936018320793,1282.35584962783));
#274198=CARTESIAN_POINT('Origin',(-27.0086446004716,-26.9913553995289,910.));
#274199=CARTESIAN_POINT('',(-32.7063981679208,-18.8689326793906,1282.35584962783));
#274200=CARTESIAN_POINT('',(-32.7063981679209,-18.8689326793907,910.));
#274201=CARTESIAN_POINT('Origin',(-27.0086446004717,-26.991355399529,1282.35584962783));
#274202=CARTESIAN_POINT('Origin',(-32.7063981679209,-18.8689326793907,910.));
#274203=CARTESIAN_POINT('',(-29.7665062889869,-21.3270638368518,1282.35584962783));
#274204=CARTESIAN_POINT('',(-29.7665062889871,-21.3270638368515,910.));
#274205=CARTESIAN_POINT('',(-32.706398167921,-18.8689326793908,1282.35584962783));
#274206=CARTESIAN_POINT('Origin',(-27.0086446004716,-26.9913553995289,910.));
#274207=CARTESIAN_POINT('',(-24.250782911956,-21.3270638368517,1282.35584962783));
#274208=CARTESIAN_POINT('',(-24.250782911956,-21.3270638368516,910.));
#274209=CARTESIAN_POINT('Origin',(-27.0086446004717,-26.991355399529,1282.35584962783));
#274210=CARTESIAN_POINT('Origin',(-21.3108910330221,-18.8689326793908,910.));
#274211=CARTESIAN_POINT('',(-21.3108910330219,-18.8689326793906,1282.35584962783));
#274212=CARTESIAN_POINT('',(-21.3108910330221,-18.8689326793908,910.));
#274213=CARTESIAN_POINT('',(-21.3108910330221,-18.8689326793908,1282.35584962783));
#274214=CARTESIAN_POINT('Origin',(-27.0086446004716,-26.9913553995289,910.));
#274215=CARTESIAN_POINT('',(-18.8862218803336,-21.2936018320794,1282.35584962783));
#274216=CARTESIAN_POINT('',(-18.8862218803335,-21.2936018320794,910.));
#274217=CARTESIAN_POINT('Origin',(-27.0086446004717,-26.991355399529,1282.35584962783));
#274218=CARTESIAN_POINT('Origin',(-18.8862218803335,-21.2936018320794,910.));
#274219=CARTESIAN_POINT('',(-21.3443530377943,-24.2334937110133,1282.35584962783));
#274220=CARTESIAN_POINT('',(-21.3443530377943,-24.2334937110133,910.));
#274221=CARTESIAN_POINT('',(-18.8862218803335,-21.2936018320794,1282.35584962783));
#274222=CARTESIAN_POINT('Origin',(-27.0086446004716,-26.9913553995289,910.));
#274223=CARTESIAN_POINT('',(-21.3443530377942,-29.7492170880444,1282.35584962783));
#274224=CARTESIAN_POINT('',(-21.3443530377943,-29.7492170880446,910.));
#274225=CARTESIAN_POINT('Origin',(-27.0086446004717,-26.991355399529,1282.35584962783));
#274226=CARTESIAN_POINT('Origin',(-18.8862218803335,-32.6891089669785,910.));
#274227=CARTESIAN_POINT('',(-18.8862218803336,-32.6891089669785,1282.35584962783));
#274228=CARTESIAN_POINT('',(-18.8862218803335,-32.6891089669785,910.));
#274229=CARTESIAN_POINT('',(-18.8862218803336,-32.6891089669786,1282.35584962783));
#274230=CARTESIAN_POINT('Origin',(-27.0086446004716,-26.9913553995289,910.));
#274231=CARTESIAN_POINT('',(-21.310891033022,-35.113778119667,1282.35584962783));
#274232=CARTESIAN_POINT('',(-21.3108910330221,-35.1137781196671,910.));
#274233=CARTESIAN_POINT('Origin',(-27.0086446004717,-26.991355399529,1282.35584962783));
#274234=CARTESIAN_POINT('Origin',(-21.3108910330221,-35.1137781196671,910.));
#274235=CARTESIAN_POINT('',(-24.2507829119561,-32.6556469622064,1282.35584962783));
#274236=CARTESIAN_POINT('',(-24.2507829119561,-32.6556469622063,910.));
#274237=CARTESIAN_POINT('',(-21.3108910330222,-35.1137781196672,1282.35584962783));
#274238=CARTESIAN_POINT('Origin',(-27.0086446004716,-26.9913553995289,910.));
#274239=CARTESIAN_POINT('',(-29.7665062889873,-32.6556469622064,1282.35584962783));
#274240=CARTESIAN_POINT('',(-29.7665062889873,-32.6556469622062,910.));
#274241=CARTESIAN_POINT('Origin',(-27.0086446004717,-26.991355399529,1282.35584962783));
#274242=CARTESIAN_POINT('Origin',(-32.7063981679213,-35.113778119667,910.));
#274243=CARTESIAN_POINT('',(-32.7063981679213,-35.113778119667,1282.35584962783));
#274244=CARTESIAN_POINT('',(-32.7063981679213,-35.113778119667,910.));
#274245=CARTESIAN_POINT('',(-32.7063981679212,-35.113778119667,1282.35584962783));
#274246=CARTESIAN_POINT('Origin',(-27.0086446004716,-26.9913553995289,910.));
#274247=CARTESIAN_POINT('Origin',(-27.0086446004717,-26.991355399529,1282.35584962783));
#274248=CARTESIAN_POINT('Origin',(0.,0.,1282.35584962783));
#274249=CARTESIAN_POINT('Origin',(0.,0.,-260.));
#274250=CARTESIAN_POINT('',(-45.9014446004718,-51.6603553995284,-260.));
#274251=CARTESIAN_POINT('',(-44.1014446004718,-49.8603553995284,-260.));
#274252=CARTESIAN_POINT('Origin',(-45.9014446004718,-49.8603553995284,-260.));
#274253=CARTESIAN_POINT('',(-44.1014446004717,-45.8841553995285,-260.));
#274254=CARTESIAN_POINT('',(-44.1014446004718,-49.8603553995284,-260.));
#274255=CARTESIAN_POINT('',(-45.9014446004717,-44.0841553995285,-260.));
#274256=CARTESIAN_POINT('Origin',(-45.9014446004717,-45.8841553995285,-260.));
#274257=CARTESIAN_POINT('',(-49.8776446004716,-44.0841553995285,-260.));
#274258=CARTESIAN_POINT('',(-45.9014446004717,-44.0841553995285,-260.));
#274259=CARTESIAN_POINT('',(-51.6776446004716,-45.8841553995285,-260.));
#274260=CARTESIAN_POINT('Origin',(-49.8776446004716,-45.8841553995285,-260.));
#274261=CARTESIAN_POINT('',(-51.6776446004716,-49.8603553995283,-260.));
#274262=CARTESIAN_POINT('',(-51.6776446004716,-45.8841553995285,-260.));
#274263=CARTESIAN_POINT('',(-49.8776446004716,-51.6603553995283,-260.));
#274264=CARTESIAN_POINT('Origin',(-49.8776446004716,-49.8603553995283,-260.));
#274265=CARTESIAN_POINT('',(-49.8776446004716,-51.6603553995283,-260.));
#274266=CARTESIAN_POINT('Origin',(-49.8776446004719,-51.6603553995285,910.));
#274267=CARTESIAN_POINT('',(-49.8776446004719,-51.6603553995286,1282.35584962783));
#274268=CARTESIAN_POINT('',(-49.8776446004719,-51.6603553995285,910.));
#274269=CARTESIAN_POINT('',(-45.9014446004721,-51.6603553995287,1282.35584962783));
#274270=CARTESIAN_POINT('',(-49.8776446004719,-51.6603553995286,1282.35584962783));
#274271=CARTESIAN_POINT('',(-45.901444600472,-51.6603553995286,910.));
#274272=CARTESIAN_POINT('Origin',(-49.8776446004718,-49.8603553995285,910.));
#274273=CARTESIAN_POINT('',(-51.6776446004719,-49.8603553995284,1282.35584962783));
#274274=CARTESIAN_POINT('',(-51.6776446004718,-49.8603553995285,910.));
#274275=CARTESIAN_POINT('Origin',(-49.8776446004719,-49.8603553995286,1282.35584962783));
#274276=CARTESIAN_POINT('Origin',(-51.6776446004718,-45.8841553995287,910.));
#274277=CARTESIAN_POINT('',(-51.6776446004719,-45.8841553995285,1282.35584962783));
#274278=CARTESIAN_POINT('',(-51.6776446004718,-45.8841553995287,910.));
#274279=CARTESIAN_POINT('',(-51.6776446004719,-45.8841553995287,1282.35584962783));
#274280=CARTESIAN_POINT('Origin',(-49.8776446004718,-45.8841553995287,910.));
#274281=CARTESIAN_POINT('',(-49.8776446004717,-44.0841553995288,1282.35584962783));
#274282=CARTESIAN_POINT('',(-49.8776446004718,-44.0841553995287,910.));
#274283=CARTESIAN_POINT('Origin',(-49.8776446004719,-45.8841553995288,1282.35584962783));
#274284=CARTESIAN_POINT('Origin',(-45.9014446004719,-44.0841553995287,910.));
#274285=CARTESIAN_POINT('',(-45.9014446004717,-44.0841553995288,1282.35584962783));
#274286=CARTESIAN_POINT('',(-45.9014446004719,-44.0841553995287,910.));
#274287=CARTESIAN_POINT('',(-45.9014446004719,-44.0841553995288,1282.35584962783));
#274288=CARTESIAN_POINT('Origin',(-45.901444600472,-45.8841553995287,910.));
#274289=CARTESIAN_POINT('',(-44.101444600472,-45.8841553995288,1282.35584962783));
#274290=CARTESIAN_POINT('',(-44.101444600472,-45.8841553995288,910.));
#274291=CARTESIAN_POINT('Origin',(-45.901444600472,-45.8841553995288,1282.35584962783));
#274292=CARTESIAN_POINT('Origin',(-44.101444600472,-49.8603553995286,910.));
#274293=CARTESIAN_POINT('',(-44.1014446004721,-49.8603553995286,1282.35584962783));
#274294=CARTESIAN_POINT('',(-44.101444600472,-49.8603553995286,910.));
#274295=CARTESIAN_POINT('',(-44.1014446004721,-49.8603553995286,1282.35584962783));
#274296=CARTESIAN_POINT('Origin',(-45.901444600472,-49.8603553995286,910.));
#274297=CARTESIAN_POINT('Origin',(-45.9014446004721,-49.8603553995287,1282.35584962783));
#274298=CARTESIAN_POINT('Origin',(0.,0.,1282.35584962783));
#274299=CARTESIAN_POINT('Origin',(0.,0.,1282.35584962783));
#274300=CARTESIAN_POINT('',(-48.3386446004713,-7.56935539952863,1282.35584962783));
#274301=CARTESIAN_POINT('',(-51.0386446004713,-4.8693553995284,1282.35584962783));
#274302=CARTESIAN_POINT('Origin',(-48.3386446004713,-4.86935539952863,1282.35584962783));
#274303=CARTESIAN_POINT('',(-51.0386446004713,4.88664460047119,1282.35584962783));
#274304=CARTESIAN_POINT('',(-51.0386446004713,4.88664460047119,1282.35584962783));
#274305=CARTESIAN_POINT('',(-48.3386446004713,7.58664460047119,1282.35584962783));
#274306=CARTESIAN_POINT('Origin',(-48.3386446004713,4.88664460047119,1282.35584962783));
#274307=CARTESIAN_POINT('',(-44.2652173270483,7.58664460047119,1282.35584962783));
#274308=CARTESIAN_POINT('',(-48.3386446004713,7.58664460047119,1282.35584962783));
#274309=CARTESIAN_POINT('',(-42.3560290178447,8.37745629126751,1282.35584962783));
#274310=CARTESIAN_POINT('Origin',(-44.2652173270483,10.2866446004712,1282.35584962783));
#274311=CARTESIAN_POINT('',(-35.3156523994373,15.4178329096749,1282.35584962783));
#274312=CARTESIAN_POINT('',(-42.3560290178447,8.37745629126751,1282.35584962783));
#274313=CARTESIAN_POINT('',(-33.4064640902336,16.2086446004712,1282.35584962783));
#274314=CARTESIAN_POINT('Origin',(-33.4064640902336,13.5086446004712,1282.35584962783));
#274315=CARTESIAN_POINT('',(-20.7806446004713,16.2086446004712,1282.35584962783));
#274316=CARTESIAN_POINT('',(-27.0086446004713,16.2086446004712,1282.35584962783));
#274317=CARTESIAN_POINT('',(-16.2086446004713,20.7806446004712,1282.35584962783));
#274318=CARTESIAN_POINT('',(-20.7806446004713,16.2086446004712,1282.35584962783));
#274319=CARTESIAN_POINT('',(-16.2086446004713,33.4064640902334,1282.35584962783));
#274320=CARTESIAN_POINT('',(-16.2086446004713,33.4064640902334,1282.35584962783));
#274321=CARTESIAN_POINT('',(-15.4178329096749,35.3156523994371,1282.35584962783));
#274322=CARTESIAN_POINT('Origin',(-13.5086446004713,33.4064640902334,1282.35584962783));
#274323=CARTESIAN_POINT('',(-8.37745629126753,42.3560290178444,1282.35584962783));
#274324=CARTESIAN_POINT('',(-8.37745629126753,42.3560290178444,1282.35584962783));
#274325=CARTESIAN_POINT('',(-7.58664460047119,44.2652173270481,1282.35584962783));
#274326=CARTESIAN_POINT('Origin',(-10.2866446004712,44.2652173270481,1282.35584962783));
#274327=CARTESIAN_POINT('',(-7.58664460047116,48.338644600471,1282.35584962783));
#274328=CARTESIAN_POINT('',(-7.58664460047116,48.338644600471,1282.35584962783));
#274329=CARTESIAN_POINT('',(-4.88664460047113,51.038644600471,1282.35584962783));
#274330=CARTESIAN_POINT('Origin',(-4.88664460047115,48.338644600471,1282.35584962783));
#274331=CARTESIAN_POINT('',(4.86935539952935,51.0386446004711,1282.35584962783));
#274332=CARTESIAN_POINT('',(-4.88664460047113,51.038644600471,1282.35584962783));
#274333=CARTESIAN_POINT('',(7.56935539952934,48.3386446004711,1282.35584962783));
#274334=CARTESIAN_POINT('Origin',(4.86935539952934,48.3386446004711,1282.35584962783));
#274335=CARTESIAN_POINT('',(7.56935539952933,44.2652173270481,1282.35584962783));
#274336=CARTESIAN_POINT('',(7.56935539952934,48.3386446004712,1282.35584962783));
#274337=CARTESIAN_POINT('',(8.36016709032564,42.3560290178444,1282.35584962783));
#274338=CARTESIAN_POINT('Origin',(10.2693553995293,44.2652173270481,1282.35584962783));
#274339=CARTESIAN_POINT('',(15.400543708733,35.315652399437,1282.35584962783));
#274340=CARTESIAN_POINT('',(8.36016709032557,42.3560290178445,1282.35584962783));
#274341=CARTESIAN_POINT('',(16.1913553995293,33.4064640902334,1282.35584962783));
#274342=CARTESIAN_POINT('Origin',(13.4913553995293,33.4064640902334,1282.35584962783));
#274343=CARTESIAN_POINT('',(16.1913553995292,20.7806446004711,1282.35584962783));
#274344=CARTESIAN_POINT('',(16.1913553995293,27.0086446004711,1282.35584962783));
#274345=CARTESIAN_POINT('',(20.7633553995292,16.208644600471,1282.35584962783));
#274346=CARTESIAN_POINT('',(16.1913553995292,20.7806446004711,1282.35584962783));
#274347=CARTESIAN_POINT('',(33.3891748892915,16.2086446004709,1282.35584962783));
#274348=CARTESIAN_POINT('',(33.3891748892914,16.2086446004709,1282.35584962783));
#274349=CARTESIAN_POINT('',(35.2983631984951,15.4178329096746,1282.35584962783));
#274350=CARTESIAN_POINT('Origin',(33.3891748892914,13.508644600471,1282.35584962783));
#274351=CARTESIAN_POINT('',(42.3387398169024,8.37745629126718,1282.35584962783));
#274352=CARTESIAN_POINT('',(42.3387398169023,8.37745629126725,1282.35584962783));
#274353=CARTESIAN_POINT('',(44.2479281261061,7.58664460047083,1282.35584962783));
#274354=CARTESIAN_POINT('Origin',(44.2479281261061,10.2866446004708,1282.35584962783));
#274355=CARTESIAN_POINT('',(48.321355399529,7.58664460047079,1282.35584962783));
#274356=CARTESIAN_POINT('',(48.321355399529,7.58664460047079,1282.35584962783));
#274357=CARTESIAN_POINT('',(51.021355399529,4.88664460047075,1282.35584962783));
#274358=CARTESIAN_POINT('Origin',(48.321355399529,4.88664460047079,1282.35584962783));
#274359=CARTESIAN_POINT('',(51.0213553995291,-4.86935539952937,1282.35584962783));
#274360=CARTESIAN_POINT('',(51.021355399529,4.88664460047082,1282.35584962783));
#274361=CARTESIAN_POINT('',(48.3213553995291,-7.56935539952937,1282.35584962783));
#274362=CARTESIAN_POINT('Origin',(48.3213553995291,-4.86935539952937,1282.35584962783));
#274363=CARTESIAN_POINT('',(44.2479281261061,-7.56935539952937,1282.35584962783));
#274364=CARTESIAN_POINT('',(48.3213553995291,-7.56935539952937,1282.35584962783));
#274365=CARTESIAN_POINT('',(42.3387398169024,-8.36016709032569,1282.35584962783));
#274366=CARTESIAN_POINT('Origin',(44.2479281261061,-10.2693553995294,1282.35584962783));
#274367=CARTESIAN_POINT('',(35.2983631984951,-15.400543708733,1282.35584962783));
#274368=CARTESIAN_POINT('',(42.3387398169025,-8.36016709032562,1282.35584962783));
#274369=CARTESIAN_POINT('',(33.3891748892914,-16.1913553995294,1282.35584962783));
#274370=CARTESIAN_POINT('Origin',(33.3891748892914,-13.4913553995294,1282.35584962783));
#274371=CARTESIAN_POINT('',(20.7633553995291,-16.1913553995294,1282.35584962783));
#274372=CARTESIAN_POINT('',(26.9913553995291,-16.1913553995294,1282.35584962783));
#274373=CARTESIAN_POINT('',(16.1913553995291,-20.7633553995294,1282.35584962783));
#274374=CARTESIAN_POINT('',(20.7633553995292,-16.1913553995293,1282.35584962783));
#274375=CARTESIAN_POINT('',(16.191355399529,-33.3891748892916,1282.35584962783));
#274376=CARTESIAN_POINT('',(16.191355399529,-33.3891748892915,1282.35584962783));
#274377=CARTESIAN_POINT('',(15.4005437087327,-35.2983631984953,1282.35584962783));
#274378=CARTESIAN_POINT('Origin',(13.491355399529,-33.3891748892916,1282.35584962783));
#274379=CARTESIAN_POINT('',(8.36016709032531,-42.3387398169026,1282.35584962783));
#274380=CARTESIAN_POINT('',(8.36016709032537,-42.3387398169025,1282.35584962783));
#274381=CARTESIAN_POINT('',(7.56935539952897,-44.2479281261063,1282.35584962783));
#274382=CARTESIAN_POINT('Origin',(10.269355399529,-44.2479281261063,1282.35584962783));
#274383=CARTESIAN_POINT('',(7.56935539952894,-48.3213553995292,1282.35584962783));
#274384=CARTESIAN_POINT('',(7.56935539952894,-48.3213553995291,1282.35584962783));
#274385=CARTESIAN_POINT('',(4.86935539952891,-51.0213553995292,1282.35584962783));
#274386=CARTESIAN_POINT('Origin',(4.86935539952893,-48.3213553995292,1282.35584962783));
#274387=CARTESIAN_POINT('',(-4.88664460047193,-51.0213553995292,1282.35584962783));
#274388=CARTESIAN_POINT('',(4.86935539952891,-51.0213553995292,1282.35584962783));
#274389=CARTESIAN_POINT('',(-7.5866446004719,-48.3213553995292,1282.35584962783));
#274390=CARTESIAN_POINT('Origin',(-4.8866446004719,-48.3213553995292,1282.35584962783));
#274391=CARTESIAN_POINT('',(-7.58664460047186,-44.2479281261062,1282.35584962783));
#274392=CARTESIAN_POINT('',(-7.5866446004719,-48.3213553995291,1282.35584962783));
#274393=CARTESIAN_POINT('',(-8.37745629126815,-42.3387398169026,1282.35584962783));
#274394=CARTESIAN_POINT('Origin',(-10.2866446004719,-44.2479281261062,1282.35584962783));
#274395=CARTESIAN_POINT('',(-15.4178329096754,-35.2983631984951,1282.35584962783));
#274396=CARTESIAN_POINT('',(-8.37745629126815,-42.3387398169026,1282.35584962783));
#274397=CARTESIAN_POINT('',(-16.2086446004717,-33.3891748892914,1282.35584962783));
#274398=CARTESIAN_POINT('Origin',(-13.5086446004717,-33.3891748892915,1282.35584962783));
#274399=CARTESIAN_POINT('',(-16.2086446004716,-20.7633553995291,1282.35584962783));
#274400=CARTESIAN_POINT('',(-16.2086446004717,-26.9913553995291,1282.35584962783));
#274401=CARTESIAN_POINT('',(-20.7806446004716,-16.1913553995291,1282.35584962783));
#274402=CARTESIAN_POINT('',(-16.2086446004716,-20.7633553995291,1282.35584962783));
#274403=CARTESIAN_POINT('',(-33.4064640902338,-16.1913553995289,1282.35584962783));
#274404=CARTESIAN_POINT('',(-33.4064640902337,-16.1913553995289,1282.35584962783));
#274405=CARTESIAN_POINT('',(-35.3156523994374,-15.4005437087325,1282.35584962783));
#274406=CARTESIAN_POINT('Origin',(-33.4064640902337,-13.4913553995289,1282.35584962783));
#274407=CARTESIAN_POINT('',(-42.3560290178447,-8.36016709032506,1282.35584962783));
#274408=CARTESIAN_POINT('',(-42.3560290178447,-8.36016709032506,1282.35584962783));
#274409=CARTESIAN_POINT('',(-44.2652173270483,-7.5693553995287,1282.35584962783));
#274410=CARTESIAN_POINT('Origin',(-44.2652173270484,-10.2693553995287,1282.35584962783));
#274411=CARTESIAN_POINT('',(-48.3386446004712,-7.56935539952863,1282.35584962783));
#274412=CARTESIAN_POINT('Origin',(0.,0.,-260.));
#274413=CARTESIAN_POINT('',(-51.0386446004713,4.88664460047119,-260.));
#274414=CARTESIAN_POINT('',(-48.3386446004713,7.58664460047119,-260.));
#274415=CARTESIAN_POINT('Origin',(-48.3386446004713,4.88664460047119,-260.));
#274416=CARTESIAN_POINT('',(-51.038644600471,-4.86935539952829,-260.));
#274417=CARTESIAN_POINT('',(-51.0386446004713,4.88664460047119,-260.));
#274418=CARTESIAN_POINT('',(-48.338644600471,-7.56935539952835,-260.));
#274419=CARTESIAN_POINT('Origin',(-48.338644600471,-4.86935539952834,-260.));
#274420=CARTESIAN_POINT('',(-44.2652173270481,-7.56935539952842,-260.));
#274421=CARTESIAN_POINT('',(-48.338644600471,-7.56935539952835,-260.));
#274422=CARTESIAN_POINT('',(-42.3560290178444,-8.36016709032478,-260.));
#274423=CARTESIAN_POINT('Origin',(-44.2652173270481,-10.2693553995284,-260.));
#274424=CARTESIAN_POINT('',(-35.3156523994372,-15.4005437087323,-260.));
#274425=CARTESIAN_POINT('',(-42.3560290178444,-8.36016709032478,-260.));
#274426=CARTESIAN_POINT('',(-33.4064640902335,-16.1913553995286,-260.));
#274427=CARTESIAN_POINT('Origin',(-33.4064640902334,-13.4913553995286,-260.));
#274428=CARTESIAN_POINT('',(-20.7806446004713,-16.1913553995288,-260.));
#274429=CARTESIAN_POINT('',(-33.4064640902335,-16.1913553995286,-260.));
#274430=CARTESIAN_POINT('',(-16.2086446004713,-20.7633553995288,-260.));
#274431=CARTESIAN_POINT('',(-16.2086446004713,-20.7633553995288,-260.));
#274432=CARTESIAN_POINT('',(-16.2086446004715,-33.3891748892914,-260.));
#274433=CARTESIAN_POINT('',(-16.2086446004714,-26.9913553995288,-260.));
#274434=CARTESIAN_POINT('',(-15.4178329096752,-35.2983631984948,-260.));
#274435=CARTESIAN_POINT('Origin',(-13.5086446004715,-33.3891748892912,-260.));
#274436=CARTESIAN_POINT('',(-8.37745629126787,-42.3387398169023,-260.));
#274437=CARTESIAN_POINT('',(-8.37745629126787,-42.3387398169023,-260.));
#274438=CARTESIAN_POINT('',(-7.58664460047157,-44.247928126106,-260.));
#274439=CARTESIAN_POINT('Origin',(-10.2866446004716,-44.2479281261059,-260.));
#274440=CARTESIAN_POINT('',(-7.58664460047161,-48.3213553995291,-260.));
#274441=CARTESIAN_POINT('',(-7.58664460047161,-48.3213553995289,-260.));
#274442=CARTESIAN_POINT('',(-4.88664460047164,-51.021355399529,-260.));
#274443=CARTESIAN_POINT('Origin',(-4.88664460047161,-48.321355399529,-260.));
#274444=CARTESIAN_POINT('',(4.86935539952891,-51.0213553995286,-260.));
#274445=CARTESIAN_POINT('',(4.86935539952891,-51.0213553995286,-260.));
#274446=CARTESIAN_POINT('',(7.56935539952894,-48.3213553995286,-260.));
#274447=CARTESIAN_POINT('Origin',(4.86935539952893,-48.3213553995286,-260.));
#274448=CARTESIAN_POINT('',(7.56935539952897,-44.2479281261057,-260.));
#274449=CARTESIAN_POINT('',(7.56935539952894,-48.3213553995286,-260.));
#274450=CARTESIAN_POINT('',(8.36016709032531,-42.338739816902,-260.));
#274451=CARTESIAN_POINT('Origin',(10.269355399529,-44.2479281261057,-260.));
#274452=CARTESIAN_POINT('',(15.4005437087327,-35.2983631984947,-260.));
#274453=CARTESIAN_POINT('',(8.36016709032531,-42.338739816902,-260.));
#274454=CARTESIAN_POINT('',(16.191355399529,-33.389174889291,-260.));
#274455=CARTESIAN_POINT('Origin',(13.491355399529,-33.389174889291,-260.));
#274456=CARTESIAN_POINT('',(16.1913553995291,-20.7633553995288,-260.));
#274457=CARTESIAN_POINT('',(16.191355399529,-33.389174889291,-260.));
#274458=CARTESIAN_POINT('',(20.7633553995291,-16.1913553995288,-260.));
#274459=CARTESIAN_POINT('',(20.7633553995291,-16.1913553995288,-260.));
#274460=CARTESIAN_POINT('',(33.3891748892914,-16.1913553995288,-260.));
#274461=CARTESIAN_POINT('',(26.9913553995291,-16.1913553995288,-260.));
#274462=CARTESIAN_POINT('',(35.2983631984951,-15.4005437087325,-260.));
#274463=CARTESIAN_POINT('Origin',(33.3891748892914,-13.4913553995288,-260.));
#274464=CARTESIAN_POINT('',(42.3387398169024,-8.36016709032512,-260.));
#274465=CARTESIAN_POINT('',(42.3387398169024,-8.36016709032512,-260.));
#274466=CARTESIAN_POINT('',(44.2479281261061,-7.5693553995288,-260.));
#274467=CARTESIAN_POINT('Origin',(44.2479281261061,-10.2693553995288,-260.));
#274468=CARTESIAN_POINT('',(48.3213553995291,-7.5693553995288,-260.));
#274469=CARTESIAN_POINT('',(48.3213553995291,-7.5693553995288,-260.));
#274470=CARTESIAN_POINT('',(51.0213553995291,-4.8693553995288,-260.));
#274471=CARTESIAN_POINT('Origin',(48.3213553995291,-4.8693553995288,-260.));
#274472=CARTESIAN_POINT('',(51.0213553995287,4.88664460047104,-260.));
#274473=CARTESIAN_POINT('',(51.0213553995287,4.88664460047104,-260.));
#274474=CARTESIAN_POINT('',(48.3213553995288,7.58664460047108,-260.));
#274475=CARTESIAN_POINT('Origin',(48.3213553995287,4.88664460047107,-260.));
#274476=CARTESIAN_POINT('',(44.2479281261058,7.58664460047112,-260.));
#274477=CARTESIAN_POINT('',(48.3213553995288,7.58664460047107,-260.));
#274478=CARTESIAN_POINT('',(42.3387398169021,8.37745629126746,-260.));
#274479=CARTESIAN_POINT('Origin',(44.2479281261058,10.2866446004711,-260.));
#274480=CARTESIAN_POINT('',(35.2983631984948,15.4178329096749,-260.));
#274481=CARTESIAN_POINT('',(42.3387398169021,8.37745629126746,-260.));
#274482=CARTESIAN_POINT('',(33.3891748892912,16.2086446004712,-260.));
#274483=CARTESIAN_POINT('Origin',(33.3891748892911,13.5086446004712,-260.));
#274484=CARTESIAN_POINT('',(20.7633553995289,16.2086446004714,-260.));
#274485=CARTESIAN_POINT('',(33.3891748892912,16.2086446004712,-260.));
#274486=CARTESIAN_POINT('',(16.191355399529,20.7806446004713,-260.));
#274487=CARTESIAN_POINT('',(16.191355399529,20.7806446004713,-260.));
#274488=CARTESIAN_POINT('',(16.191355399529,33.4064640902336,-260.));
#274489=CARTESIAN_POINT('',(16.191355399529,27.0086446004713,-260.));
#274490=CARTESIAN_POINT('',(15.4005437087327,35.3156523994373,-260.));
#274491=CARTESIAN_POINT('Origin',(13.491355399529,33.4064640902337,-260.));
#274492=CARTESIAN_POINT('',(8.36016709032535,42.3560290178447,-260.));
#274493=CARTESIAN_POINT('',(8.36016709032535,42.3560290178447,-260.));
#274494=CARTESIAN_POINT('',(7.56935539952904,44.2652173270484,-260.));
#274495=CARTESIAN_POINT('Origin',(10.269355399529,44.2652173270484,-260.));
#274496=CARTESIAN_POINT('',(7.56935539952906,48.3386446004714,-260.));
#274497=CARTESIAN_POINT('',(7.56935539952906,48.3386446004714,-260.));
#274498=CARTESIAN_POINT('',(4.86935539952906,51.0386446004714,-260.));
#274499=CARTESIAN_POINT('Origin',(4.86935539952905,48.3386446004714,-260.));
#274500=CARTESIAN_POINT('',(-4.88664460047113,51.038644600471,-260.));
#274501=CARTESIAN_POINT('',(-4.88664460047113,51.038644600471,-260.));
#274502=CARTESIAN_POINT('',(-7.58664460047116,48.338644600471,-260.));
#274503=CARTESIAN_POINT('Origin',(-4.88664460047115,48.338644600471,-260.));
#274504=CARTESIAN_POINT('',(-7.58664460047119,44.2652173270481,-260.));
#274505=CARTESIAN_POINT('',(-7.58664460047116,48.338644600471,-260.));
#274506=CARTESIAN_POINT('',(-8.37745629126753,42.3560290178444,-260.));
#274507=CARTESIAN_POINT('Origin',(-10.2866446004712,44.2652173270481,-260.));
#274508=CARTESIAN_POINT('',(-15.4178329096749,35.3156523994371,-260.));
#274509=CARTESIAN_POINT('',(-8.37745629126753,42.3560290178444,-260.));
#274510=CARTESIAN_POINT('',(-16.2086446004713,33.4064640902334,-260.));
#274511=CARTESIAN_POINT('Origin',(-13.5086446004713,33.4064640902334,-260.));
#274512=CARTESIAN_POINT('',(-16.2086446004714,20.7806446004712,-260.));
#274513=CARTESIAN_POINT('',(-16.2086446004713,33.4064640902334,-260.));
#274514=CARTESIAN_POINT('',(-20.7806446004713,16.2086446004712,-260.));
#274515=CARTESIAN_POINT('',(-20.7806446004713,16.2086446004712,-260.));
#274516=CARTESIAN_POINT('',(-33.4064640902336,16.2086446004712,-260.));
#274517=CARTESIAN_POINT('',(-27.0086446004713,16.2086446004712,-260.));
#274518=CARTESIAN_POINT('',(-35.3156523994373,15.4178329096749,-260.));
#274519=CARTESIAN_POINT('Origin',(-33.4064640902336,13.5086446004712,-260.));
#274520=CARTESIAN_POINT('',(-42.3560290178447,8.37745629126751,-260.));
#274521=CARTESIAN_POINT('',(-42.3560290178447,8.37745629126751,-260.));
#274522=CARTESIAN_POINT('',(-44.2652173270483,7.58664460047119,-260.));
#274523=CARTESIAN_POINT('Origin',(-44.2652173270483,10.2866446004712,-260.));
#274524=CARTESIAN_POINT('',(-48.3386446004713,7.58664460047119,-260.));
#274525=CARTESIAN_POINT('Origin',(-48.3386446004712,-4.86935539952856,910.));
#274526=CARTESIAN_POINT('',(-48.3386446004712,-7.56935539952856,910.));
#274527=CARTESIAN_POINT('',(-51.0386446004712,-4.8693553995285,910.));
#274528=CARTESIAN_POINT('Origin',(-48.3386446004712,-7.56935539952856,910.));
#274529=CARTESIAN_POINT('',(-44.2652173270483,-7.56935539952864,910.));
#274530=CARTESIAN_POINT('Origin',(-44.2652173270483,-10.2693553995286,910.));
#274531=CARTESIAN_POINT('',(-42.3560290178446,-8.36016709032499,910.));
#274532=CARTESIAN_POINT('Origin',(-42.3560290178446,-8.36016709032499,910.));
#274533=CARTESIAN_POINT('',(-35.3156523994374,-15.4005437087325,910.));
#274534=CARTESIAN_POINT('Origin',(-33.4064640902337,-13.4913553995288,910.));
#274535=CARTESIAN_POINT('',(-33.4064640902337,-16.1913553995288,910.));
#274536=CARTESIAN_POINT('Origin',(-33.4064640902337,-16.1913553995288,910.));
#274537=CARTESIAN_POINT('',(-20.7806446004715,-16.191355399529,910.));
#274538=CARTESIAN_POINT('Origin',(-16.2086446004715,-20.7633553995291,910.));
#274539=CARTESIAN_POINT('',(-16.2086446004715,-20.7633553995291,910.));
#274540=CARTESIAN_POINT('Origin',(-16.2086446004716,-26.9913553995291,910.));
#274541=CARTESIAN_POINT('',(-16.2086446004717,-33.3891748892914,910.));
#274542=CARTESIAN_POINT('Origin',(-13.5086446004717,-33.3891748892914,910.));
#274543=CARTESIAN_POINT('',(-15.4178329096754,-35.298363198495,910.));
#274544=CARTESIAN_POINT('Origin',(-8.37745629126809,-42.3387398169025,910.));
#274545=CARTESIAN_POINT('',(-8.37745629126808,-42.3387398169025,910.));
#274546=CARTESIAN_POINT('Origin',(-10.2866446004718,-44.2479281261061,910.));
#274547=CARTESIAN_POINT('',(-7.58664460047179,-44.2479281261062,910.));
#274548=CARTESIAN_POINT('Origin',(-7.58664460047183,-48.3213553995291,910.));
#274549=CARTESIAN_POINT('',(-7.58664460047183,-48.3213553995291,910.));
#274550=CARTESIAN_POINT('Origin',(-4.88664460047183,-48.3213553995292,910.));
#274551=CARTESIAN_POINT('',(-4.88664460047186,-51.0213553995292,910.));
#274552=CARTESIAN_POINT('Origin',(4.86935539952891,-51.021355399529,910.));
#274553=CARTESIAN_POINT('',(4.86935539952891,-51.021355399529,910.));
#274554=CARTESIAN_POINT('Origin',(4.86935539952893,-48.3213553995291,910.));
#274555=CARTESIAN_POINT('',(7.56935539952894,-48.3213553995291,910.));
#274556=CARTESIAN_POINT('Origin',(7.56935539952894,-48.3213553995291,910.));
#274557=CARTESIAN_POINT('',(7.56935539952897,-44.2479281261061,910.));
#274558=CARTESIAN_POINT('Origin',(10.269355399529,-44.2479281261061,910.));
#274559=CARTESIAN_POINT('',(8.36016709032531,-42.3387398169024,910.));
#274560=CARTESIAN_POINT('Origin',(8.36016709032531,-42.3387398169024,910.));
#274561=CARTESIAN_POINT('',(15.4005437087327,-35.2983631984951,910.));
#274562=CARTESIAN_POINT('Origin',(13.491355399529,-33.3891748892914,910.));
#274563=CARTESIAN_POINT('',(16.191355399529,-33.3891748892915,910.));
#274564=CARTESIAN_POINT('Origin',(16.191355399529,-33.3891748892915,910.));
#274565=CARTESIAN_POINT('',(16.1913553995291,-20.7633553995292,910.));
#274566=CARTESIAN_POINT('Origin',(20.7633553995291,-16.1913553995292,910.));
#274567=CARTESIAN_POINT('',(20.7633553995291,-16.1913553995292,910.));
#274568=CARTESIAN_POINT('Origin',(26.9913553995291,-16.1913553995292,910.));
#274569=CARTESIAN_POINT('',(33.3891748892914,-16.1913553995292,910.));
#274570=CARTESIAN_POINT('Origin',(33.3891748892914,-13.4913553995292,910.));
#274571=CARTESIAN_POINT('',(35.2983631984951,-15.4005437087329,910.));
#274572=CARTESIAN_POINT('Origin',(42.3387398169024,-8.36016709032555,910.));
#274573=CARTESIAN_POINT('',(42.3387398169024,-8.36016709032555,910.));
#274574=CARTESIAN_POINT('Origin',(44.2479281261061,-10.2693553995292,910.));
#274575=CARTESIAN_POINT('',(44.2479281261061,-7.56935539952923,910.));
#274576=CARTESIAN_POINT('Origin',(48.3213553995291,-7.56935539952923,910.));
#274577=CARTESIAN_POINT('',(48.3213553995291,-7.56935539952923,910.));
#274578=CARTESIAN_POINT('Origin',(48.3213553995291,-4.86935539952923,910.));
#274579=CARTESIAN_POINT('',(51.0213553995291,-4.86935539952923,910.));
#274580=CARTESIAN_POINT('Origin',(51.0213553995289,4.88664460047082,910.));
#274581=CARTESIAN_POINT('',(51.0213553995289,4.88664460047082,910.));
#274582=CARTESIAN_POINT('Origin',(48.3213553995289,4.88664460047086,910.));
#274583=CARTESIAN_POINT('',(48.321355399529,7.58664460047086,910.));
#274584=CARTESIAN_POINT('Origin',(48.321355399529,7.58664460047086,910.));
#274585=CARTESIAN_POINT('',(44.247928126106,7.5866446004709,910.));
#274586=CARTESIAN_POINT('Origin',(44.247928126106,10.2866446004709,910.));
#274587=CARTESIAN_POINT('',(42.3387398169023,8.37745629126725,910.));
#274588=CARTESIAN_POINT('Origin',(42.3387398169023,8.37745629126725,910.));
#274589=CARTESIAN_POINT('',(35.298363198495,15.4178329096747,910.));
#274590=CARTESIAN_POINT('Origin',(33.3891748892913,13.508644600471,910.));
#274591=CARTESIAN_POINT('',(33.3891748892914,16.208644600471,910.));
#274592=CARTESIAN_POINT('Origin',(33.3891748892914,16.208644600471,910.));
#274593=CARTESIAN_POINT('',(20.7633553995292,16.2086446004711,910.));
#274594=CARTESIAN_POINT('Origin',(16.1913553995292,20.7806446004711,910.));
#274595=CARTESIAN_POINT('',(16.1913553995292,20.7806446004711,910.));
#274596=CARTESIAN_POINT('Origin',(16.1913553995292,27.0086446004711,910.));
#274597=CARTESIAN_POINT('',(16.1913553995292,33.4064640902334,910.));
#274598=CARTESIAN_POINT('Origin',(13.4913553995292,33.4064640902334,910.));
#274599=CARTESIAN_POINT('',(15.4005437087329,35.3156523994371,910.));
#274600=CARTESIAN_POINT('Origin',(8.36016709032557,42.3560290178445,910.));
#274601=CARTESIAN_POINT('',(8.36016709032557,42.3560290178445,910.));
#274602=CARTESIAN_POINT('Origin',(10.2693553995293,44.2652173270482,910.));
#274603=CARTESIAN_POINT('',(7.56935539952926,44.2652173270482,910.));
#274604=CARTESIAN_POINT('Origin',(7.56935539952927,48.3386446004712,910.));
#274605=CARTESIAN_POINT('',(7.56935539952927,48.3386446004712,910.));
#274606=CARTESIAN_POINT('Origin',(4.86935539952927,48.3386446004712,910.));
#274607=CARTESIAN_POINT('',(4.86935539952928,51.0386446004712,910.));
#274608=CARTESIAN_POINT('Origin',(-4.88664460047113,51.038644600471,910.));
#274609=CARTESIAN_POINT('',(-4.88664460047113,51.038644600471,910.));
#274610=CARTESIAN_POINT('Origin',(-4.88664460047115,48.338644600471,910.));
#274611=CARTESIAN_POINT('',(-7.58664460047116,48.338644600471,910.));
#274612=CARTESIAN_POINT('Origin',(-7.58664460047116,48.338644600471,910.));
#274613=CARTESIAN_POINT('',(-7.58664460047119,44.2652173270481,910.));
#274614=CARTESIAN_POINT('Origin',(-10.2866446004712,44.2652173270481,910.));
#274615=CARTESIAN_POINT('',(-8.37745629126753,42.3560290178444,910.));
#274616=CARTESIAN_POINT('Origin',(-8.37745629126753,42.3560290178444,910.));
#274617=CARTESIAN_POINT('',(-15.4178329096749,35.3156523994371,910.));
#274618=CARTESIAN_POINT('Origin',(-13.5086446004713,33.4064640902334,910.));
#274619=CARTESIAN_POINT('',(-16.2086446004713,33.4064640902334,910.));
#274620=CARTESIAN_POINT('Origin',(-16.2086446004713,33.4064640902334,910.));
#274621=CARTESIAN_POINT('',(-16.2086446004713,20.7806446004712,910.));
#274622=CARTESIAN_POINT('Origin',(-20.7806446004713,16.2086446004712,910.));
#274623=CARTESIAN_POINT('',(-20.7806446004713,16.2086446004712,910.));
#274624=CARTESIAN_POINT('Origin',(-27.0086446004713,16.2086446004712,910.));
#274625=CARTESIAN_POINT('',(-33.4064640902336,16.2086446004712,910.));
#274626=CARTESIAN_POINT('Origin',(-33.4064640902336,13.5086446004712,910.));
#274627=CARTESIAN_POINT('',(-35.3156523994373,15.4178329096749,910.));
#274628=CARTESIAN_POINT('Origin',(-42.3560290178447,8.37745629126751,910.));
#274629=CARTESIAN_POINT('',(-42.3560290178447,8.37745629126751,910.));
#274630=CARTESIAN_POINT('Origin',(-44.2652173270483,10.2866446004712,910.));
#274631=CARTESIAN_POINT('',(-44.2652173270483,7.58664460047119,910.));
#274632=CARTESIAN_POINT('Origin',(-48.3386446004713,7.58664460047119,910.));
#274633=CARTESIAN_POINT('',(-48.3386446004713,7.58664460047119,910.));
#274634=CARTESIAN_POINT('Origin',(-48.3386446004713,4.88664460047119,910.));
#274635=CARTESIAN_POINT('',(-51.0386446004713,4.88664460047119,910.));
#274636=CARTESIAN_POINT('Origin',(-51.0386446004713,4.88664460047119,910.));
#274637=CARTESIAN_POINT('Origin',(26.9913553995291,-26.9913553995292,910.));
#274638=CARTESIAN_POINT('',(29.7492170880445,-21.3270638368519,1282.35584962783));
#274639=CARTESIAN_POINT('',(24.2334937110134,-21.327063836852,1282.35584962783));
#274640=CARTESIAN_POINT('Origin',(26.9913553995291,-26.9913553995294,1282.35584962783));
#274641=CARTESIAN_POINT('',(24.2334937110134,-21.3270638368515,-260.));
#274642=CARTESIAN_POINT('',(24.2334937110134,-21.3270638368519,910.));
#274643=CARTESIAN_POINT('',(29.7492170880447,-21.3270638368514,-260.));
#274644=CARTESIAN_POINT('Origin',(26.9913553995291,-26.9913553995288,-260.));
#274645=CARTESIAN_POINT('',(29.7492170880447,-21.3270638368519,910.));
#274646=CARTESIAN_POINT('Origin',(0.,0.,-260.));
#274647=CARTESIAN_POINT('',(32.6891089669786,-35.113778119667,-260.));
#274648=CARTESIAN_POINT('',(35.1137781196672,-32.6891089669784,-260.));
#274649=CARTESIAN_POINT('Origin',(26.9913553995291,-26.9913553995288,-260.));
#274650=CARTESIAN_POINT('',(32.6556469622064,-29.7492170880444,-260.));
#274651=CARTESIAN_POINT('',(35.1137781196672,-32.6891089669784,-260.));
#274652=CARTESIAN_POINT('',(32.6556469622064,-24.2334937110132,-260.));
#274653=CARTESIAN_POINT('Origin',(26.9913553995291,-26.9913553995288,-260.));
#274654=CARTESIAN_POINT('',(35.1137781196672,-21.2936018320792,-260.));
#274655=CARTESIAN_POINT('',(35.1137781196672,-21.2936018320792,-260.));
#274656=CARTESIAN_POINT('',(32.6891089669786,-18.8689326793906,-260.));
#274657=CARTESIAN_POINT('Origin',(26.9913553995291,-26.9913553995288,-260.));
#274658=CARTESIAN_POINT('',(32.6891089669786,-18.8689326793906,-260.));
#274659=CARTESIAN_POINT('',(21.2936018320795,-18.8689326793908,-260.));
#274660=CARTESIAN_POINT('',(21.2936018320795,-18.8689326793907,-260.));
#274661=CARTESIAN_POINT('',(18.8689326793909,-21.2936018320794,-260.));
#274662=CARTESIAN_POINT('Origin',(26.9913553995291,-26.9913553995288,-260.));
#274663=CARTESIAN_POINT('',(21.3270638368517,-24.2334937110133,-260.));
#274664=CARTESIAN_POINT('',(18.8689326793909,-21.2936018320794,-260.));
#274665=CARTESIAN_POINT('',(21.3270638368517,-29.7492170880443,-260.));
#274666=CARTESIAN_POINT('Origin',(26.9913553995291,-26.9913553995288,-260.));
#274667=CARTESIAN_POINT('',(18.8689326793909,-32.6891089669782,-260.));
#274668=CARTESIAN_POINT('',(18.8689326793909,-32.6891089669782,-260.));
#274669=CARTESIAN_POINT('',(21.2936018320795,-35.1137781196669,-260.));
#274670=CARTESIAN_POINT('Origin',(26.9913553995291,-26.9913553995288,-260.));
#274671=CARTESIAN_POINT('',(24.2334937110134,-32.6556469622061,-260.));
#274672=CARTESIAN_POINT('',(21.2936018320795,-35.1137781196669,-260.));
#274673=CARTESIAN_POINT('',(29.7492170880447,-32.6556469622062,-260.));
#274674=CARTESIAN_POINT('Origin',(26.9913553995291,-26.9913553995288,-260.));
#274675=CARTESIAN_POINT('',(32.6891089669786,-35.113778119667,-260.));
#274676=CARTESIAN_POINT('Origin',(32.6891089669786,-35.1137781196674,910.));
#274677=CARTESIAN_POINT('',(29.7492170880447,-32.6556469622067,1282.35584962783));
#274678=CARTESIAN_POINT('',(29.7492170880447,-32.6556469622066,910.));
#274679=CARTESIAN_POINT('',(32.6891089669786,-35.1137781196675,1282.35584962783));
#274680=CARTESIAN_POINT('',(32.6891089669785,-35.1137781196675,1282.35584962783));
#274681=CARTESIAN_POINT('',(32.6891089669786,-35.1137781196674,910.));
#274682=CARTESIAN_POINT('Origin',(26.9913553995291,-26.9913553995292,910.));
#274683=CARTESIAN_POINT('',(24.2334937110133,-32.6556469622066,1282.35584962783));
#274684=CARTESIAN_POINT('',(24.2334937110134,-32.6556469622066,910.));
#274685=CARTESIAN_POINT('Origin',(26.9913553995291,-26.9913553995294,1282.35584962783));
#274686=CARTESIAN_POINT('Origin',(21.2936018320795,-35.1137781196673,910.));
#274687=CARTESIAN_POINT('',(21.2936018320795,-35.1137781196674,1282.35584962783));
#274688=CARTESIAN_POINT('',(21.2936018320795,-35.1137781196673,910.));
#274689=CARTESIAN_POINT('',(21.2936018320795,-35.1137781196674,1282.35584962783));
#274690=CARTESIAN_POINT('Origin',(26.9913553995291,-26.9913553995292,910.));
#274691=CARTESIAN_POINT('',(18.8689326793907,-32.6891089669786,1282.35584962783));
#274692=CARTESIAN_POINT('',(18.8689326793909,-32.6891089669787,910.));
#274693=CARTESIAN_POINT('Origin',(26.9913553995291,-26.9913553995294,1282.35584962783));
#274694=CARTESIAN_POINT('Origin',(18.8689326793909,-32.6891089669787,910.));
#274695=CARTESIAN_POINT('',(21.3270638368522,-29.7492170880443,1282.35584962783));
#274696=CARTESIAN_POINT('',(21.3270638368517,-29.7492170880447,910.));
#274697=CARTESIAN_POINT('',(18.868932679391,-32.6891089669787,1282.35584962783));
#274698=CARTESIAN_POINT('Origin',(26.9913553995291,-26.9913553995292,910.));
#274699=CARTESIAN_POINT('',(21.3270638368518,-24.2334937110136,1282.35584962783));
#274700=CARTESIAN_POINT('',(21.3270638368517,-24.2334937110137,910.));
#274701=CARTESIAN_POINT('Origin',(26.9913553995291,-26.9913553995294,1282.35584962783));
#274702=CARTESIAN_POINT('Origin',(18.8689326793909,-21.2936018320798,910.));
#274703=CARTESIAN_POINT('',(18.8689326793904,-21.2936018320794,1282.35584962783));
#274704=CARTESIAN_POINT('',(18.8689326793909,-21.2936018320798,910.));
#274705=CARTESIAN_POINT('',(18.8689326793908,-21.2936018320799,1282.35584962783));
#274706=CARTESIAN_POINT('Origin',(26.9913553995291,-26.9913553995292,910.));
#274707=CARTESIAN_POINT('',(21.2936018320796,-18.8689326793912,1282.35584962783));
#274708=CARTESIAN_POINT('',(21.2936018320795,-18.8689326793912,910.));
#274709=CARTESIAN_POINT('Origin',(26.9913553995291,-26.9913553995294,1282.35584962783));
#274710=CARTESIAN_POINT('Origin',(21.2936018320795,-18.8689326793912,910.));
#274711=CARTESIAN_POINT('',(21.2936018320794,-18.8689326793913,1282.35584962783));
#274712=CARTESIAN_POINT('Origin',(32.6891089669786,-18.8689326793911,910.));
#274713=CARTESIAN_POINT('',(32.6891089669786,-18.8689326793912,1282.35584962783));
#274714=CARTESIAN_POINT('',(32.6891089669786,-18.8689326793911,910.));
#274715=CARTESIAN_POINT('',(32.6891089669787,-18.8689326793912,1282.35584962783));
#274716=CARTESIAN_POINT('Origin',(26.9913553995291,-26.9913553995292,910.));
#274717=CARTESIAN_POINT('',(35.113778119667,-21.2936018320796,1282.35584962783));
#274718=CARTESIAN_POINT('',(35.1137781196672,-21.2936018320797,910.));
#274719=CARTESIAN_POINT('Origin',(26.9913553995291,-26.9913553995294,1282.35584962783));
#274720=CARTESIAN_POINT('Origin',(35.1137781196672,-21.2936018320797,910.));
#274721=CARTESIAN_POINT('',(32.6556469622065,-24.2334937110136,1282.35584962783));
#274722=CARTESIAN_POINT('',(32.6556469622064,-24.2334937110136,910.));
#274723=CARTESIAN_POINT('',(35.1137781196673,-21.2936018320797,1282.35584962783));
#274724=CARTESIAN_POINT('Origin',(26.9913553995291,-26.9913553995292,910.));
#274725=CARTESIAN_POINT('',(32.6556469622066,-29.7492170880447,1282.35584962783));
#274726=CARTESIAN_POINT('',(32.6556469622064,-29.7492170880448,910.));
#274727=CARTESIAN_POINT('Origin',(26.9913553995291,-26.9913553995294,1282.35584962783));
#274728=CARTESIAN_POINT('Origin',(35.1137781196672,-32.6891089669788,910.));
#274729=CARTESIAN_POINT('',(35.1137781196671,-32.6891089669788,1282.35584962783));
#274730=CARTESIAN_POINT('',(35.1137781196672,-32.6891089669788,910.));
#274731=CARTESIAN_POINT('',(35.1137781196671,-32.6891089669788,1282.35584962783));
#274732=CARTESIAN_POINT('Origin',(26.9913553995291,-26.9913553995292,910.));
#274733=CARTESIAN_POINT('Origin',(26.9913553995291,-26.9913553995294,1282.35584962783));
#274734=CARTESIAN_POINT('Origin',(0.,0.,1282.35584962783));
#274735=CARTESIAN_POINT('Origin',(0.,0.,-260.));
#274736=CARTESIAN_POINT('',(51.6603553995289,-45.884155399529,-260.));
#274737=CARTESIAN_POINT('',(49.8603553995289,-44.084155399529,-260.));
#274738=CARTESIAN_POINT('Origin',(49.8603553995289,-45.884155399529,-260.));
#274739=CARTESIAN_POINT('',(45.8841553995291,-44.084155399529,-260.));
#274740=CARTESIAN_POINT('',(49.8603553995289,-44.084155399529,-260.));
#274741=CARTESIAN_POINT('',(44.0841553995291,-45.884155399529,-260.));
#274742=CARTESIAN_POINT('Origin',(45.8841553995291,-45.884155399529,-260.));
#274743=CARTESIAN_POINT('',(44.0841553995291,-49.8603553995288,-260.));
#274744=CARTESIAN_POINT('',(44.0841553995291,-45.884155399529,-260.));
#274745=CARTESIAN_POINT('',(45.8841553995291,-51.6603553995288,-260.));
#274746=CARTESIAN_POINT('Origin',(45.8841553995291,-49.8603553995288,-260.));
#274747=CARTESIAN_POINT('',(49.8603553995289,-51.6603553995288,-260.));
#274748=CARTESIAN_POINT('',(45.8841553995291,-51.6603553995288,-260.));
#274749=CARTESIAN_POINT('',(51.6603553995289,-49.8603553995288,-260.));
#274750=CARTESIAN_POINT('Origin',(49.8603553995289,-49.8603553995288,-260.));
#274751=CARTESIAN_POINT('',(51.6603553995289,-49.8603553995288,-260.));
#274752=CARTESIAN_POINT('Origin',(51.6603553995289,-49.8603553995292,910.));
#274753=CARTESIAN_POINT('',(51.6603553995289,-49.8603553995294,1282.35584962783));
#274754=CARTESIAN_POINT('',(51.6603553995289,-49.8603553995292,910.));
#274755=CARTESIAN_POINT('',(51.6603553995289,-45.8841553995295,1282.35584962783));
#274756=CARTESIAN_POINT('',(51.6603553995289,-49.8603553995292,1282.35584962783));
#274757=CARTESIAN_POINT('',(51.6603553995289,-45.8841553995294,910.));
#274758=CARTESIAN_POINT('Origin',(49.8603553995289,-49.8603553995292,910.));
#274759=CARTESIAN_POINT('',(49.8603553995289,-51.6603553995294,1282.35584962783));
#274760=CARTESIAN_POINT('',(49.8603553995289,-51.6603553995292,910.));
#274761=CARTESIAN_POINT('Origin',(49.8603553995289,-49.8603553995294,1282.35584962783));
#274762=CARTESIAN_POINT('Origin',(45.8841553995291,-51.6603553995292,910.));
#274763=CARTESIAN_POINT('',(45.8841553995291,-51.6603553995294,1282.35584962783));
#274764=CARTESIAN_POINT('',(45.8841553995291,-51.6603553995292,910.));
#274765=CARTESIAN_POINT('',(45.8841553995291,-51.6603553995294,1282.35584962783));
#274766=CARTESIAN_POINT('Origin',(45.8841553995291,-49.8603553995292,910.));
#274767=CARTESIAN_POINT('',(44.0841553995291,-49.860355399529,1282.35584962783));
#274768=CARTESIAN_POINT('',(44.0841553995291,-49.8603553995292,910.));
#274769=CARTESIAN_POINT('Origin',(45.8841553995291,-49.8603553995294,1282.35584962783));
#274770=CARTESIAN_POINT('Origin',(44.0841553995291,-45.8841553995294,910.));
#274771=CARTESIAN_POINT('',(44.0841553995291,-45.884155399529,1282.35584962783));
#274772=CARTESIAN_POINT('',(44.0841553995291,-45.8841553995294,910.));
#274773=CARTESIAN_POINT('',(44.0841553995291,-45.8841553995294,1282.35584962783));
#274774=CARTESIAN_POINT('Origin',(45.8841553995291,-45.8841553995294,910.));
#274775=CARTESIAN_POINT('',(45.8841553995291,-44.0841553995295,1282.35584962783));
#274776=CARTESIAN_POINT('',(45.8841553995291,-44.0841553995294,910.));
#274777=CARTESIAN_POINT('Origin',(45.8841553995291,-45.8841553995295,1282.35584962783));
#274778=CARTESIAN_POINT('Origin',(49.8603553995289,-44.0841553995294,910.));
#274779=CARTESIAN_POINT('',(49.8603553995289,-44.0841553995295,1282.35584962783));
#274780=CARTESIAN_POINT('',(49.8603553995289,-44.0841553995294,910.));
#274781=CARTESIAN_POINT('',(49.8603553995289,-44.0841553995295,1282.35584962783));
#274782=CARTESIAN_POINT('Origin',(49.8603553995289,-45.8841553995294,910.));
#274783=CARTESIAN_POINT('Origin',(49.8603553995289,-45.8841553995295,1282.35584962783));
#274784=CARTESIAN_POINT('Origin',(0.,0.,1282.35584962783));
#274785=CARTESIAN_POINT('Origin',(26.9913553995292,27.0086446004711,910.));
#274786=CARTESIAN_POINT('',(29.7492170880447,32.6729361631484,1282.35584962783));
#274787=CARTESIAN_POINT('',(24.2334937110136,32.6729361631484,1282.35584962783));
#274788=CARTESIAN_POINT('Origin',(26.9913553995293,27.008644600471,1282.35584962783));
#274789=CARTESIAN_POINT('',(24.2334937110134,32.6729361631487,-260.));
#274790=CARTESIAN_POINT('',(24.2334937110136,32.6729361631484,910.));
#274791=CARTESIAN_POINT('',(29.7492170880446,32.6729361631486,-260.));
#274792=CARTESIAN_POINT('Origin',(26.991355399529,27.0086446004713,-260.));
#274793=CARTESIAN_POINT('',(29.7492170880448,32.6729361631484,910.));
#274794=CARTESIAN_POINT('Origin',(0.,0.,-260.));
#274795=CARTESIAN_POINT('',(35.1137781196672,32.7063981679208,-260.));
#274796=CARTESIAN_POINT('',(32.6891089669786,35.1310673206094,-260.));
#274797=CARTESIAN_POINT('Origin',(26.991355399529,27.0086446004713,-260.));
#274798=CARTESIAN_POINT('',(32.6891089669786,35.1310673206094,-260.));
#274799=CARTESIAN_POINT('',(21.2936018320794,35.1310673206094,-260.));
#274800=CARTESIAN_POINT('',(21.2936018320794,35.1310673206094,-260.));
#274801=CARTESIAN_POINT('',(18.8689326793908,32.7063981679208,-260.));
#274802=CARTESIAN_POINT('Origin',(26.991355399529,27.0086446004713,-260.));
#274803=CARTESIAN_POINT('',(21.3270638368516,29.7665062889869,-260.));
#274804=CARTESIAN_POINT('',(18.8689326793908,32.7063981679208,-260.));
#274805=CARTESIAN_POINT('',(21.3270638368517,24.2507829119557,-260.));
#274806=CARTESIAN_POINT('Origin',(26.991355399529,27.0086446004713,-260.));
#274807=CARTESIAN_POINT('',(18.8689326793909,21.3108910330217,-260.));
#274808=CARTESIAN_POINT('',(18.8689326793909,21.3108910330217,-260.));
#274809=CARTESIAN_POINT('',(21.2936018320795,18.8862218803331,-260.));
#274810=CARTESIAN_POINT('Origin',(26.991355399529,27.0086446004713,-260.));
#274811=CARTESIAN_POINT('',(24.2334937110134,21.3443530377939,-260.));
#274812=CARTESIAN_POINT('',(21.2936018320795,18.8862218803331,-260.));
#274813=CARTESIAN_POINT('',(29.7492170880445,21.3443530377939,-260.));
#274814=CARTESIAN_POINT('Origin',(26.991355399529,27.0086446004713,-260.));
#274815=CARTESIAN_POINT('',(32.6891089669784,18.8862218803331,-260.));
#274816=CARTESIAN_POINT('',(32.6891089669784,18.8862218803331,-260.));
#274817=CARTESIAN_POINT('',(35.113778119667,21.3108910330217,-260.));
#274818=CARTESIAN_POINT('Origin',(26.991355399529,27.0086446004713,-260.));
#274819=CARTESIAN_POINT('',(32.6556469622063,24.2507829119556,-260.));
#274820=CARTESIAN_POINT('',(35.113778119667,21.3108910330217,-260.));
#274821=CARTESIAN_POINT('',(32.6556469622064,29.7665062889869,-260.));
#274822=CARTESIAN_POINT('Origin',(26.991355399529,27.0086446004713,-260.));
#274823=CARTESIAN_POINT('',(35.1137781196672,32.7063981679208,-260.));
#274824=CARTESIAN_POINT('Origin',(35.1137781196674,32.7063981679205,910.));
#274825=CARTESIAN_POINT('',(32.6556469622066,29.7665062889866,1282.35584962783));
#274826=CARTESIAN_POINT('',(32.6556469622066,29.7665062889866,910.));
#274827=CARTESIAN_POINT('',(35.1137781196674,32.7063981679205,1282.35584962783));
#274828=CARTESIAN_POINT('',(35.1137781196675,32.7063981679205,1282.35584962783));
#274829=CARTESIAN_POINT('',(35.1137781196674,32.7063981679205,910.));
#274830=CARTESIAN_POINT('Origin',(26.9913553995292,27.0086446004711,910.));
#274831=CARTESIAN_POINT('',(32.6556469622066,24.2507829119554,1282.35584962783));
#274832=CARTESIAN_POINT('',(32.6556469622065,24.2507829119554,910.));
#274833=CARTESIAN_POINT('Origin',(26.9913553995293,27.008644600471,1282.35584962783));
#274834=CARTESIAN_POINT('Origin',(35.1137781196672,21.3108910330214,910.));
#274835=CARTESIAN_POINT('',(35.1137781196672,21.3108910330214,1282.35584962783));
#274836=CARTESIAN_POINT('',(35.1137781196672,21.3108910330214,910.));
#274837=CARTESIAN_POINT('',(35.1137781196672,21.3108910330214,1282.35584962783));
#274838=CARTESIAN_POINT('Origin',(26.9913553995292,27.0086446004711,910.));
#274839=CARTESIAN_POINT('',(32.6891089669786,18.8862218803328,1282.35584962783));
#274840=CARTESIAN_POINT('',(32.6891089669786,18.8862218803329,910.));
#274841=CARTESIAN_POINT('Origin',(26.9913553995293,27.008644600471,1282.35584962783));
#274842=CARTESIAN_POINT('Origin',(32.6891089669786,18.8862218803329,910.));
#274843=CARTESIAN_POINT('',(29.7492170880445,21.3443530377939,1282.35584962783));
#274844=CARTESIAN_POINT('',(29.7492170880447,21.3443530377937,910.));
#274845=CARTESIAN_POINT('',(32.6891089669786,18.8862218803329,1282.35584962783));
#274846=CARTESIAN_POINT('Origin',(26.9913553995292,27.0086446004711,910.));
#274847=CARTESIAN_POINT('',(24.2334937110135,21.3443530377937,1282.35584962783));
#274848=CARTESIAN_POINT('',(24.2334937110137,21.3443530377937,910.));
#274849=CARTESIAN_POINT('Origin',(26.9913553995293,27.008644600471,1282.35584962783));
#274850=CARTESIAN_POINT('Origin',(21.2936018320797,18.8862218803329,910.));
#274851=CARTESIAN_POINT('',(21.2936018320795,18.8862218803326,1282.35584962783));
#274852=CARTESIAN_POINT('',(21.2936018320797,18.8862218803329,910.));
#274853=CARTESIAN_POINT('',(21.2936018320798,18.8862218803328,1282.35584962783));
#274854=CARTESIAN_POINT('Origin',(26.9913553995292,27.0086446004711,910.));
#274855=CARTESIAN_POINT('',(18.8689326793911,21.3108910330216,1282.35584962783));
#274856=CARTESIAN_POINT('',(18.8689326793911,21.3108910330215,910.));
#274857=CARTESIAN_POINT('Origin',(26.9913553995293,27.008644600471,1282.35584962783));
#274858=CARTESIAN_POINT('Origin',(18.8689326793911,21.3108910330215,910.));
#274859=CARTESIAN_POINT('',(21.3270638368522,24.2507829119557,1282.35584962783));
#274860=CARTESIAN_POINT('',(21.3270638368519,24.2507829119555,910.));
#274861=CARTESIAN_POINT('',(18.8689326793912,21.3108910330214,1282.35584962783));
#274862=CARTESIAN_POINT('Origin',(26.9913553995292,27.0086446004711,910.));
#274863=CARTESIAN_POINT('',(21.3270638368519,29.7665062889867,1282.35584962783));
#274864=CARTESIAN_POINT('',(21.3270638368518,29.7665062889867,910.));
#274865=CARTESIAN_POINT('Origin',(26.9913553995293,27.008644600471,1282.35584962783));
#274866=CARTESIAN_POINT('Origin',(18.8689326793911,32.7063981679206,910.));
#274867=CARTESIAN_POINT('',(18.8689326793909,32.7063981679208,1282.35584962783));
#274868=CARTESIAN_POINT('',(18.8689326793911,32.7063981679206,910.));
#274869=CARTESIAN_POINT('',(18.8689326793911,32.7063981679206,1282.35584962783));
#274870=CARTESIAN_POINT('Origin',(26.9913553995292,27.0086446004711,910.));
#274871=CARTESIAN_POINT('',(21.2936018320797,35.1310673206091,1282.35584962783));
#274872=CARTESIAN_POINT('',(21.2936018320797,35.1310673206092,910.));
#274873=CARTESIAN_POINT('Origin',(26.9913553995293,27.008644600471,1282.35584962783));
#274874=CARTESIAN_POINT('Origin',(21.2936018320797,35.1310673206092,910.));
#274875=CARTESIAN_POINT('',(21.2936018320797,35.1310673206092,1282.35584962783));
#274876=CARTESIAN_POINT('Origin',(32.6891089669788,35.1310673206092,910.));
#274877=CARTESIAN_POINT('',(32.6891089669788,35.131067320609,1282.35584962783));
#274878=CARTESIAN_POINT('',(32.6891089669788,35.1310673206092,910.));
#274879=CARTESIAN_POINT('',(32.6891089669788,35.1310673206091,1282.35584962783));
#274880=CARTESIAN_POINT('Origin',(26.9913553995292,27.0086446004711,910.));
#274881=CARTESIAN_POINT('Origin',(26.9913553995293,27.008644600471,1282.35584962783));
#274882=CARTESIAN_POINT('Origin',(0.,0.,1282.35584962783));
#274883=CARTESIAN_POINT('Origin',(0.,0.,-260.));
#274884=CARTESIAN_POINT('',(45.8841553995292,51.6776446004711,-260.));
#274885=CARTESIAN_POINT('',(44.0841553995292,49.8776446004711,-260.));
#274886=CARTESIAN_POINT('Origin',(45.8841553995292,49.8776446004711,-260.));
#274887=CARTESIAN_POINT('',(44.0841553995292,45.9014446004712,-260.));
#274888=CARTESIAN_POINT('',(44.0841553995292,49.8776446004711,-260.));
#274889=CARTESIAN_POINT('',(45.8841553995292,44.1014446004712,-260.));
#274890=CARTESIAN_POINT('Origin',(45.8841553995292,45.9014446004712,-260.));
#274891=CARTESIAN_POINT('',(49.860355399529,44.1014446004712,-260.));
#274892=CARTESIAN_POINT('',(45.8841553995292,44.1014446004712,-260.));
#274893=CARTESIAN_POINT('',(51.6603553995291,45.9014446004712,-260.));
#274894=CARTESIAN_POINT('Origin',(49.860355399529,45.9014446004712,-260.));
#274895=CARTESIAN_POINT('',(51.6603553995291,49.8776446004711,-260.));
#274896=CARTESIAN_POINT('',(51.6603553995291,45.9014446004712,-260.));
#274897=CARTESIAN_POINT('',(49.8603553995291,51.6776446004711,-260.));
#274898=CARTESIAN_POINT('Origin',(49.8603553995291,49.8776446004711,-260.));
#274899=CARTESIAN_POINT('',(49.8603553995291,51.6776446004711,-260.));
#274900=CARTESIAN_POINT('Origin',(49.8603553995293,51.6776446004708,910.));
#274901=CARTESIAN_POINT('',(49.8603553995293,51.6776446004708,1282.35584962783));
#274902=CARTESIAN_POINT('',(49.8603553995293,51.6776446004708,910.));
#274903=CARTESIAN_POINT('',(45.8841553995295,51.6776446004708,1282.35584962783));
#274904=CARTESIAN_POINT('',(49.8603553995293,51.6776446004708,1282.35584962783));
#274905=CARTESIAN_POINT('',(45.8841553995294,51.6776446004709,910.));
#274906=CARTESIAN_POINT('Origin',(49.8603553995293,49.8776446004709,910.));
#274907=CARTESIAN_POINT('',(51.6603553995293,49.8776446004708,1282.35584962783));
#274908=CARTESIAN_POINT('',(51.6603553995293,49.8776446004709,910.));
#274909=CARTESIAN_POINT('Origin',(49.8603553995293,49.8776446004708,1282.35584962783));
#274910=CARTESIAN_POINT('Origin',(51.6603553995293,45.901444600471,910.));
#274911=CARTESIAN_POINT('',(51.6603553995293,45.901444600471,1282.35584962783));
#274912=CARTESIAN_POINT('',(51.6603553995293,45.901444600471,910.));
#274913=CARTESIAN_POINT('',(51.6603553995293,45.901444600471,1282.35584962783));
#274914=CARTESIAN_POINT('Origin',(49.8603553995293,45.901444600471,910.));
#274915=CARTESIAN_POINT('',(49.8603553995292,44.1014446004709,1282.35584962783));
#274916=CARTESIAN_POINT('',(49.8603553995293,44.101444600471,910.));
#274917=CARTESIAN_POINT('Origin',(49.8603553995293,45.9014446004709,1282.35584962783));
#274918=CARTESIAN_POINT('Origin',(45.8841553995294,44.101444600471,910.));
#274919=CARTESIAN_POINT('',(45.8841553995292,44.101444600471,1282.35584962783));
#274920=CARTESIAN_POINT('',(45.8841553995294,44.101444600471,910.));
#274921=CARTESIAN_POINT('',(45.8841553995294,44.101444600471,1282.35584962783));
#274922=CARTESIAN_POINT('Origin',(45.8841553995294,45.901444600471,910.));
#274923=CARTESIAN_POINT('',(44.0841553995295,45.9014446004711,1282.35584962783));
#274924=CARTESIAN_POINT('',(44.0841553995294,45.901444600471,910.));
#274925=CARTESIAN_POINT('Origin',(45.8841553995295,45.901444600471,1282.35584962783));
#274926=CARTESIAN_POINT('Origin',(44.0841553995294,49.8776446004709,910.));
#274927=CARTESIAN_POINT('',(44.0841553995295,49.8776446004711,1282.35584962783));
#274928=CARTESIAN_POINT('',(44.0841553995294,49.8776446004709,910.));
#274929=CARTESIAN_POINT('',(44.0841553995295,49.8776446004709,1282.35584962783));
#274930=CARTESIAN_POINT('Origin',(45.8841553995294,49.8776446004709,910.));
#274931=CARTESIAN_POINT('Origin',(45.8841553995295,49.8776446004708,1282.35584962783));
#274932=CARTESIAN_POINT('Origin',(0.,0.,1282.35584962783));
#274933=CARTESIAN_POINT('Origin',(-27.0086446004713,27.0086446004712,910.));
#274934=CARTESIAN_POINT('',(-32.6729361631486,29.7665062889868,1282.35584962783));
#274935=CARTESIAN_POINT('',(-32.6729361631486,24.2507829119556,1282.35584962783));
#274936=CARTESIAN_POINT('Origin',(-27.0086446004713,27.0086446004712,1282.35584962783));
#274937=CARTESIAN_POINT('',(-32.6729361631487,24.2507829119556,-260.));
#274938=CARTESIAN_POINT('',(-32.6729361631487,24.2507829119556,910.));
#274939=CARTESIAN_POINT('',(-32.6729361631487,29.7665062889868,-260.));
#274940=CARTESIAN_POINT('Origin',(-27.0086446004713,27.0086446004712,-260.));
#274941=CARTESIAN_POINT('',(-32.6729361631487,29.7665062889868,910.));
#274942=CARTESIAN_POINT('Origin',(0.,0.,-260.));
#274943=CARTESIAN_POINT('',(-32.7063981679208,35.1310673206093,-260.));
#274944=CARTESIAN_POINT('',(-35.1310673206094,32.7063981679208,-260.));
#274945=CARTESIAN_POINT('Origin',(-27.0086446004713,27.0086446004712,-260.));
#274946=CARTESIAN_POINT('',(-35.1310673206094,32.7063981679208,-260.));
#274947=CARTESIAN_POINT('',(-35.1310673206094,21.3108910330216,-260.));
#274948=CARTESIAN_POINT('',(-35.1310673206094,21.3108910330216,-260.));
#274949=CARTESIAN_POINT('',(-32.7063981679208,18.886221880333,-260.));
#274950=CARTESIAN_POINT('Origin',(-27.0086446004713,27.0086446004712,-260.));
#274951=CARTESIAN_POINT('',(-29.7665062889869,21.3443530377938,-260.));
#274952=CARTESIAN_POINT('',(-32.7063981679208,18.886221880333,-260.));
#274953=CARTESIAN_POINT('',(-24.2507829119557,21.3443530377939,-260.));
#274954=CARTESIAN_POINT('Origin',(-27.0086446004713,27.0086446004712,-260.));
#274955=CARTESIAN_POINT('',(-21.3108910330217,18.8862218803331,-260.));
#274956=CARTESIAN_POINT('',(-21.3108910330217,18.8862218803331,-260.));
#274957=CARTESIAN_POINT('',(-18.8862218803331,21.3108910330218,-260.));
#274958=CARTESIAN_POINT('Origin',(-27.0086446004713,27.0086446004712,-260.));
#274959=CARTESIAN_POINT('',(-21.3443530377939,24.2507829119557,-260.));
#274960=CARTESIAN_POINT('',(-18.8862218803331,21.3108910330218,-260.));
#274961=CARTESIAN_POINT('',(-21.3443530377939,29.7665062889867,-260.));
#274962=CARTESIAN_POINT('Origin',(-27.0086446004713,27.0086446004712,-260.));
#274963=CARTESIAN_POINT('',(-18.8862218803331,32.7063981679206,-260.));
#274964=CARTESIAN_POINT('',(-18.8862218803331,32.7063981679206,-260.));
#274965=CARTESIAN_POINT('',(-21.3108910330217,35.1310673206092,-260.));
#274966=CARTESIAN_POINT('Origin',(-27.0086446004713,27.0086446004712,-260.));
#274967=CARTESIAN_POINT('',(-24.2507829119557,32.6729361631485,-260.));
#274968=CARTESIAN_POINT('',(-21.3108910330217,35.1310673206092,-260.));
#274969=CARTESIAN_POINT('',(-29.7665062889869,32.6729361631486,-260.));
#274970=CARTESIAN_POINT('Origin',(-27.0086446004713,27.0086446004712,-260.));
#274971=CARTESIAN_POINT('',(-32.7063981679208,35.1310673206093,-260.));
#274972=CARTESIAN_POINT('Origin',(-32.7063981679208,35.1310673206093,910.));
#274973=CARTESIAN_POINT('',(-29.7665062889869,32.6729361631486,1282.35584962783));
#274974=CARTESIAN_POINT('',(-29.7665062889869,32.6729361631486,910.));
#274975=CARTESIAN_POINT('',(-32.7063981679208,35.1310673206093,1282.35584962783));
#274976=CARTESIAN_POINT('',(-32.7063981679208,35.1310673206093,1282.35584962783));
#274977=CARTESIAN_POINT('',(-32.7063981679208,35.1310673206093,910.));
#274978=CARTESIAN_POINT('Origin',(-27.0086446004713,27.0086446004712,910.));
#274979=CARTESIAN_POINT('',(-24.2507829119557,32.6729361631485,1282.35584962783));
#274980=CARTESIAN_POINT('',(-24.2507829119557,32.6729361631485,910.));
#274981=CARTESIAN_POINT('Origin',(-27.0086446004713,27.0086446004712,1282.35584962783));
#274982=CARTESIAN_POINT('Origin',(-21.3108910330217,35.1310673206092,910.));
#274983=CARTESIAN_POINT('',(-21.3108910330217,35.1310673206092,1282.35584962783));
#274984=CARTESIAN_POINT('',(-21.3108910330217,35.1310673206092,910.));
#274985=CARTESIAN_POINT('',(-21.3108910330217,35.1310673206092,1282.35584962783));
#274986=CARTESIAN_POINT('Origin',(-27.0086446004713,27.0086446004712,910.));
#274987=CARTESIAN_POINT('',(-18.8862218803331,32.7063981679206,1282.35584962783));
#274988=CARTESIAN_POINT('',(-18.8862218803331,32.7063981679206,910.));
#274989=CARTESIAN_POINT('Origin',(-27.0086446004713,27.0086446004712,1282.35584962783));
#274990=CARTESIAN_POINT('Origin',(-18.8862218803331,32.7063981679206,910.));
#274991=CARTESIAN_POINT('',(-21.3443530377939,29.7665062889867,1282.35584962783));
#274992=CARTESIAN_POINT('',(-21.3443530377939,29.7665062889867,910.));
#274993=CARTESIAN_POINT('',(-18.8862218803331,32.7063981679206,1282.35584962783));
#274994=CARTESIAN_POINT('Origin',(-27.0086446004713,27.0086446004712,910.));
#274995=CARTESIAN_POINT('',(-21.3443530377939,24.2507829119557,1282.35584962783));
#274996=CARTESIAN_POINT('',(-21.3443530377939,24.2507829119557,910.));
#274997=CARTESIAN_POINT('Origin',(-27.0086446004713,27.0086446004712,1282.35584962783));
#274998=CARTESIAN_POINT('Origin',(-18.8862218803331,21.3108910330218,910.));
#274999=CARTESIAN_POINT('',(-18.8862218803331,21.3108910330218,1282.35584962783));
#275000=CARTESIAN_POINT('',(-18.8862218803331,21.3108910330218,910.));
#275001=CARTESIAN_POINT('',(-18.8862218803331,21.3108910330218,1282.35584962783));
#275002=CARTESIAN_POINT('Origin',(-27.0086446004713,27.0086446004712,910.));
#275003=CARTESIAN_POINT('',(-21.3108910330217,18.8862218803331,1282.35584962783));
#275004=CARTESIAN_POINT('',(-21.3108910330217,18.8862218803331,910.));
#275005=CARTESIAN_POINT('Origin',(-27.0086446004713,27.0086446004712,1282.35584962783));
#275006=CARTESIAN_POINT('Origin',(-21.3108910330217,18.8862218803331,910.));
#275007=CARTESIAN_POINT('',(-24.2507829119557,21.3443530377939,1282.35584962783));
#275008=CARTESIAN_POINT('',(-24.2507829119557,21.3443530377939,910.));
#275009=CARTESIAN_POINT('',(-21.3108910330217,18.8862218803331,1282.35584962783));
#275010=CARTESIAN_POINT('Origin',(-27.0086446004713,27.0086446004712,910.));
#275011=CARTESIAN_POINT('',(-29.7665062889869,21.3443530377938,1282.35584962783));
#275012=CARTESIAN_POINT('',(-29.7665062889869,21.3443530377938,910.));
#275013=CARTESIAN_POINT('Origin',(-27.0086446004713,27.0086446004712,1282.35584962783));
#275014=CARTESIAN_POINT('Origin',(-32.7063981679208,18.886221880333,910.));
#275015=CARTESIAN_POINT('',(-32.7063981679208,18.886221880333,1282.35584962783));
#275016=CARTESIAN_POINT('',(-32.7063981679208,18.886221880333,910.));
#275017=CARTESIAN_POINT('',(-32.7063981679208,18.886221880333,1282.35584962783));
#275018=CARTESIAN_POINT('Origin',(-27.0086446004713,27.0086446004712,910.));
#275019=CARTESIAN_POINT('',(-35.1310673206094,21.3108910330216,1282.35584962783));
#275020=CARTESIAN_POINT('',(-35.1310673206094,21.3108910330216,910.));
#275021=CARTESIAN_POINT('Origin',(-27.0086446004713,27.0086446004712,1282.35584962783));
#275022=CARTESIAN_POINT('Origin',(-35.1310673206094,21.3108910330216,910.));
#275023=CARTESIAN_POINT('',(-35.1310673206094,21.3108910330216,1282.35584962783));
#275024=CARTESIAN_POINT('Origin',(-35.1310673206094,32.7063981679208,910.));
#275025=CARTESIAN_POINT('',(-35.1310673206094,32.7063981679208,1282.35584962783));
#275026=CARTESIAN_POINT('',(-35.1310673206094,32.7063981679208,910.));
#275027=CARTESIAN_POINT('',(-35.1310673206094,32.7063981679208,1282.35584962783));
#275028=CARTESIAN_POINT('Origin',(-27.0086446004713,27.0086446004712,910.));
#275029=CARTESIAN_POINT('Origin',(-27.0086446004713,27.0086446004712,1282.35584962783));
#275030=CARTESIAN_POINT('Origin',(0.,0.,1282.35584962783));
#275031=CARTESIAN_POINT('Origin',(0.,0.,-260.));
#275032=CARTESIAN_POINT('',(-51.6776446004712,45.9014446004714,-260.));
#275033=CARTESIAN_POINT('',(-49.8776446004712,44.1014446004714,-260.));
#275034=CARTESIAN_POINT('Origin',(-49.8776446004712,45.9014446004714,-260.));
#275035=CARTESIAN_POINT('',(-45.9014446004713,44.1014446004714,-260.));
#275036=CARTESIAN_POINT('',(-49.8776446004712,44.1014446004714,-260.));
#275037=CARTESIAN_POINT('',(-44.1014446004713,45.9014446004714,-260.));
#275038=CARTESIAN_POINT('Origin',(-45.9014446004713,45.9014446004714,-260.));
#275039=CARTESIAN_POINT('',(-44.1014446004713,49.8776446004712,-260.));
#275040=CARTESIAN_POINT('',(-44.1014446004713,45.9014446004714,-260.));
#275041=CARTESIAN_POINT('',(-45.9014446004713,51.6776446004712,-260.));
#275042=CARTESIAN_POINT('Origin',(-45.9014446004713,49.8776446004712,-260.));
#275043=CARTESIAN_POINT('',(-49.8776446004712,51.6776446004712,-260.));
#275044=CARTESIAN_POINT('',(-45.9014446004713,51.6776446004712,-260.));
#275045=CARTESIAN_POINT('',(-51.6776446004712,49.8776446004712,-260.));
#275046=CARTESIAN_POINT('Origin',(-49.8776446004712,49.8776446004712,-260.));
#275047=CARTESIAN_POINT('',(-51.6776446004712,49.8776446004712,-260.));
#275048=CARTESIAN_POINT('Origin',(-51.6776446004712,49.8776446004712,910.));
#275049=CARTESIAN_POINT('',(-51.6776446004712,49.8776446004712,1282.35584962783));
#275050=CARTESIAN_POINT('',(-51.6776446004712,49.8776446004712,910.));
#275051=CARTESIAN_POINT('',(-51.6776446004712,45.9014446004714,1282.35584962783));
#275052=CARTESIAN_POINT('',(-51.6776446004712,49.8776446004712,1282.35584962783));
#275053=CARTESIAN_POINT('',(-51.6776446004712,45.9014446004714,910.));
#275054=CARTESIAN_POINT('Origin',(-49.8776446004712,49.8776446004712,910.));
#275055=CARTESIAN_POINT('',(-49.8776446004712,51.6776446004712,1282.35584962783));
#275056=CARTESIAN_POINT('',(-49.8776446004712,51.6776446004712,910.));
#275057=CARTESIAN_POINT('Origin',(-49.8776446004712,49.8776446004712,1282.35584962783));
#275058=CARTESIAN_POINT('Origin',(-45.9014446004713,51.6776446004712,910.));
#275059=CARTESIAN_POINT('',(-45.9014446004713,51.6776446004712,1282.35584962783));
#275060=CARTESIAN_POINT('',(-45.9014446004713,51.6776446004712,910.));
#275061=CARTESIAN_POINT('',(-45.9014446004713,51.6776446004712,1282.35584962783));
#275062=CARTESIAN_POINT('Origin',(-45.9014446004713,49.8776446004712,910.));
#275063=CARTESIAN_POINT('',(-44.1014446004713,49.8776446004712,1282.35584962783));
#275064=CARTESIAN_POINT('',(-44.1014446004713,49.8776446004712,910.));
#275065=CARTESIAN_POINT('Origin',(-45.9014446004713,49.8776446004712,1282.35584962783));
#275066=CARTESIAN_POINT('Origin',(-44.1014446004713,45.9014446004714,910.));
#275067=CARTESIAN_POINT('',(-44.1014446004713,45.9014446004714,1282.35584962783));
#275068=CARTESIAN_POINT('',(-44.1014446004713,45.9014446004714,910.));
#275069=CARTESIAN_POINT('',(-44.1014446004713,45.9014446004714,1282.35584962783));
#275070=CARTESIAN_POINT('Origin',(-45.9014446004713,45.9014446004714,910.));
#275071=CARTESIAN_POINT('',(-45.9014446004713,44.1014446004714,1282.35584962783));
#275072=CARTESIAN_POINT('',(-45.9014446004713,44.1014446004714,910.));
#275073=CARTESIAN_POINT('Origin',(-45.9014446004713,45.9014446004714,1282.35584962783));
#275074=CARTESIAN_POINT('Origin',(-49.8776446004712,44.1014446004714,910.));
#275075=CARTESIAN_POINT('',(-49.8776446004712,44.1014446004714,1282.35584962783));
#275076=CARTESIAN_POINT('',(-49.8776446004712,44.1014446004714,910.));
#275077=CARTESIAN_POINT('',(-49.8776446004712,44.1014446004714,1282.35584962783));
#275078=CARTESIAN_POINT('Origin',(-49.8776446004712,45.9014446004714,910.));
#275079=CARTESIAN_POINT('Origin',(-49.8776446004712,45.9014446004714,1282.35584962783));
#275080=CARTESIAN_POINT('Origin',(0.,0.,1282.35584962783));
#275081=CARTESIAN_POINT('Origin',(-35.1086446004713,50.0486446004712,910.));
#275082=CARTESIAN_POINT('',(-40.9586446004713,50.0486446004712,1282.35584962783));
#275083=CARTESIAN_POINT('',(-39.1586446004713,50.0486446004712,1282.35584962783));
#275084=CARTESIAN_POINT('',(-35.1086446004713,50.0486446004712,1282.35584962783));
#275085=CARTESIAN_POINT('',(-40.9586446004713,50.0486446004712,-260.));
#275086=CARTESIAN_POINT('',(-40.9586446004713,50.0486446004712,910.));
#275087=CARTESIAN_POINT('',(-39.1586446004713,50.0486446004712,-260.));
#275088=CARTESIAN_POINT('',(-35.1086446004713,50.0486446004712,-260.));
#275089=CARTESIAN_POINT('',(-39.1586446004713,50.0486446004712,910.));
#275090=CARTESIAN_POINT('Origin',(-50.0486446004713,35.1086446004712,910.));
#275091=CARTESIAN_POINT('',(-50.0486446004713,39.1586446004712,1282.35584962783));
#275092=CARTESIAN_POINT('',(-50.0486446004713,40.9586446004712,1282.35584962783));
#275093=CARTESIAN_POINT('',(-50.0486446004713,35.1086446004712,1282.35584962783));
#275094=CARTESIAN_POINT('',(-50.0486446004713,39.1586446004712,-260.));
#275095=CARTESIAN_POINT('',(-50.0486446004713,39.1586446004712,910.));
#275096=CARTESIAN_POINT('',(-50.0486446004713,40.9586446004712,-260.));
#275097=CARTESIAN_POINT('',(-50.0486446004713,35.1086446004712,-260.));
#275098=CARTESIAN_POINT('',(-50.0486446004713,40.9586446004712,910.));
#275099=CARTESIAN_POINT('Origin',(-37.8086446004713,28.5300780298397,910.));
#275100=CARTESIAN_POINT('',(-37.8086446004713,28.5300780298397,1282.35584962783));
#275101=CARTESIAN_POINT('',(-36.9302446004713,27.0086446004712,1282.35584962783));
#275102=CARTESIAN_POINT('',(-37.8086446004713,28.5300780298397,1282.35584962783));
#275103=CARTESIAN_POINT('',(-37.8086446004713,28.5300780298397,-260.));
#275104=CARTESIAN_POINT('',(-37.8086446004713,28.5300780298397,910.));
#275105=CARTESIAN_POINT('',(-36.9302446004713,27.0086446004712,-260.));
#275106=CARTESIAN_POINT('',(-37.8086446004713,28.5300780298397,-260.));
#275107=CARTESIAN_POINT('',(-36.9302446004713,27.0086446004712,910.));
#275108=CARTESIAN_POINT('Origin',(-37.8086446004713,25.4872111711027,910.));
#275109=CARTESIAN_POINT('',(-37.8086446004713,25.4872111711027,1282.35584962783));
#275110=CARTESIAN_POINT('',(-37.8086446004713,25.4872111711027,1282.35584962783));
#275111=CARTESIAN_POINT('',(-37.8086446004713,25.4872111711027,-260.));
#275112=CARTESIAN_POINT('',(-37.8086446004713,25.4872111711027,-260.));
#275113=CARTESIAN_POINT('',(-37.8086446004713,25.4872111711027,910.));
#275114=CARTESIAN_POINT('Origin',(-37.8086446004713,19.7634173219464,910.));
#275115=CARTESIAN_POINT('',(-37.8086446004713,19.7634173219464,1282.35584962783));
#275116=CARTESIAN_POINT('',(-37.8086446004713,19.7634173219464,1282.35584962783));
#275117=CARTESIAN_POINT('',(-37.8086446004713,19.7634173219464,-260.));
#275118=CARTESIAN_POINT('',(-37.8086446004713,19.7634173219464,-260.));
#275119=CARTESIAN_POINT('',(-37.8086446004713,19.7634173219464,910.));
#275120=CARTESIAN_POINT('Origin',(-38.7086446004713,19.7634173219464,910.));
#275121=CARTESIAN_POINT('',(-38.0722484974034,19.1270212188785,1282.35584962783));
#275122=CARTESIAN_POINT('Origin',(-38.7086446004713,19.7634173219464,1282.35584962783));
#275123=CARTESIAN_POINT('',(-38.0722484974034,19.1270212188785,-260.));
#275124=CARTESIAN_POINT('Origin',(-38.7086446004713,19.7634173219464,-260.));
#275125=CARTESIAN_POINT('',(-38.0722484974034,19.1270212188785,910.));
#275126=CARTESIAN_POINT('Origin',(-44.7770212188787,12.4222484974033,910.));
#275127=CARTESIAN_POINT('',(-44.7770212188787,12.4222484974033,1282.35584962783));
#275128=CARTESIAN_POINT('',(-44.7770212188787,12.4222484974033,1282.35584962783));
#275129=CARTESIAN_POINT('',(-44.7770212188787,12.4222484974033,-260.));
#275130=CARTESIAN_POINT('',(-44.7770212188787,12.4222484974033,-260.));
#275131=CARTESIAN_POINT('',(-44.7770212188787,12.4222484974033,910.));
#275132=CARTESIAN_POINT('Origin',(-45.4134173219466,13.0586446004712,910.));
#275133=CARTESIAN_POINT('',(-45.4134173219466,12.1586446004712,1282.35584962783));
#275134=CARTESIAN_POINT('Origin',(-45.4134173219466,13.0586446004712,1282.35584962783));
#275135=CARTESIAN_POINT('',(-45.4134173219466,12.1586446004712,-260.));
#275136=CARTESIAN_POINT('Origin',(-45.4134173219466,13.0586446004712,-260.));
#275137=CARTESIAN_POINT('',(-45.4134173219466,12.1586446004712,910.));
#275138=CARTESIAN_POINT('Origin',(-49.1486446004713,12.1586446004712,910.));
#275139=CARTESIAN_POINT('',(-49.1486446004713,12.1586446004712,1282.35584962783));
#275140=CARTESIAN_POINT('',(-49.1486446004713,12.1586446004712,1282.35584962783));
#275141=CARTESIAN_POINT('',(-49.1486446004713,12.1586446004712,-260.));
#275142=CARTESIAN_POINT('',(-49.1486446004713,12.1586446004712,-260.));
#275143=CARTESIAN_POINT('',(-49.1486446004713,12.1586446004712,910.));
#275144=CARTESIAN_POINT('Origin',(-49.1486446004713,13.0586446004712,910.));
#275145=CARTESIAN_POINT('',(-50.0486446004713,13.0586446004712,1282.35584962783));
#275146=CARTESIAN_POINT('Origin',(-49.1486446004713,13.0586446004712,1282.35584962783));
#275147=CARTESIAN_POINT('',(-50.0486446004713,13.0586446004712,-260.));
#275148=CARTESIAN_POINT('Origin',(-49.1486446004713,13.0586446004712,-260.));
#275149=CARTESIAN_POINT('',(-50.0486446004713,13.0586446004712,910.));
#275150=CARTESIAN_POINT('Origin',(-50.0486446004713,18.9086446004712,910.));
#275151=CARTESIAN_POINT('',(-50.0486446004713,18.9086446004712,1282.35584962783));
#275152=CARTESIAN_POINT('',(-50.0486446004713,18.9086446004712,1282.35584962783));
#275153=CARTESIAN_POINT('',(-50.0486446004713,18.9086446004712,-260.));
#275154=CARTESIAN_POINT('',(-50.0486446004713,18.9086446004712,-260.));
#275155=CARTESIAN_POINT('',(-50.0486446004713,18.9086446004712,910.));
#275156=CARTESIAN_POINT('Origin',(-50.9486446004713,18.9086446004712,910.));
#275157=CARTESIAN_POINT('',(-50.9486446004713,19.8086446004712,1282.35584962783));
#275158=CARTESIAN_POINT('Origin',(-50.9486446004713,18.9086446004712,1282.35584962783));
#275159=CARTESIAN_POINT('',(-50.9486446004713,19.8086446004712,-260.));
#275160=CARTESIAN_POINT('Origin',(-50.9486446004713,18.9086446004712,-260.));
#275161=CARTESIAN_POINT('',(-50.9486446004713,19.8086446004712,910.));
#275162=CARTESIAN_POINT('Origin',(-53.0186446004713,19.8086446004712,910.));
#275163=CARTESIAN_POINT('',(-53.0186446004713,19.8086446004712,1282.35584962783));
#275164=CARTESIAN_POINT('',(-53.0186446004713,19.8086446004712,1282.35584962783));
#275165=CARTESIAN_POINT('',(-53.0186446004713,19.8086446004712,-260.));
#275166=CARTESIAN_POINT('',(-53.0186446004713,19.8086446004712,-260.));
#275167=CARTESIAN_POINT('',(-53.0186446004713,19.8086446004712,910.));
#275168=CARTESIAN_POINT('Origin',(-53.0186446004713,18.8186446004712,910.));
#275169=CARTESIAN_POINT('',(-53.0186446004713,18.8186446004712,1282.35584962783));
#275170=CARTESIAN_POINT('',(-53.0186446004713,18.8186446004712,1282.35584962783));
#275171=CARTESIAN_POINT('',(-53.0186446004713,18.8186446004712,-260.));
#275172=CARTESIAN_POINT('',(-53.0186446004713,18.8186446004712,-260.));
#275173=CARTESIAN_POINT('',(-53.0186446004713,18.8186446004712,910.));
#275174=CARTESIAN_POINT('Origin',(-54.0086446004713,18.8186446004712,910.));
#275175=CARTESIAN_POINT('',(-54.0086446004713,18.8186446004712,1282.35584962783));
#275176=CARTESIAN_POINT('',(-54.0086446004713,18.8186446004712,1282.35584962783));
#275177=CARTESIAN_POINT('',(-54.0086446004713,18.8186446004712,-260.));
#275178=CARTESIAN_POINT('',(-54.0086446004713,18.8186446004712,-260.));
#275179=CARTESIAN_POINT('',(-54.0086446004713,18.8186446004712,910.));
#275180=CARTESIAN_POINT('Origin',(-54.0086446004713,18.8186446004712,910.));
#275181=CARTESIAN_POINT('',(-54.0086446004715,-18.8013553995285,1282.35584962783));
#275182=CARTESIAN_POINT('',(-54.0086446004713,18.8186446004712,1282.35584962783));
#275183=CARTESIAN_POINT('',(-54.0086446004715,-18.8013553995282,-260.));
#275184=CARTESIAN_POINT('',(-54.0086446004713,18.8186446004712,-260.));
#275185=CARTESIAN_POINT('',(-54.0086446004715,-18.8013553995285,910.));
#275186=CARTESIAN_POINT('Origin',(-18.8186446004711,54.0086446004711,910.));
#275187=CARTESIAN_POINT('',(18.8013553995294,54.0086446004711,1282.35584962783));
#275188=CARTESIAN_POINT('',(-18.8186446004711,54.0086446004711,1282.35584962783));
#275189=CARTESIAN_POINT('',(-18.8186446004711,54.0086446004711,1282.35584962783));
#275190=CARTESIAN_POINT('',(18.8013553995293,54.0086446004709,-260.));
#275191=CARTESIAN_POINT('',(18.8013553995293,54.0086446004711,910.));
#275192=CARTESIAN_POINT('',(-18.8186446004711,54.0086446004711,-260.));
#275193=CARTESIAN_POINT('',(-18.8186446004711,54.0086446004711,-260.));
#275194=CARTESIAN_POINT('',(-18.8186446004711,54.0086446004711,910.));
#275195=CARTESIAN_POINT('Origin',(-18.8186446004711,54.0086446004711,910.));
#275196=CARTESIAN_POINT('',(-18.8186446004711,53.0186446004711,1282.35584962783));
#275197=CARTESIAN_POINT('',(-18.8186446004711,54.0086446004711,1282.35584962783));
#275198=CARTESIAN_POINT('',(-18.8186446004711,53.0186446004711,-260.));
#275199=CARTESIAN_POINT('',(-18.8186446004711,54.0086446004711,-260.));
#275200=CARTESIAN_POINT('',(-18.8186446004711,53.0186446004711,910.));
#275201=CARTESIAN_POINT('Origin',(-18.8186446004711,53.0186446004711,910.));
#275202=CARTESIAN_POINT('',(-19.8086446004711,53.0186446004711,1282.35584962783));
#275203=CARTESIAN_POINT('',(-18.8186446004711,53.0186446004711,1282.35584962783));
#275204=CARTESIAN_POINT('',(-19.8086446004711,53.0186446004711,-260.));
#275205=CARTESIAN_POINT('',(-18.8186446004711,53.0186446004711,-260.));
#275206=CARTESIAN_POINT('',(-19.8086446004711,53.0186446004711,910.));
#275207=CARTESIAN_POINT('Origin',(-19.8086446004711,53.0186446004711,910.));
#275208=CARTESIAN_POINT('',(-19.8086446004711,50.9486446004711,1282.35584962783));
#275209=CARTESIAN_POINT('',(-19.8086446004711,53.0186446004711,1282.35584962783));
#275210=CARTESIAN_POINT('',(-19.8086446004711,50.9486446004711,-260.));
#275211=CARTESIAN_POINT('',(-19.8086446004711,53.0186446004711,-260.));
#275212=CARTESIAN_POINT('',(-19.8086446004711,50.9486446004711,910.));
#275213=CARTESIAN_POINT('Origin',(-18.9086446004711,50.9486446004711,910.));
#275214=CARTESIAN_POINT('',(-18.9086446004711,50.0486446004711,1282.35584962783));
#275215=CARTESIAN_POINT('Origin',(-18.9086446004711,50.9486446004711,1282.35584962783));
#275216=CARTESIAN_POINT('',(-18.9086446004711,50.0486446004711,-260.));
#275217=CARTESIAN_POINT('Origin',(-18.9086446004711,50.9486446004711,-260.));
#275218=CARTESIAN_POINT('',(-18.9086446004711,50.0486446004711,910.));
#275219=CARTESIAN_POINT('Origin',(-18.9086446004711,50.0486446004711,910.));
#275220=CARTESIAN_POINT('',(-13.0586446004711,50.0486446004711,1282.35584962783));
#275221=CARTESIAN_POINT('',(-18.9086446004711,50.0486446004711,1282.35584962783));
#275222=CARTESIAN_POINT('',(-13.0586446004711,50.0486446004711,-260.));
#275223=CARTESIAN_POINT('',(-18.9086446004711,50.0486446004711,-260.));
#275224=CARTESIAN_POINT('',(-13.0586446004711,50.0486446004711,910.));
#275225=CARTESIAN_POINT('Origin',(-13.0586446004712,49.1486446004711,910.));
#275226=CARTESIAN_POINT('',(-12.1586446004712,49.1486446004711,1282.35584962783));
#275227=CARTESIAN_POINT('Origin',(-13.0586446004712,49.1486446004711,1282.35584962783));
#275228=CARTESIAN_POINT('',(-12.1586446004712,49.1486446004711,-260.));
#275229=CARTESIAN_POINT('Origin',(-13.0586446004712,49.1486446004711,-260.));
#275230=CARTESIAN_POINT('',(-12.1586446004712,49.1486446004711,910.));
#275231=CARTESIAN_POINT('Origin',(-12.1586446004712,49.1486446004711,910.));
#275232=CARTESIAN_POINT('',(-12.1586446004712,45.4134173219463,1282.35584962783));
#275233=CARTESIAN_POINT('',(-12.1586446004712,49.1486446004711,1282.35584962783));
#275234=CARTESIAN_POINT('',(-12.1586446004712,45.4134173219463,-260.));
#275235=CARTESIAN_POINT('',(-12.1586446004712,49.1486446004711,-260.));
#275236=CARTESIAN_POINT('',(-12.1586446004712,45.4134173219463,910.));
#275237=CARTESIAN_POINT('Origin',(-13.0586446004712,45.4134173219463,910.));
#275238=CARTESIAN_POINT('',(-12.4222484974033,44.7770212188784,1282.35584962783));
#275239=CARTESIAN_POINT('Origin',(-13.0586446004712,45.4134173219463,1282.35584962783));
#275240=CARTESIAN_POINT('',(-12.4222484974033,44.7770212188784,-260.));
#275241=CARTESIAN_POINT('Origin',(-13.0586446004712,45.4134173219463,-260.));
#275242=CARTESIAN_POINT('',(-12.4222484974033,44.7770212188784,910.));
#275243=CARTESIAN_POINT('Origin',(-12.4222484974033,44.7770212188784,910.));
#275244=CARTESIAN_POINT('',(-19.1270212188786,38.0722484974032,1282.35584962783));
#275245=CARTESIAN_POINT('',(-12.4222484974033,44.7770212188784,1282.35584962783));
#275246=CARTESIAN_POINT('',(-19.1270212188786,38.0722484974032,-260.));
#275247=CARTESIAN_POINT('',(-12.4222484974033,44.7770212188784,-260.));
#275248=CARTESIAN_POINT('',(-19.1270212188786,38.0722484974032,910.));
#275249=CARTESIAN_POINT('Origin',(-19.7634173219465,38.7086446004711,910.));
#275250=CARTESIAN_POINT('',(-19.7634173219465,37.8086446004711,1282.35584962783));
#275251=CARTESIAN_POINT('Origin',(-19.7634173219465,38.7086446004711,1282.35584962783));
#275252=CARTESIAN_POINT('',(-19.7634173219465,37.8086446004711,-260.));
#275253=CARTESIAN_POINT('Origin',(-19.7634173219465,38.7086446004711,-260.));
#275254=CARTESIAN_POINT('',(-19.7634173219465,37.8086446004711,910.));
#275255=CARTESIAN_POINT('Origin',(-19.7634173219465,37.8086446004711,910.));
#275256=CARTESIAN_POINT('',(-25.4872111711027,37.8086446004712,1282.35584962783));
#275257=CARTESIAN_POINT('',(-19.7634173219465,37.8086446004711,1282.35584962783));
#275258=CARTESIAN_POINT('',(-25.4872111711027,37.8086446004712,-260.));
#275259=CARTESIAN_POINT('',(-19.7634173219465,37.8086446004711,-260.));
#275260=CARTESIAN_POINT('',(-25.4872111711027,37.8086446004712,910.));
#275261=CARTESIAN_POINT('Origin',(-25.4872111711027,37.8086446004712,910.));
#275262=CARTESIAN_POINT('',(-27.0086446004713,36.9302446004712,1282.35584962783));
#275263=CARTESIAN_POINT('',(-25.4872111711027,37.8086446004712,1282.35584962783));
#275264=CARTESIAN_POINT('',(-27.0086446004713,36.9302446004712,-260.));
#275265=CARTESIAN_POINT('',(-25.4872111711027,37.8086446004712,-260.));
#275266=CARTESIAN_POINT('',(-27.0086446004713,36.9302446004712,910.));
#275267=CARTESIAN_POINT('Origin',(-28.5300780298398,37.8086446004712,910.));
#275268=CARTESIAN_POINT('',(-28.5300780298398,37.8086446004712,1282.35584962783));
#275269=CARTESIAN_POINT('',(-28.5300780298398,37.8086446004712,1282.35584962783));
#275270=CARTESIAN_POINT('',(-28.5300780298398,37.8086446004712,-260.));
#275271=CARTESIAN_POINT('',(-28.5300780298398,37.8086446004712,-260.));
#275272=CARTESIAN_POINT('',(-28.5300780298398,37.8086446004712,910.));
#275273=CARTESIAN_POINT('Origin',(-34.2538718789961,37.8086446004712,910.));
#275274=CARTESIAN_POINT('',(-34.2538718789961,37.8086446004712,1282.35584962783));
#275275=CARTESIAN_POINT('',(-34.2538718789961,37.8086446004712,1282.35584962783));
#275276=CARTESIAN_POINT('',(-34.2538718789961,37.8086446004712,-260.));
#275277=CARTESIAN_POINT('',(-34.2538718789961,37.8086446004712,-260.));
#275278=CARTESIAN_POINT('',(-34.2538718789961,37.8086446004712,910.));
#275279=CARTESIAN_POINT('Origin',(-34.2538718789961,38.7086446004712,910.));
#275280=CARTESIAN_POINT('',(-34.890267982064,38.0722484974033,1282.35584962783));
#275281=CARTESIAN_POINT('Origin',(-34.2538718789961,38.7086446004712,1282.35584962783));
#275282=CARTESIAN_POINT('',(-34.890267982064,38.0722484974033,-260.));
#275283=CARTESIAN_POINT('Origin',(-34.2538718789961,38.7086446004712,-260.));
#275284=CARTESIAN_POINT('',(-34.890267982064,38.0722484974033,910.));
#275285=CARTESIAN_POINT('Origin',(-41.5950407035392,44.7770212188785,910.));
#275286=CARTESIAN_POINT('',(-41.5950407035392,44.7770212188785,1282.35584962783));
#275287=CARTESIAN_POINT('',(-41.5950407035392,44.7770212188785,1282.35584962783));
#275288=CARTESIAN_POINT('',(-41.5950407035392,44.7770212188785,-260.));
#275289=CARTESIAN_POINT('',(-41.5950407035392,44.7770212188785,-260.));
#275290=CARTESIAN_POINT('',(-41.5950407035392,44.7770212188785,910.));
#275291=CARTESIAN_POINT('Origin',(-40.9586446004713,45.4134173219464,910.));
#275292=CARTESIAN_POINT('',(-41.8586446004713,45.4134173219464,1282.35584962783));
#275293=CARTESIAN_POINT('Origin',(-40.9586446004713,45.4134173219464,1282.35584962783));
#275294=CARTESIAN_POINT('',(-41.8586446004713,45.4134173219464,-260.));
#275295=CARTESIAN_POINT('Origin',(-40.9586446004713,45.4134173219464,-260.));
#275296=CARTESIAN_POINT('',(-41.8586446004713,45.4134173219464,910.));
#275297=CARTESIAN_POINT('Origin',(-41.8586446004713,49.1486446004712,910.));
#275298=CARTESIAN_POINT('',(-41.8586446004713,49.1486446004712,1282.35584962783));
#275299=CARTESIAN_POINT('',(-41.8586446004713,49.1486446004712,1282.35584962783));
#275300=CARTESIAN_POINT('',(-41.8586446004713,49.1486446004712,-260.));
#275301=CARTESIAN_POINT('',(-41.8586446004713,49.1486446004712,-260.));
#275302=CARTESIAN_POINT('',(-41.8586446004713,49.1486446004712,910.));
#275303=CARTESIAN_POINT('Origin',(-40.9586446004713,49.1486446004712,910.));
#275304=CARTESIAN_POINT('Origin',(-40.9586446004713,49.1486446004712,1282.35584962783));
#275305=CARTESIAN_POINT('Origin',(-40.9586446004713,49.1486446004712,-260.));
#275306=CARTESIAN_POINT('Origin',(-35.1086446004713,50.0486446004712,910.));
#275307=CARTESIAN_POINT('',(-37.5386446004713,50.0486446004712,1282.35584962783));
#275308=CARTESIAN_POINT('',(-35.1086446004713,50.0486446004712,1282.35584962783));
#275309=CARTESIAN_POINT('',(-35.1086446004713,50.0486446004712,1282.35584962783));
#275310=CARTESIAN_POINT('',(-37.5386446004713,50.0486446004712,-260.));
#275311=CARTESIAN_POINT('',(-37.5386446004713,50.0486446004712,910.));
#275312=CARTESIAN_POINT('',(-35.1086446004713,50.0486446004712,-260.));
#275313=CARTESIAN_POINT('',(-35.1086446004713,50.0486446004712,-260.));
#275314=CARTESIAN_POINT('',(-35.1086446004713,50.0486446004712,910.));
#275315=CARTESIAN_POINT('Origin',(-35.1086446004713,50.9486446004712,910.));
#275316=CARTESIAN_POINT('',(-34.2086446004713,50.9486446004712,1282.35584962783));
#275317=CARTESIAN_POINT('Origin',(-35.1086446004713,50.9486446004712,1282.35584962783));
#275318=CARTESIAN_POINT('',(-34.2086446004713,50.9486446004712,-260.));
#275319=CARTESIAN_POINT('Origin',(-35.1086446004713,50.9486446004712,-260.));
#275320=CARTESIAN_POINT('',(-34.2086446004713,50.9486446004712,910.));
#275321=CARTESIAN_POINT('Origin',(-34.2086446004713,53.0186446004712,910.));
#275322=CARTESIAN_POINT('',(-34.2086446004713,53.0186446004712,1282.35584962783));
#275323=CARTESIAN_POINT('',(-34.2086446004713,53.0186446004712,1282.35584962783));
#275324=CARTESIAN_POINT('',(-34.2086446004713,53.0186446004712,-260.));
#275325=CARTESIAN_POINT('',(-34.2086446004713,53.0186446004712,-260.));
#275326=CARTESIAN_POINT('',(-34.2086446004713,53.0186446004712,910.));
#275327=CARTESIAN_POINT('Origin',(-35.1986446004713,53.0186446004712,910.));
#275328=CARTESIAN_POINT('',(-35.1986446004713,53.0186446004712,1282.35584962783));
#275329=CARTESIAN_POINT('',(-35.1986446004713,53.0186446004712,1282.35584962783));
#275330=CARTESIAN_POINT('',(-35.1986446004713,53.0186446004712,-260.));
#275331=CARTESIAN_POINT('',(-35.1986446004713,53.0186446004712,-260.));
#275332=CARTESIAN_POINT('',(-35.1986446004713,53.0186446004712,910.));
#275333=CARTESIAN_POINT('Origin',(-35.1986446004713,54.0086446004712,910.));
#275334=CARTESIAN_POINT('',(-35.1986446004713,54.0086446004712,1282.35584962783));
#275335=CARTESIAN_POINT('',(-35.1986446004713,54.0086446004712,1282.35584962783));
#275336=CARTESIAN_POINT('',(-35.1986446004713,54.0086446004712,-260.));
#275337=CARTESIAN_POINT('',(-35.1986446004713,54.0086446004712,-260.));
#275338=CARTESIAN_POINT('',(-35.1986446004713,54.0086446004712,910.));
#275339=CARTESIAN_POINT('Origin',(-35.1986446004713,54.0086446004712,910.));
#275340=CARTESIAN_POINT('',(-50.3510446004713,54.0086446004712,1282.35584962783));
#275341=CARTESIAN_POINT('',(-35.1986446004713,54.0086446004712,1282.35584962783));
#275342=CARTESIAN_POINT('',(-50.3510446004713,54.0086446004712,-260.));
#275343=CARTESIAN_POINT('',(-35.1986446004713,54.0086446004712,-260.));
#275344=CARTESIAN_POINT('',(-50.3510446004713,54.0086446004712,910.));
#275345=CARTESIAN_POINT('Origin',(-50.3510446004712,50.3510446004711,910.));
#275346=CARTESIAN_POINT('',(-54.0086446004713,50.3510446004711,1282.35584962783));
#275347=CARTESIAN_POINT('Origin',(-50.3510446004712,50.3510446004711,1282.35584962783));
#275348=CARTESIAN_POINT('',(-54.0086446004713,50.3510446004711,-260.));
#275349=CARTESIAN_POINT('Origin',(-50.3510446004712,50.3510446004711,-260.));
#275350=CARTESIAN_POINT('',(-54.0086446004713,50.3510446004711,910.));
#275351=CARTESIAN_POINT('Origin',(-54.0086446004713,35.1986446004712,910.));
#275352=CARTESIAN_POINT('',(-54.0086446004713,35.1986446004712,1282.35584962783));
#275353=CARTESIAN_POINT('',(-54.0086446004713,35.1986446004712,1282.35584962783));
#275354=CARTESIAN_POINT('',(-54.0086446004713,35.1986446004712,-260.));
#275355=CARTESIAN_POINT('',(-54.0086446004713,35.1986446004712,-260.));
#275356=CARTESIAN_POINT('',(-54.0086446004713,35.1986446004712,910.));
#275357=CARTESIAN_POINT('Origin',(-54.0086446004713,35.1986446004712,910.));
#275358=CARTESIAN_POINT('',(-53.0186446004713,35.1986446004712,1282.35584962783));
#275359=CARTESIAN_POINT('',(-54.0086446004713,35.1986446004712,1282.35584962783));
#275360=CARTESIAN_POINT('',(-53.0186446004713,35.1986446004712,-260.));
#275361=CARTESIAN_POINT('',(-54.0086446004713,35.1986446004712,-260.));
#275362=CARTESIAN_POINT('',(-53.0186446004713,35.1986446004712,910.));
#275363=CARTESIAN_POINT('Origin',(-53.0186446004713,35.1986446004712,910.));
#275364=CARTESIAN_POINT('',(-53.0186446004713,34.2086446004712,1282.35584962783));
#275365=CARTESIAN_POINT('',(-53.0186446004713,35.1986446004712,1282.35584962783));
#275366=CARTESIAN_POINT('',(-53.0186446004713,34.2086446004712,-260.));
#275367=CARTESIAN_POINT('',(-53.0186446004713,35.1986446004712,-260.));
#275368=CARTESIAN_POINT('',(-53.0186446004713,34.2086446004712,910.));
#275369=CARTESIAN_POINT('Origin',(-53.0186446004713,34.2086446004712,910.));
#275370=CARTESIAN_POINT('',(-50.9486446004713,34.2086446004712,1282.35584962783));
#275371=CARTESIAN_POINT('',(-53.0186446004713,34.2086446004712,1282.35584962783));
#275372=CARTESIAN_POINT('',(-50.9486446004713,34.2086446004712,-260.));
#275373=CARTESIAN_POINT('',(-53.0186446004713,34.2086446004712,-260.));
#275374=CARTESIAN_POINT('',(-50.9486446004713,34.2086446004712,910.));
#275375=CARTESIAN_POINT('Origin',(-50.9486446004713,35.1086446004712,910.));
#275376=CARTESIAN_POINT('',(-50.0486446004713,35.1086446004712,1282.35584962783));
#275377=CARTESIAN_POINT('Origin',(-50.9486446004713,35.1086446004712,1282.35584962783));
#275378=CARTESIAN_POINT('',(-50.0486446004713,35.1086446004712,-260.));
#275379=CARTESIAN_POINT('Origin',(-50.9486446004713,35.1086446004712,-260.));
#275380=CARTESIAN_POINT('',(-50.0486446004713,35.1086446004712,910.));
#275381=CARTESIAN_POINT('Origin',(-50.0486446004713,35.1086446004712,910.));
#275382=CARTESIAN_POINT('',(-50.0486446004713,37.5386446004715,1282.35584962783));
#275383=CARTESIAN_POINT('',(-50.0486446004713,35.1086446004712,1282.35584962783));
#275384=CARTESIAN_POINT('',(-50.0486446004712,37.5386446004714,-260.));
#275385=CARTESIAN_POINT('',(-50.0486446004713,35.1086446004712,-260.));
#275386=CARTESIAN_POINT('',(-50.0486446004713,37.5386446004715,910.));
#275387=CARTESIAN_POINT('Origin',(-49.1486446004713,40.9586446004712,910.));
#275388=CARTESIAN_POINT('',(-49.1486446004713,41.8586446004712,1282.35584962783));
#275389=CARTESIAN_POINT('Origin',(-49.1486446004713,40.9586446004712,1282.35584962783));
#275390=CARTESIAN_POINT('',(-49.1486446004713,41.8586446004712,-260.));
#275391=CARTESIAN_POINT('Origin',(-49.1486446004713,40.9586446004712,-260.));
#275392=CARTESIAN_POINT('',(-49.1486446004713,41.8586446004712,910.));
#275393=CARTESIAN_POINT('Origin',(-49.1486446004713,41.8586446004712,910.));
#275394=CARTESIAN_POINT('',(-45.4134173219466,41.8586446004712,1282.35584962783));
#275395=CARTESIAN_POINT('',(-49.1486446004713,41.8586446004712,1282.35584962783));
#275396=CARTESIAN_POINT('',(-45.4134173219466,41.8586446004712,-260.));
#275397=CARTESIAN_POINT('',(-49.1486446004713,41.8586446004712,-260.));
#275398=CARTESIAN_POINT('',(-45.4134173219466,41.8586446004712,910.));
#275399=CARTESIAN_POINT('Origin',(-45.4134173219466,40.9586446004712,910.));
#275400=CARTESIAN_POINT('',(-44.7770212188787,41.5950407035391,1282.35584962783));
#275401=CARTESIAN_POINT('Origin',(-45.4134173219466,40.9586446004712,1282.35584962783));
#275402=CARTESIAN_POINT('',(-44.7770212188787,41.5950407035391,-260.));
#275403=CARTESIAN_POINT('Origin',(-45.4134173219466,40.9586446004712,-260.));
#275404=CARTESIAN_POINT('',(-44.7770212188787,41.5950407035391,910.));
#275405=CARTESIAN_POINT('Origin',(-44.7770212188787,41.5950407035391,910.));
#275406=CARTESIAN_POINT('',(-38.0722484974034,34.8902679820638,1282.35584962783));
#275407=CARTESIAN_POINT('',(-44.7770212188787,41.5950407035391,1282.35584962783));
#275408=CARTESIAN_POINT('',(-38.0722484974034,34.8902679820638,-260.));
#275409=CARTESIAN_POINT('',(-44.7770212188787,41.5950407035391,-260.));
#275410=CARTESIAN_POINT('',(-38.0722484974034,34.8902679820638,910.));
#275411=CARTESIAN_POINT('Origin',(-38.7086446004713,34.2538718789959,910.));
#275412=CARTESIAN_POINT('',(-37.8086446004713,34.2538718789959,1282.35584962783));
#275413=CARTESIAN_POINT('Origin',(-38.7086446004713,34.2538718789959,1282.35584962783));
#275414=CARTESIAN_POINT('',(-37.8086446004713,34.2538718789959,-260.));
#275415=CARTESIAN_POINT('Origin',(-38.7086446004713,34.2538718789959,-260.));
#275416=CARTESIAN_POINT('',(-37.8086446004713,34.2538718789959,910.));
#275417=CARTESIAN_POINT('Origin',(-37.8086446004713,34.2538718789959,910.));
#275418=CARTESIAN_POINT('',(-37.8086446004713,34.2538718789959,1282.35584962783));
#275419=CARTESIAN_POINT('',(-37.8086446004713,34.2538718789959,-260.));
#275420=CARTESIAN_POINT('Origin',(28.5127888288977,37.8086446004711,910.));
#275421=CARTESIAN_POINT('',(28.5127888288978,37.808644600471,1282.35584962783));
#275422=CARTESIAN_POINT('',(26.9913553995293,36.930244600471,1282.35584962783));
#275423=CARTESIAN_POINT('',(28.5127888288978,37.808644600471,1282.35584962783));
#275424=CARTESIAN_POINT('',(28.5127888288977,37.8086446004714,-260.));
#275425=CARTESIAN_POINT('',(28.5127888288977,37.8086446004711,910.));
#275426=CARTESIAN_POINT('',(26.9913553995292,36.9302446004712,-260.));
#275427=CARTESIAN_POINT('',(28.5127888288975,37.8086446004713,-260.));
#275428=CARTESIAN_POINT('',(26.9913553995292,36.9302446004711,910.));
#275429=CARTESIAN_POINT('Origin',(25.4699219701607,37.8086446004711,910.));
#275430=CARTESIAN_POINT('',(25.4699219701608,37.808644600471,1282.35584962783));
#275431=CARTESIAN_POINT('',(25.4699219701607,37.8086446004711,1282.35584962783));
#275432=CARTESIAN_POINT('',(25.4699219701607,37.8086446004713,-260.));
#275433=CARTESIAN_POINT('',(25.4699219701605,37.8086446004713,-260.));
#275434=CARTESIAN_POINT('',(25.4699219701607,37.8086446004711,910.));
#275435=CARTESIAN_POINT('Origin',(19.7461281210045,37.8086446004711,910.));
#275436=CARTESIAN_POINT('',(19.7461281210046,37.808644600471,1282.35584962783));
#275437=CARTESIAN_POINT('',(19.7461281210045,37.808644600471,1282.35584962783));
#275438=CARTESIAN_POINT('',(19.7461281210043,37.8086446004713,-260.));
#275439=CARTESIAN_POINT('',(19.7461281210043,37.8086446004713,-260.));
#275440=CARTESIAN_POINT('',(19.7461281210045,37.8086446004711,910.));
#275441=CARTESIAN_POINT('Origin',(19.7461281210045,38.7086446004711,910.));
#275442=CARTESIAN_POINT('',(19.1097320179367,38.0722484974032,1282.35584962783));
#275443=CARTESIAN_POINT('Origin',(19.7461281210046,38.708644600471,1282.35584962783));
#275444=CARTESIAN_POINT('',(19.1097320179366,38.0722484974032,-260.));
#275445=CARTESIAN_POINT('Origin',(19.7461281210043,38.7086446004713,-260.));
#275446=CARTESIAN_POINT('',(19.1097320179366,38.0722484974032,910.));
#275447=CARTESIAN_POINT('Origin',(12.4049592964614,44.7770212188785,910.));
#275448=CARTESIAN_POINT('',(12.4049592964614,44.7770212188784,1282.35584962783));
#275449=CARTESIAN_POINT('',(12.4049592964614,44.7770212188785,1282.35584962783));
#275450=CARTESIAN_POINT('',(12.4049592964612,44.7770212188787,-260.));
#275451=CARTESIAN_POINT('',(12.4049592964612,44.7770212188787,-260.));
#275452=CARTESIAN_POINT('',(12.4049592964614,44.7770212188785,910.));
#275453=CARTESIAN_POINT('Origin',(13.0413553995293,45.4134173219464,910.));
#275454=CARTESIAN_POINT('',(12.1413553995293,45.4134173219463,1282.35584962783));
#275455=CARTESIAN_POINT('Origin',(13.0413553995293,45.4134173219463,1282.35584962783));
#275456=CARTESIAN_POINT('',(12.1413553995291,45.4134173219464,-260.));
#275457=CARTESIAN_POINT('Origin',(13.041355399529,45.4134173219466,-260.));
#275458=CARTESIAN_POINT('',(12.1413553995293,45.4134173219464,910.));
#275459=CARTESIAN_POINT('Origin',(12.1413553995293,49.1486446004711,910.));
#275460=CARTESIAN_POINT('',(12.1413553995293,49.1486446004711,1282.35584962783));
#275461=CARTESIAN_POINT('',(12.1413553995293,49.1486446004711,1282.35584962783));
#275462=CARTESIAN_POINT('',(12.1413553995291,49.1486446004713,-260.));
#275463=CARTESIAN_POINT('',(12.1413553995291,49.1486446004713,-260.));
#275464=CARTESIAN_POINT('',(12.1413553995293,49.1486446004711,910.));
#275465=CARTESIAN_POINT('Origin',(13.0413553995293,49.1486446004711,910.));
#275466=CARTESIAN_POINT('',(13.0413553995293,50.0486446004711,1282.35584962783));
#275467=CARTESIAN_POINT('Origin',(13.0413553995293,49.1486446004711,1282.35584962783));
#275468=CARTESIAN_POINT('',(13.0413553995291,50.0486446004713,-260.));
#275469=CARTESIAN_POINT('Origin',(13.0413553995291,49.1486446004713,-260.));
#275470=CARTESIAN_POINT('',(13.0413553995293,50.0486446004711,910.));
#275471=CARTESIAN_POINT('Origin',(18.8913553995293,50.0486446004711,910.));
#275472=CARTESIAN_POINT('',(18.8913553995294,50.048644600471,1282.35584962783));
#275473=CARTESIAN_POINT('',(18.8913553995293,50.048644600471,1282.35584962783));
#275474=CARTESIAN_POINT('',(18.8913553995291,50.0486446004713,-260.));
#275475=CARTESIAN_POINT('',(18.8913553995291,50.0486446004713,-260.));
#275476=CARTESIAN_POINT('',(18.8913553995293,50.0486446004711,910.));
#275477=CARTESIAN_POINT('Origin',(18.8913553995293,50.9486446004711,910.));
#275478=CARTESIAN_POINT('',(19.7913553995294,50.948644600471,1282.35584962783));
#275479=CARTESIAN_POINT('Origin',(18.8913553995294,50.948644600471,1282.35584962783));
#275480=CARTESIAN_POINT('',(19.7913553995291,50.9486446004711,-260.));
#275481=CARTESIAN_POINT('Origin',(18.8913553995291,50.9486446004713,-260.));
#275482=CARTESIAN_POINT('',(19.7913553995293,50.9486446004711,910.));
#275483=CARTESIAN_POINT('Origin',(19.7913553995293,53.0186446004711,910.));
#275484=CARTESIAN_POINT('',(19.7913553995294,53.018644600471,1282.35584962783));
#275485=CARTESIAN_POINT('',(19.7913553995294,53.0186446004711,1282.35584962783));
#275486=CARTESIAN_POINT('',(19.7913553995293,53.0186446004713,-260.));
#275487=CARTESIAN_POINT('',(19.7913553995291,53.0186446004713,-260.));
#275488=CARTESIAN_POINT('',(19.7913553995293,53.0186446004711,910.));
#275489=CARTESIAN_POINT('Origin',(18.8013553995293,53.0186446004711,910.));
#275490=CARTESIAN_POINT('',(18.8013553995294,53.018644600471,1282.35584962783));
#275491=CARTESIAN_POINT('',(18.8013553995293,53.018644600471,1282.35584962783));
#275492=CARTESIAN_POINT('',(18.8013553995291,53.0186446004711,-260.));
#275493=CARTESIAN_POINT('',(18.8013553995291,53.0186446004713,-260.));
#275494=CARTESIAN_POINT('',(18.8013553995293,53.0186446004711,910.));
#275495=CARTESIAN_POINT('Origin',(18.8013553995293,54.0086446004711,910.));
#275496=CARTESIAN_POINT('',(18.8013553995294,54.0086446004711,1282.35584962783));
#275497=CARTESIAN_POINT('',(18.8013553995291,54.0086446004713,-260.));
#275498=CARTESIAN_POINT('Origin',(53.9913553995291,18.8186446004708,910.));
#275499=CARTESIAN_POINT('',(53.9913553995291,-18.8013553995294,1282.35584962783));
#275500=CARTESIAN_POINT('',(53.9913553995292,18.8186446004707,1282.35584962783));
#275501=CARTESIAN_POINT('',(53.9913553995292,18.8186446004708,1282.35584962783));
#275502=CARTESIAN_POINT('',(53.9913553995285,-18.8013553995292,-260.));
#275503=CARTESIAN_POINT('',(53.9913553995291,-18.8013553995292,910.));
#275504=CARTESIAN_POINT('',(53.9913553995291,18.818644600471,-260.));
#275505=CARTESIAN_POINT('',(53.9913553995289,18.818644600471,-260.));
#275506=CARTESIAN_POINT('',(53.9913553995291,18.8186446004708,910.));
#275507=CARTESIAN_POINT('Origin',(53.9913553995291,18.8186446004708,910.));
#275508=CARTESIAN_POINT('',(53.0013553995292,18.8186446004707,1282.35584962783));
#275509=CARTESIAN_POINT('',(53.9913553995291,18.8186446004707,1282.35584962783));
#275510=CARTESIAN_POINT('',(53.0013553995289,18.8186446004708,-260.));
#275511=CARTESIAN_POINT('',(53.9913553995289,18.818644600471,-260.));
#275512=CARTESIAN_POINT('',(53.0013553995291,18.8186446004708,910.));
#275513=CARTESIAN_POINT('Origin',(53.0013553995291,18.8186446004708,910.));
#275514=CARTESIAN_POINT('',(53.0013553995292,19.8086446004707,1282.35584962783));
#275515=CARTESIAN_POINT('',(53.0013553995292,18.8186446004708,1282.35584962783));
#275516=CARTESIAN_POINT('',(53.0013553995291,19.808644600471,-260.));
#275517=CARTESIAN_POINT('',(53.0013553995289,18.818644600471,-260.));
#275518=CARTESIAN_POINT('',(53.0013553995291,19.8086446004708,910.));
#275519=CARTESIAN_POINT('Origin',(53.0013553995291,19.8086446004708,910.));
#275520=CARTESIAN_POINT('',(50.9313553995292,19.8086446004708,1282.35584962783));
#275521=CARTESIAN_POINT('',(53.0013553995291,19.8086446004707,1282.35584962783));
#275522=CARTESIAN_POINT('',(50.9313553995289,19.808644600471,-260.));
#275523=CARTESIAN_POINT('',(53.0013553995289,19.808644600471,-260.));
#275524=CARTESIAN_POINT('',(50.9313553995291,19.8086446004708,910.));
#275525=CARTESIAN_POINT('Origin',(50.9313553995291,18.9086446004708,910.));
#275526=CARTESIAN_POINT('',(50.0313553995292,18.9086446004708,1282.35584962783));
#275527=CARTESIAN_POINT('Origin',(50.9313553995292,18.9086446004708,1282.35584962783));
#275528=CARTESIAN_POINT('',(50.0313553995289,18.9086446004711,-260.));
#275529=CARTESIAN_POINT('Origin',(50.9313553995289,18.908644600471,-260.));
#275530=CARTESIAN_POINT('',(50.0313553995291,18.9086446004708,910.));
#275531=CARTESIAN_POINT('Origin',(50.0313553995291,18.9086446004708,910.));
#275532=CARTESIAN_POINT('',(50.0313553995291,13.0586446004708,1282.35584962783));
#275533=CARTESIAN_POINT('',(50.0313553995292,18.9086446004708,1282.35584962783));
#275534=CARTESIAN_POINT('',(50.0313553995288,13.0586446004711,-260.));
#275535=CARTESIAN_POINT('',(50.0313553995289,18.9086446004711,-260.));
#275536=CARTESIAN_POINT('',(50.031355399529,13.0586446004708,910.));
#275537=CARTESIAN_POINT('Origin',(49.131355399529,13.0586446004708,910.));
#275538=CARTESIAN_POINT('',(49.1313553995291,12.1586446004708,1282.35584962783));
#275539=CARTESIAN_POINT('Origin',(49.1313553995291,13.0586446004708,1282.35584962783));
#275540=CARTESIAN_POINT('',(49.131355399529,12.1586446004711,-260.));
#275541=CARTESIAN_POINT('Origin',(49.1313553995288,13.0586446004711,-260.));
#275542=CARTESIAN_POINT('',(49.131355399529,12.1586446004708,910.));
#275543=CARTESIAN_POINT('Origin',(49.131355399529,12.1586446004708,910.));
#275544=CARTESIAN_POINT('',(45.3961281210043,12.1586446004708,1282.35584962783));
#275545=CARTESIAN_POINT('',(49.131355399529,12.1586446004708,1282.35584962783));
#275546=CARTESIAN_POINT('',(45.3961281210041,12.1586446004711,-260.));
#275547=CARTESIAN_POINT('',(49.1313553995288,12.1586446004711,-260.));
#275548=CARTESIAN_POINT('',(45.3961281210043,12.1586446004709,910.));
#275549=CARTESIAN_POINT('Origin',(45.3961281210043,13.0586446004709,910.));
#275550=CARTESIAN_POINT('',(44.7597320179365,12.4222484974029,1282.35584962783));
#275551=CARTESIAN_POINT('Origin',(45.3961281210044,13.0586446004708,1282.35584962783));
#275552=CARTESIAN_POINT('',(44.7597320179364,12.422248497403,-260.));
#275553=CARTESIAN_POINT('Origin',(45.3961281210041,13.0586446004711,-260.));
#275554=CARTESIAN_POINT('',(44.7597320179364,12.422248497403,910.));
#275555=CARTESIAN_POINT('Origin',(44.7597320179364,12.422248497403,910.));
#275556=CARTESIAN_POINT('',(38.0549592964613,19.1270212188783,1282.35584962783));
#275557=CARTESIAN_POINT('',(44.7597320179364,12.422248497403,1282.35584962783));
#275558=CARTESIAN_POINT('',(38.054959296461,19.1270212188785,-260.));
#275559=CARTESIAN_POINT('',(44.7597320179362,12.4222484974032,-260.));
#275560=CARTESIAN_POINT('',(38.0549592964612,19.1270212188783,910.));
#275561=CARTESIAN_POINT('Origin',(38.6913553995291,19.7634173219462,910.));
#275562=CARTESIAN_POINT('',(37.7913553995292,19.7634173219462,1282.35584962783));
#275563=CARTESIAN_POINT('Origin',(38.6913553995292,19.7634173219461,1282.35584962783));
#275564=CARTESIAN_POINT('',(37.7913553995289,19.7634173219462,-260.));
#275565=CARTESIAN_POINT('Origin',(38.6913553995289,19.7634173219464,-260.));
#275566=CARTESIAN_POINT('',(37.7913553995291,19.7634173219462,910.));
#275567=CARTESIAN_POINT('Origin',(37.7913553995291,19.7634173219462,910.));
#275568=CARTESIAN_POINT('',(37.7913553995292,25.4872111711024,1282.35584962783));
#275569=CARTESIAN_POINT('',(37.7913553995292,19.7634173219462,1282.35584962783));
#275570=CARTESIAN_POINT('',(37.7913553995291,25.4872111711025,-260.));
#275571=CARTESIAN_POINT('',(37.7913553995289,19.7634173219464,-260.));
#275572=CARTESIAN_POINT('',(37.7913553995292,25.4872111711025,910.));
#275573=CARTESIAN_POINT('Origin',(37.7913553995292,25.4872111711025,910.));
#275574=CARTESIAN_POINT('',(36.9129553995293,27.008644600471,1282.35584962783));
#275575=CARTESIAN_POINT('',(37.7913553995292,25.4872111711025,1282.35584962783));
#275576=CARTESIAN_POINT('',(36.9129553995288,27.0086446004711,-260.));
#275577=CARTESIAN_POINT('',(37.791355399529,25.4872111711027,-260.));
#275578=CARTESIAN_POINT('',(36.9129553995292,27.0086446004711,910.));
#275579=CARTESIAN_POINT('Origin',(37.7913553995292,28.5300780298395,910.));
#275580=CARTESIAN_POINT('',(37.7913553995293,28.5300780298395,1282.35584962783));
#275581=CARTESIAN_POINT('',(37.7913553995293,28.5300780298395,1282.35584962783));
#275582=CARTESIAN_POINT('',(37.791355399529,28.5300780298395,-260.));
#275583=CARTESIAN_POINT('',(37.791355399529,28.5300780298398,-260.));
#275584=CARTESIAN_POINT('',(37.7913553995292,28.5300780298395,910.));
#275585=CARTESIAN_POINT('Origin',(37.7913553995292,34.2538718789958,910.));
#275586=CARTESIAN_POINT('',(37.7913553995293,34.2538718789957,1282.35584962783));
#275587=CARTESIAN_POINT('',(37.7913553995293,34.2538718789958,1282.35584962783));
#275588=CARTESIAN_POINT('',(37.791355399529,34.253871878996,-260.));
#275589=CARTESIAN_POINT('',(37.791355399529,34.253871878996,-260.));
#275590=CARTESIAN_POINT('',(37.7913553995292,34.2538718789958,910.));
#275591=CARTESIAN_POINT('Origin',(38.6913553995292,34.2538718789958,910.));
#275592=CARTESIAN_POINT('',(38.0549592964614,34.8902679820636,1282.35584962783));
#275593=CARTESIAN_POINT('Origin',(38.6913553995293,34.2538718789957,1282.35584962783));
#275594=CARTESIAN_POINT('',(38.0549592964611,34.8902679820639,-260.));
#275595=CARTESIAN_POINT('Origin',(38.691355399529,34.253871878996,-260.));
#275596=CARTESIAN_POINT('',(38.0549592964613,34.8902679820637,910.));
#275597=CARTESIAN_POINT('Origin',(44.7597320179366,41.5950407035389,910.));
#275598=CARTESIAN_POINT('',(44.7597320179367,41.5950407035389,1282.35584962783));
#275599=CARTESIAN_POINT('',(44.7597320179367,41.5950407035389,1282.35584962783));
#275600=CARTESIAN_POINT('',(44.7597320179364,41.5950407035391,-260.));
#275601=CARTESIAN_POINT('',(44.7597320179364,41.5950407035391,-260.));
#275602=CARTESIAN_POINT('',(44.7597320179366,41.5950407035389,910.));
#275603=CARTESIAN_POINT('Origin',(45.3961281210045,40.958644600471,910.));
#275604=CARTESIAN_POINT('',(45.3961281210046,41.858644600471,1282.35584962783));
#275605=CARTESIAN_POINT('Origin',(45.3961281210046,40.958644600471,1282.35584962783));
#275606=CARTESIAN_POINT('',(45.3961281210043,41.8586446004712,-260.));
#275607=CARTESIAN_POINT('Origin',(45.3961281210043,40.9586446004712,-260.));
#275608=CARTESIAN_POINT('',(45.3961281210045,41.858644600471,910.));
#275609=CARTESIAN_POINT('Origin',(49.1313553995292,41.858644600471,910.));
#275610=CARTESIAN_POINT('',(49.1313553995293,41.858644600471,1282.35584962783));
#275611=CARTESIAN_POINT('',(49.1313553995292,41.858644600471,1282.35584962783));
#275612=CARTESIAN_POINT('',(49.131355399529,41.8586446004712,-260.));
#275613=CARTESIAN_POINT('',(49.131355399529,41.8586446004712,-260.));
#275614=CARTESIAN_POINT('',(49.1313553995292,41.858644600471,910.));
#275615=CARTESIAN_POINT('Origin',(49.1313553995292,40.958644600471,910.));
#275616=CARTESIAN_POINT('',(50.0313553995293,40.9586446004709,1282.35584962783));
#275617=CARTESIAN_POINT('Origin',(49.1313553995293,40.958644600471,1282.35584962783));
#275618=CARTESIAN_POINT('',(50.031355399529,40.9586446004712,-260.));
#275619=CARTESIAN_POINT('Origin',(49.131355399529,40.9586446004712,-260.));
#275620=CARTESIAN_POINT('',(50.0313553995292,40.958644600471,910.));
#275621=CARTESIAN_POINT('Origin',(50.0313553995292,35.108644600471,910.));
#275622=CARTESIAN_POINT('',(50.0313553995293,35.1086446004709,1282.35584962783));
#275623=CARTESIAN_POINT('',(50.0313553995293,35.108644600471,1282.35584962783));
#275624=CARTESIAN_POINT('',(50.031355399529,35.1086446004712,-260.));
#275625=CARTESIAN_POINT('',(50.031355399529,35.1086446004712,-260.));
#275626=CARTESIAN_POINT('',(50.0313553995292,35.108644600471,910.));
#275627=CARTESIAN_POINT('Origin',(50.9313553995292,35.108644600471,910.));
#275628=CARTESIAN_POINT('',(50.9313553995293,34.2086446004709,1282.35584962783));
#275629=CARTESIAN_POINT('Origin',(50.9313553995293,35.1086446004709,1282.35584962783));
#275630=CARTESIAN_POINT('',(50.931355399529,34.2086446004712,-260.));
#275631=CARTESIAN_POINT('Origin',(50.931355399529,35.1086446004712,-260.));
#275632=CARTESIAN_POINT('',(50.9313553995292,34.208644600471,910.));
#275633=CARTESIAN_POINT('Origin',(53.0013553995292,34.208644600471,910.));
#275634=CARTESIAN_POINT('',(53.0013553995293,34.2086446004709,1282.35584962783));
#275635=CARTESIAN_POINT('',(53.0013553995292,34.2086446004709,1282.35584962783));
#275636=CARTESIAN_POINT('',(53.001355399529,34.208644600471,-260.));
#275637=CARTESIAN_POINT('',(53.001355399529,34.2086446004712,-260.));
#275638=CARTESIAN_POINT('',(53.0013553995292,34.208644600471,910.));
#275639=CARTESIAN_POINT('Origin',(53.0013553995292,35.198644600471,910.));
#275640=CARTESIAN_POINT('',(53.0013553995293,35.1986446004709,1282.35584962783));
#275641=CARTESIAN_POINT('',(53.0013553995293,35.198644600471,1282.35584962783));
#275642=CARTESIAN_POINT('',(53.001355399529,35.1986446004712,-260.));
#275643=CARTESIAN_POINT('',(53.001355399529,35.1986446004712,-260.));
#275644=CARTESIAN_POINT('',(53.0013553995292,35.198644600471,910.));
#275645=CARTESIAN_POINT('Origin',(53.9913553995292,35.198644600471,910.));
#275646=CARTESIAN_POINT('',(53.9913553995293,35.1986446004709,1282.35584962783));
#275647=CARTESIAN_POINT('',(53.9913553995292,35.1986446004709,1282.35584962783));
#275648=CARTESIAN_POINT('',(53.991355399529,35.198644600471,-260.));
#275649=CARTESIAN_POINT('',(53.991355399529,35.1986446004712,-260.));
#275650=CARTESIAN_POINT('',(53.9913553995292,35.198644600471,910.));
#275651=CARTESIAN_POINT('Origin',(53.9913553995292,35.198644600471,910.));
#275652=CARTESIAN_POINT('',(53.9913553995293,50.3510446004709,1282.35584962783));
#275653=CARTESIAN_POINT('',(53.9913553995293,35.198644600471,1282.35584962783));
#275654=CARTESIAN_POINT('',(53.9913553995291,50.3510446004712,-260.));
#275655=CARTESIAN_POINT('',(53.991355399529,35.1986446004712,-260.));
#275656=CARTESIAN_POINT('',(53.9913553995293,50.3510446004709,910.));
#275657=CARTESIAN_POINT('Origin',(50.3337553995292,50.3510446004709,910.));
#275658=CARTESIAN_POINT('',(50.3337553995293,54.0086446004709,1282.35584962783));
#275659=CARTESIAN_POINT('Origin',(50.3337553995293,50.3510446004709,1282.35584962783));
#275660=CARTESIAN_POINT('',(50.3337553995292,54.0086446004712,-260.));
#275661=CARTESIAN_POINT('Origin',(50.333755399529,50.3510446004712,-260.));
#275662=CARTESIAN_POINT('',(50.3337553995292,54.008644600471,910.));
#275663=CARTESIAN_POINT('Origin',(35.1813553995293,54.0086446004711,910.));
#275664=CARTESIAN_POINT('',(35.1813553995294,54.008644600471,1282.35584962783));
#275665=CARTESIAN_POINT('',(35.1813553995293,54.008644600471,1282.35584962783));
#275666=CARTESIAN_POINT('',(35.1813553995291,54.0086446004713,-260.));
#275667=CARTESIAN_POINT('',(35.1813553995291,54.0086446004713,-260.));
#275668=CARTESIAN_POINT('',(35.1813553995293,54.0086446004711,910.));
#275669=CARTESIAN_POINT('Origin',(35.1813553995293,54.0086446004711,910.));
#275670=CARTESIAN_POINT('',(35.1813553995294,53.018644600471,1282.35584962783));
#275671=CARTESIAN_POINT('',(35.1813553995294,54.0086446004711,1282.35584962783));
#275672=CARTESIAN_POINT('',(35.1813553995293,53.0186446004713,-260.));
#275673=CARTESIAN_POINT('',(35.1813553995291,54.0086446004713,-260.));
#275674=CARTESIAN_POINT('',(35.1813553995293,53.0186446004711,910.));
#275675=CARTESIAN_POINT('Origin',(35.1813553995293,53.0186446004711,910.));
#275676=CARTESIAN_POINT('',(34.1913553995294,53.018644600471,1282.35584962783));
#275677=CARTESIAN_POINT('',(35.1813553995293,53.018644600471,1282.35584962783));
#275678=CARTESIAN_POINT('',(34.1913553995291,53.0186446004713,-260.));
#275679=CARTESIAN_POINT('',(35.1813553995291,53.0186446004713,-260.));
#275680=CARTESIAN_POINT('',(34.1913553995293,53.0186446004711,910.));
#275681=CARTESIAN_POINT('Origin',(34.1913553995293,53.0186446004711,910.));
#275682=CARTESIAN_POINT('',(34.1913553995293,50.948644600471,1282.35584962783));
#275683=CARTESIAN_POINT('',(34.1913553995294,53.0186446004711,1282.35584962783));
#275684=CARTESIAN_POINT('',(34.1913553995291,50.9486446004713,-260.));
#275685=CARTESIAN_POINT('',(34.1913553995291,53.0186446004713,-260.));
#275686=CARTESIAN_POINT('',(34.1913553995293,50.9486446004711,910.));
#275687=CARTESIAN_POINT('Origin',(35.0913553995293,50.948644600471,910.));
#275688=CARTESIAN_POINT('',(35.0913553995293,50.048644600471,1282.35584962783));
#275689=CARTESIAN_POINT('Origin',(35.0913553995293,50.948644600471,1282.35584962783));
#275690=CARTESIAN_POINT('',(35.091355399529,50.0486446004713,-260.));
#275691=CARTESIAN_POINT('Origin',(35.091355399529,50.9486446004713,-260.));
#275692=CARTESIAN_POINT('',(35.0913553995293,50.0486446004711,910.));
#275693=CARTESIAN_POINT('Origin',(35.0913553995293,50.0486446004711,910.));
#275694=CARTESIAN_POINT('',(40.9413553995293,50.048644600471,1282.35584962783));
#275695=CARTESIAN_POINT('',(35.0913553995293,50.048644600471,1282.35584962783));
#275696=CARTESIAN_POINT('',(40.9413553995291,50.0486446004712,-260.));
#275697=CARTESIAN_POINT('',(35.091355399529,50.0486446004713,-260.));
#275698=CARTESIAN_POINT('',(40.9413553995293,50.048644600471,910.));
#275699=CARTESIAN_POINT('Origin',(40.9413553995293,49.148644600471,910.));
#275700=CARTESIAN_POINT('',(41.8413553995293,49.148644600471,1282.35584962783));
#275701=CARTESIAN_POINT('Origin',(40.9413553995293,49.148644600471,1282.35584962783));
#275702=CARTESIAN_POINT('',(41.841355399529,49.1486446004712,-260.));
#275703=CARTESIAN_POINT('Origin',(40.9413553995291,49.1486446004712,-260.));
#275704=CARTESIAN_POINT('',(41.8413553995293,49.148644600471,910.));
#275705=CARTESIAN_POINT('Origin',(41.8413553995293,49.148644600471,910.));
#275706=CARTESIAN_POINT('',(41.8413553995293,45.4134173219462,1282.35584962783));
#275707=CARTESIAN_POINT('',(41.8413553995293,49.148644600471,1282.35584962783));
#275708=CARTESIAN_POINT('',(41.841355399529,45.4134173219465,-260.));
#275709=CARTESIAN_POINT('',(41.841355399529,49.1486446004712,-260.));
#275710=CARTESIAN_POINT('',(41.8413553995293,45.4134173219463,910.));
#275711=CARTESIAN_POINT('Origin',(40.9413553995293,45.4134173219463,910.));
#275712=CARTESIAN_POINT('',(41.5777515025972,44.7770212188783,1282.35584962783));
#275713=CARTESIAN_POINT('Origin',(40.9413553995293,45.4134173219462,1282.35584962783));
#275714=CARTESIAN_POINT('',(41.5777515025969,44.7770212188786,-260.));
#275715=CARTESIAN_POINT('Origin',(40.941355399529,45.4134173219465,-260.));
#275716=CARTESIAN_POINT('',(41.5777515025972,44.7770212188784,910.));
#275717=CARTESIAN_POINT('Origin',(41.5777515025972,44.7770212188784,910.));
#275718=CARTESIAN_POINT('',(34.8729787811219,38.0722484974031,1282.35584962783));
#275719=CARTESIAN_POINT('',(41.5777515025972,44.7770212188783,1282.35584962783));
#275720=CARTESIAN_POINT('',(34.8729787811217,38.0722484974034,-260.));
#275721=CARTESIAN_POINT('',(41.5777515025969,44.7770212188786,-260.));
#275722=CARTESIAN_POINT('',(34.8729787811219,38.0722484974032,910.));
#275723=CARTESIAN_POINT('Origin',(34.236582678054,38.7086446004711,910.));
#275724=CARTESIAN_POINT('',(34.236582678054,37.808644600471,1282.35584962783));
#275725=CARTESIAN_POINT('Origin',(34.2365826780541,38.708644600471,1282.35584962783));
#275726=CARTESIAN_POINT('',(34.236582678054,37.8086446004713,-260.));
#275727=CARTESIAN_POINT('Origin',(34.2365826780538,38.7086446004713,-260.));
#275728=CARTESIAN_POINT('',(34.236582678054,37.8086446004711,910.));
#275729=CARTESIAN_POINT('Origin',(34.236582678054,37.8086446004711,910.));
#275730=CARTESIAN_POINT('',(34.236582678054,37.808644600471,1282.35584962783));
#275731=CARTESIAN_POINT('',(34.2365826780538,37.8086446004713,-260.));
#275732=CARTESIAN_POINT('Origin',(37.7913553995291,-28.5127888288977,910.));
#275733=CARTESIAN_POINT('',(37.7913553995291,-28.5127888288979,1282.35584962783));
#275734=CARTESIAN_POINT('',(36.9129553995291,-26.9913553995294,1282.35584962783));
#275735=CARTESIAN_POINT('',(37.791355399529,-28.5127888288978,1282.35584962783));
#275736=CARTESIAN_POINT('',(37.7913553995293,-28.5127888288977,-260.));
#275737=CARTESIAN_POINT('',(37.7913553995291,-28.5127888288977,910.));
#275738=CARTESIAN_POINT('',(36.9129553995288,-26.9913553995292,-260.));
#275739=CARTESIAN_POINT('',(37.7913553995291,-28.5127888288973,-260.));
#275740=CARTESIAN_POINT('',(36.9129553995291,-26.9913553995292,910.));
#275741=CARTESIAN_POINT('Origin',(37.7913553995291,-25.4699219701607,910.));
#275742=CARTESIAN_POINT('',(37.7913553995291,-25.4699219701609,1282.35584962783));
#275743=CARTESIAN_POINT('',(37.7913553995292,-25.4699219701608,1282.35584962783));
#275744=CARTESIAN_POINT('',(37.7913553995291,-25.4699219701607,-260.));
#275745=CARTESIAN_POINT('',(37.7913553995291,-25.4699219701603,-260.));
#275746=CARTESIAN_POINT('',(37.7913553995291,-25.4699219701607,910.));
#275747=CARTESIAN_POINT('Origin',(37.7913553995291,-19.7461281210045,910.));
#275748=CARTESIAN_POINT('',(37.7913553995291,-19.7461281210046,1282.35584962783));
#275749=CARTESIAN_POINT('',(37.7913553995291,-19.7461281210045,1282.35584962783));
#275750=CARTESIAN_POINT('',(37.7913553995291,-19.7461281210041,-260.));
#275751=CARTESIAN_POINT('',(37.7913553995291,-19.7461281210041,-260.));
#275752=CARTESIAN_POINT('',(37.7913553995291,-19.7461281210045,910.));
#275753=CARTESIAN_POINT('Origin',(38.6913553995291,-19.7461281210045,910.));
#275754=CARTESIAN_POINT('',(38.0549592964612,-19.1097320179367,1282.35584962783));
#275755=CARTESIAN_POINT('Origin',(38.6913553995291,-19.7461281210046,1282.35584962783));
#275756=CARTESIAN_POINT('',(38.0549592964612,-19.1097320179362,-260.));
#275757=CARTESIAN_POINT('Origin',(38.6913553995291,-19.7461281210041,-260.));
#275758=CARTESIAN_POINT('',(38.0549592964612,-19.1097320179366,910.));
#275759=CARTESIAN_POINT('Origin',(44.7597320179365,-12.4049592964613,910.));
#275760=CARTESIAN_POINT('',(44.7597320179365,-12.4049592964615,1282.35584962783));
#275761=CARTESIAN_POINT('',(44.7597320179365,-12.4049592964614,1282.35584962783));
#275762=CARTESIAN_POINT('',(44.7597320179365,-12.4049592964609,-260.));
#275763=CARTESIAN_POINT('',(44.7597320179365,-12.4049592964609,-260.));
#275764=CARTESIAN_POINT('',(44.7597320179365,-12.4049592964613,910.));
#275765=CARTESIAN_POINT('Origin',(45.3961281210043,-13.0413553995292,910.));
#275766=CARTESIAN_POINT('',(45.3961281210043,-12.1413553995294,1282.35584962783));
#275767=CARTESIAN_POINT('Origin',(45.3961281210043,-13.0413553995294,1282.35584962783));
#275768=CARTESIAN_POINT('',(45.3961281210043,-12.1413553995288,-260.));
#275769=CARTESIAN_POINT('Origin',(45.3961281210043,-13.0413553995288,-260.));
#275770=CARTESIAN_POINT('',(45.3961281210043,-12.1413553995292,910.));
#275771=CARTESIAN_POINT('Origin',(49.1313553995291,-12.1413553995292,910.));
#275772=CARTESIAN_POINT('',(49.1313553995291,-12.1413553995294,1282.35584962783));
#275773=CARTESIAN_POINT('',(49.1313553995291,-12.1413553995294,1282.35584962783));
#275774=CARTESIAN_POINT('',(49.1313553995291,-12.1413553995288,-260.));
#275775=CARTESIAN_POINT('',(49.1313553995291,-12.1413553995288,-260.));
#275776=CARTESIAN_POINT('',(49.1313553995291,-12.1413553995292,910.));
#275777=CARTESIAN_POINT('Origin',(49.1313553995291,-13.0413553995292,910.));
#275778=CARTESIAN_POINT('',(50.0313553995291,-13.0413553995294,1282.35584962783));
#275779=CARTESIAN_POINT('Origin',(49.1313553995291,-13.0413553995294,1282.35584962783));
#275780=CARTESIAN_POINT('',(50.0313553995291,-13.0413553995288,-260.));
#275781=CARTESIAN_POINT('Origin',(49.1313553995291,-13.0413553995288,-260.));
#275782=CARTESIAN_POINT('',(50.0313553995291,-13.0413553995292,910.));
#275783=CARTESIAN_POINT('Origin',(50.0313553995291,-18.8913553995292,910.));
#275784=CARTESIAN_POINT('',(50.0313553995291,-18.8913553995294,1282.35584962783));
#275785=CARTESIAN_POINT('',(50.0313553995291,-18.8913553995292,1282.35584962783));
#275786=CARTESIAN_POINT('',(50.0313553995291,-18.8913553995288,-260.));
#275787=CARTESIAN_POINT('',(50.0313553995291,-18.8913553995288,-260.));
#275788=CARTESIAN_POINT('',(50.0313553995291,-18.8913553995292,910.));
#275789=CARTESIAN_POINT('Origin',(50.9313553995291,-18.8913553995292,910.));
#275790=CARTESIAN_POINT('',(50.9313553995291,-19.7913553995294,1282.35584962783));
#275791=CARTESIAN_POINT('Origin',(50.9313553995291,-18.8913553995294,1282.35584962783));
#275792=CARTESIAN_POINT('',(50.9313553995291,-19.7913553995288,-260.));
#275793=CARTESIAN_POINT('Origin',(50.9313553995291,-18.8913553995288,-260.));
#275794=CARTESIAN_POINT('',(50.9313553995291,-19.7913553995292,910.));
#275795=CARTESIAN_POINT('Origin',(53.0013553995291,-19.7913553995292,910.));
#275796=CARTESIAN_POINT('',(53.0013553995291,-19.7913553995294,1282.35584962783));
#275797=CARTESIAN_POINT('',(53.0013553995291,-19.7913553995294,1282.35584962783));
#275798=CARTESIAN_POINT('',(53.0013553995291,-19.7913553995292,-260.));
#275799=CARTESIAN_POINT('',(53.0013553995291,-19.7913553995288,-260.));
#275800=CARTESIAN_POINT('',(53.0013553995291,-19.7913553995292,910.));
#275801=CARTESIAN_POINT('Origin',(53.0013553995291,-18.8013553995292,910.));
#275802=CARTESIAN_POINT('',(53.0013553995291,-18.8013553995294,1282.35584962783));
#275803=CARTESIAN_POINT('',(53.0013553995291,-18.8013553995292,1282.35584962783));
#275804=CARTESIAN_POINT('',(53.0013553995291,-18.8013553995288,-260.));
#275805=CARTESIAN_POINT('',(53.0013553995291,-18.8013553995288,-260.));
#275806=CARTESIAN_POINT('',(53.0013553995291,-18.8013553995292,910.));
#275807=CARTESIAN_POINT('Origin',(53.9913553995291,-18.8013553995292,910.));
#275808=CARTESIAN_POINT('',(53.9913553995291,-18.8013553995294,1282.35584962783));
#275809=CARTESIAN_POINT('',(53.9913553995291,-18.8013553995288,-260.));
#275810=CARTESIAN_POINT('Origin',(18.8013553995289,-53.9913553995292,910.));
#275811=CARTESIAN_POINT('',(-18.818644600472,-53.9913553995291,1282.35584962783));
#275812=CARTESIAN_POINT('',(18.8013553995289,-53.9913553995293,1282.35584962783));
#275813=CARTESIAN_POINT('',(18.8013553995289,-53.9913553995293,1282.35584962783));
#275814=CARTESIAN_POINT('',(-18.8186446004719,-53.9913553995285,-260.));
#275815=CARTESIAN_POINT('',(-18.8186446004719,-53.991355399529,910.));
#275816=CARTESIAN_POINT('',(18.8013553995289,-53.9913553995292,-260.));
#275817=CARTESIAN_POINT('',(18.8013553995289,-53.9913553995287,-260.));
#275818=CARTESIAN_POINT('',(18.8013553995289,-53.9913553995292,910.));
#275819=CARTESIAN_POINT('Origin',(18.8013553995289,-53.9913553995292,910.));
#275820=CARTESIAN_POINT('',(18.8013553995289,-53.0013553995293,1282.35584962783));
#275821=CARTESIAN_POINT('',(18.8013553995289,-53.9913553995292,1282.35584962783));
#275822=CARTESIAN_POINT('',(18.8013553995289,-53.0013553995287,-260.));
#275823=CARTESIAN_POINT('',(18.8013553995289,-53.9913553995287,-260.));
#275824=CARTESIAN_POINT('',(18.8013553995289,-53.0013553995292,910.));
#275825=CARTESIAN_POINT('Origin',(18.8013553995289,-53.0013553995292,910.));
#275826=CARTESIAN_POINT('',(19.7913553995289,-53.0013553995293,1282.35584962783));
#275827=CARTESIAN_POINT('',(18.8013553995289,-53.0013553995293,1282.35584962783));
#275828=CARTESIAN_POINT('',(19.7913553995289,-53.0013553995292,-260.));
#275829=CARTESIAN_POINT('',(18.8013553995289,-53.0013553995287,-260.));
#275830=CARTESIAN_POINT('',(19.7913553995289,-53.0013553995292,910.));
#275831=CARTESIAN_POINT('Origin',(19.7913553995289,-53.0013553995292,910.));
#275832=CARTESIAN_POINT('',(19.7913553995289,-50.9313553995293,1282.35584962783));
#275833=CARTESIAN_POINT('',(19.7913553995289,-53.0013553995292,1282.35584962783));
#275834=CARTESIAN_POINT('',(19.7913553995289,-50.9313553995287,-260.));
#275835=CARTESIAN_POINT('',(19.7913553995289,-53.0013553995287,-260.));
#275836=CARTESIAN_POINT('',(19.7913553995289,-50.9313553995292,910.));
#275837=CARTESIAN_POINT('Origin',(18.8913553995289,-50.9313553995292,910.));
#275838=CARTESIAN_POINT('',(18.8913553995289,-50.0313553995293,1282.35584962783));
#275839=CARTESIAN_POINT('Origin',(18.8913553995289,-50.9313553995293,1282.35584962783));
#275840=CARTESIAN_POINT('',(18.8913553995289,-50.0313553995287,-260.));
#275841=CARTESIAN_POINT('Origin',(18.8913553995289,-50.9313553995287,-260.));
#275842=CARTESIAN_POINT('',(18.8913553995289,-50.0313553995292,910.));
#275843=CARTESIAN_POINT('Origin',(18.8913553995289,-50.0313553995292,910.));
#275844=CARTESIAN_POINT('',(13.0413553995289,-50.0313553995292,1282.35584962783));
#275845=CARTESIAN_POINT('',(18.8913553995289,-50.0313553995293,1282.35584962783));
#275846=CARTESIAN_POINT('',(13.0413553995289,-50.0313553995287,-260.));
#275847=CARTESIAN_POINT('',(18.8913553995289,-50.0313553995287,-260.));
#275848=CARTESIAN_POINT('',(13.0413553995289,-50.0313553995291,910.));
#275849=CARTESIAN_POINT('Origin',(13.0413553995289,-49.1313553995291,910.));
#275850=CARTESIAN_POINT('',(12.1413553995289,-49.1313553995292,1282.35584962783));
#275851=CARTESIAN_POINT('Origin',(13.0413553995289,-49.1313553995292,1282.35584962783));
#275852=CARTESIAN_POINT('',(12.1413553995289,-49.1313553995291,-260.));
#275853=CARTESIAN_POINT('Origin',(13.0413553995289,-49.1313553995287,-260.));
#275854=CARTESIAN_POINT('',(12.1413553995289,-49.1313553995291,910.));
#275855=CARTESIAN_POINT('Origin',(12.1413553995289,-49.1313553995291,910.));
#275856=CARTESIAN_POINT('',(12.141355399529,-45.3961281210045,1282.35584962783));
#275857=CARTESIAN_POINT('',(12.1413553995289,-49.1313553995291,1282.35584962783));
#275858=CARTESIAN_POINT('',(12.141355399529,-45.3961281210039,-260.));
#275859=CARTESIAN_POINT('',(12.1413553995289,-49.1313553995287,-260.));
#275860=CARTESIAN_POINT('',(12.141355399529,-45.3961281210044,910.));
#275861=CARTESIAN_POINT('Origin',(13.041355399529,-45.3961281210044,910.));
#275862=CARTESIAN_POINT('',(12.4049592964611,-44.7597320179366,1282.35584962783));
#275863=CARTESIAN_POINT('Origin',(13.041355399529,-45.3961281210045,1282.35584962783));
#275864=CARTESIAN_POINT('',(12.4049592964611,-44.759732017936,-260.));
#275865=CARTESIAN_POINT('Origin',(13.041355399529,-45.3961281210039,-260.));
#275866=CARTESIAN_POINT('',(12.4049592964611,-44.7597320179365,910.));
#275867=CARTESIAN_POINT('Origin',(12.4049592964611,-44.7597320179365,910.));
#275868=CARTESIAN_POINT('',(19.1097320179364,-38.0549592964614,1282.35584962783));
#275869=CARTESIAN_POINT('',(12.4049592964611,-44.7597320179365,1282.35584962783));
#275870=CARTESIAN_POINT('',(19.1097320179364,-38.0549592964608,-260.));
#275871=CARTESIAN_POINT('',(12.4049592964611,-44.759732017936,-260.));
#275872=CARTESIAN_POINT('',(19.1097320179364,-38.0549592964613,910.));
#275873=CARTESIAN_POINT('Origin',(19.7461281210043,-38.6913553995292,910.));
#275874=CARTESIAN_POINT('',(19.7461281210043,-37.7913553995293,1282.35584962783));
#275875=CARTESIAN_POINT('Origin',(19.7461281210043,-38.6913553995293,1282.35584962783));
#275876=CARTESIAN_POINT('',(19.7461281210043,-37.7913553995287,-260.));
#275877=CARTESIAN_POINT('Origin',(19.7461281210043,-38.6913553995287,-260.));
#275878=CARTESIAN_POINT('',(19.7461281210043,-37.7913553995292,910.));
#275879=CARTESIAN_POINT('Origin',(19.7461281210043,-37.7913553995292,910.));
#275880=CARTESIAN_POINT('',(25.4699219701605,-37.7913553995294,1282.35584962783));
#275881=CARTESIAN_POINT('',(19.7461281210043,-37.7913553995293,1282.35584962783));
#275882=CARTESIAN_POINT('',(25.4699219701605,-37.7913553995288,-260.));
#275883=CARTESIAN_POINT('',(19.7461281210043,-37.7913553995287,-260.));
#275884=CARTESIAN_POINT('',(25.4699219701605,-37.7913553995292,910.));
#275885=CARTESIAN_POINT('Origin',(25.4699219701605,-37.7913553995292,910.));
#275886=CARTESIAN_POINT('',(26.9913553995291,-36.9129553995294,1282.35584962783));
#275887=CARTESIAN_POINT('',(25.4699219701606,-37.7913553995293,1282.35584962783));
#275888=CARTESIAN_POINT('',(26.9913553995291,-36.9129553995288,-260.));
#275889=CARTESIAN_POINT('',(25.4699219701605,-37.7913553995288,-260.));
#275890=CARTESIAN_POINT('',(26.9913553995291,-36.9129553995292,910.));
#275891=CARTESIAN_POINT('Origin',(28.5127888288976,-37.7913553995292,910.));
#275892=CARTESIAN_POINT('',(28.5127888288976,-37.7913553995294,1282.35584962783));
#275893=CARTESIAN_POINT('',(28.5127888288975,-37.7913553995293,1282.35584962783));
#275894=CARTESIAN_POINT('',(28.5127888288976,-37.7913553995288,-260.));
#275895=CARTESIAN_POINT('',(28.5127888288976,-37.7913553995288,-260.));
#275896=CARTESIAN_POINT('',(28.5127888288976,-37.7913553995292,910.));
#275897=CARTESIAN_POINT('Origin',(34.2365826780538,-37.7913553995292,910.));
#275898=CARTESIAN_POINT('',(34.2365826780538,-37.7913553995294,1282.35584962783));
#275899=CARTESIAN_POINT('',(34.2365826780538,-37.7913553995294,1282.35584962783));
#275900=CARTESIAN_POINT('',(34.2365826780538,-37.7913553995288,-260.));
#275901=CARTESIAN_POINT('',(34.2365826780538,-37.7913553995288,-260.));
#275902=CARTESIAN_POINT('',(34.2365826780538,-37.7913553995292,910.));
#275903=CARTESIAN_POINT('Origin',(34.2365826780538,-38.6913553995292,910.));
#275904=CARTESIAN_POINT('',(34.8729787811217,-38.0549592964615,1282.35584962783));
#275905=CARTESIAN_POINT('Origin',(34.2365826780538,-38.6913553995294,1282.35584962783));
#275906=CARTESIAN_POINT('',(34.8729787811217,-38.0549592964609,-260.));
#275907=CARTESIAN_POINT('Origin',(34.2365826780538,-38.6913553995288,-260.));
#275908=CARTESIAN_POINT('',(34.8729787811217,-38.0549592964613,910.));
#275909=CARTESIAN_POINT('Origin',(41.577751502597,-44.7597320179366,910.));
#275910=CARTESIAN_POINT('',(41.577751502597,-44.7597320179367,1282.35584962783));
#275911=CARTESIAN_POINT('',(41.5777515025969,-44.7597320179367,1282.35584962783));
#275912=CARTESIAN_POINT('',(41.577751502597,-44.7597320179362,-260.));
#275913=CARTESIAN_POINT('',(41.577751502597,-44.7597320179362,-260.));
#275914=CARTESIAN_POINT('',(41.577751502597,-44.7597320179366,910.));
#275915=CARTESIAN_POINT('Origin',(40.9413553995291,-45.3961281210045,910.));
#275916=CARTESIAN_POINT('',(41.8413553995291,-45.3961281210046,1282.35584962783));
#275917=CARTESIAN_POINT('Origin',(40.9413553995291,-45.3961281210046,1282.35584962783));
#275918=CARTESIAN_POINT('',(41.8413553995291,-45.396128121004,-260.));
#275919=CARTESIAN_POINT('Origin',(40.9413553995291,-45.396128121004,-260.));
#275920=CARTESIAN_POINT('',(41.8413553995291,-45.3961281210045,910.));
#275921=CARTESIAN_POINT('Origin',(41.8413553995291,-49.1313553995292,910.));
#275922=CARTESIAN_POINT('',(41.8413553995291,-49.1313553995293,1282.35584962783));
#275923=CARTESIAN_POINT('',(41.8413553995291,-49.1313553995292,1282.35584962783));
#275924=CARTESIAN_POINT('',(41.8413553995291,-49.1313553995288,-260.));
#275925=CARTESIAN_POINT('',(41.8413553995291,-49.1313553995288,-260.));
#275926=CARTESIAN_POINT('',(41.8413553995291,-49.1313553995292,910.));
#275927=CARTESIAN_POINT('Origin',(40.9413553995291,-49.1313553995292,910.));
#275928=CARTESIAN_POINT('',(40.9413553995291,-50.0313553995293,1282.35584962783));
#275929=CARTESIAN_POINT('Origin',(40.9413553995291,-49.1313553995294,1282.35584962783));
#275930=CARTESIAN_POINT('',(40.9413553995291,-50.0313553995288,-260.));
#275931=CARTESIAN_POINT('Origin',(40.9413553995291,-49.1313553995288,-260.));
#275932=CARTESIAN_POINT('',(40.9413553995291,-50.0313553995292,910.));
#275933=CARTESIAN_POINT('Origin',(35.0913553995291,-50.0313553995292,910.));
#275934=CARTESIAN_POINT('',(35.0913553995291,-50.0313553995294,1282.35584962783));
#275935=CARTESIAN_POINT('',(35.0913553995291,-50.0313553995294,1282.35584962783));
#275936=CARTESIAN_POINT('',(35.0913553995291,-50.0313553995288,-260.));
#275937=CARTESIAN_POINT('',(35.0913553995291,-50.0313553995288,-260.));
#275938=CARTESIAN_POINT('',(35.0913553995291,-50.0313553995292,910.));
#275939=CARTESIAN_POINT('Origin',(35.0913553995291,-50.9313553995292,910.));
#275940=CARTESIAN_POINT('',(34.1913553995291,-50.9313553995294,1282.35584962783));
#275941=CARTESIAN_POINT('Origin',(35.0913553995291,-50.9313553995294,1282.35584962783));
#275942=CARTESIAN_POINT('',(34.1913553995291,-50.9313553995288,-260.));
#275943=CARTESIAN_POINT('Origin',(35.0913553995291,-50.9313553995288,-260.));
#275944=CARTESIAN_POINT('',(34.1913553995291,-50.9313553995292,910.));
#275945=CARTESIAN_POINT('Origin',(34.1913553995291,-53.0013553995292,910.));
#275946=CARTESIAN_POINT('',(34.1913553995291,-53.0013553995294,1282.35584962783));
#275947=CARTESIAN_POINT('',(34.1913553995291,-53.0013553995292,1282.35584962783));
#275948=CARTESIAN_POINT('',(34.1913553995291,-53.0013553995288,-260.));
#275949=CARTESIAN_POINT('',(34.1913553995291,-53.0013553995288,-260.));
#275950=CARTESIAN_POINT('',(34.1913553995291,-53.0013553995292,910.));
#275951=CARTESIAN_POINT('Origin',(35.1813553995291,-53.0013553995292,910.));
#275952=CARTESIAN_POINT('',(35.1813553995291,-53.0013553995294,1282.35584962783));
#275953=CARTESIAN_POINT('',(35.1813553995291,-53.0013553995294,1282.35584962783));
#275954=CARTESIAN_POINT('',(35.1813553995291,-53.0013553995288,-260.));
#275955=CARTESIAN_POINT('',(35.1813553995291,-53.0013553995288,-260.));
#275956=CARTESIAN_POINT('',(35.1813553995291,-53.0013553995292,910.));
#275957=CARTESIAN_POINT('Origin',(35.1813553995291,-53.9913553995292,910.));
#275958=CARTESIAN_POINT('',(35.1813553995291,-53.9913553995294,1282.35584962783));
#275959=CARTESIAN_POINT('',(35.1813553995291,-53.9913553995292,1282.35584962783));
#275960=CARTESIAN_POINT('',(35.1813553995291,-53.9913553995288,-260.));
#275961=CARTESIAN_POINT('',(35.1813553995291,-53.9913553995288,-260.));
#275962=CARTESIAN_POINT('',(35.1813553995291,-53.9913553995292,910.));
#275963=CARTESIAN_POINT('Origin',(35.1813553995291,-53.9913553995292,910.));
#275964=CARTESIAN_POINT('',(50.333755399529,-53.9913553995294,1282.35584962783));
#275965=CARTESIAN_POINT('',(35.1813553995291,-53.9913553995294,1282.35584962783));
#275966=CARTESIAN_POINT('',(50.333755399529,-53.9913553995288,-260.));
#275967=CARTESIAN_POINT('',(35.1813553995291,-53.9913553995288,-260.));
#275968=CARTESIAN_POINT('',(50.333755399529,-53.9913553995292,910.));
#275969=CARTESIAN_POINT('Origin',(50.333755399529,-50.3337553995292,910.));
#275970=CARTESIAN_POINT('',(53.9913553995291,-50.3337553995293,1282.35584962783));
#275971=CARTESIAN_POINT('Origin',(50.333755399529,-50.3337553995293,1282.35584962783));
#275972=CARTESIAN_POINT('',(53.9913553995291,-50.3337553995292,-260.));
#275973=CARTESIAN_POINT('Origin',(50.333755399529,-50.3337553995287,-260.));
#275974=CARTESIAN_POINT('',(53.9913553995291,-50.3337553995292,910.));
#275975=CARTESIAN_POINT('Origin',(53.9913553995291,-35.1813553995292,910.));
#275976=CARTESIAN_POINT('',(53.9913553995291,-35.1813553995294,1282.35584962783));
#275977=CARTESIAN_POINT('',(53.9913553995291,-35.1813553995292,1282.35584962783));
#275978=CARTESIAN_POINT('',(53.9913553995291,-35.1813553995288,-260.));
#275979=CARTESIAN_POINT('',(53.9913553995291,-35.1813553995288,-260.));
#275980=CARTESIAN_POINT('',(53.9913553995291,-35.1813553995292,910.));
#275981=CARTESIAN_POINT('Origin',(53.9913553995291,-35.1813553995292,910.));
#275982=CARTESIAN_POINT('',(53.0013553995291,-35.1813553995294,1282.35584962783));
#275983=CARTESIAN_POINT('',(53.9913553995291,-35.1813553995294,1282.35584962783));
#275984=CARTESIAN_POINT('',(53.0013553995291,-35.1813553995292,-260.));
#275985=CARTESIAN_POINT('',(53.9913553995291,-35.1813553995288,-260.));
#275986=CARTESIAN_POINT('',(53.0013553995291,-35.1813553995292,910.));
#275987=CARTESIAN_POINT('Origin',(53.0013553995291,-35.1813553995292,910.));
#275988=CARTESIAN_POINT('',(53.0013553995291,-34.1913553995294,1282.35584962783));
#275989=CARTESIAN_POINT('',(53.0013553995291,-35.1813553995292,1282.35584962783));
#275990=CARTESIAN_POINT('',(53.0013553995291,-34.1913553995288,-260.));
#275991=CARTESIAN_POINT('',(53.0013553995291,-35.1813553995288,-260.));
#275992=CARTESIAN_POINT('',(53.0013553995291,-34.1913553995292,910.));
#275993=CARTESIAN_POINT('Origin',(53.0013553995291,-34.1913553995292,910.));
#275994=CARTESIAN_POINT('',(50.9313553995291,-34.1913553995294,1282.35584962783));
#275995=CARTESIAN_POINT('',(53.0013553995291,-34.1913553995294,1282.35584962783));
#275996=CARTESIAN_POINT('',(50.9313553995291,-34.1913553995288,-260.));
#275997=CARTESIAN_POINT('',(53.0013553995291,-34.1913553995288,-260.));
#275998=CARTESIAN_POINT('',(50.9313553995291,-34.1913553995292,910.));
#275999=CARTESIAN_POINT('Origin',(50.9313553995291,-35.0913553995292,910.));
#276000=CARTESIAN_POINT('',(50.0313553995291,-35.0913553995294,1282.35584962783));
#276001=CARTESIAN_POINT('Origin',(50.9313553995291,-35.0913553995294,1282.35584962783));
#276002=CARTESIAN_POINT('',(50.0313553995291,-35.0913553995288,-260.));
#276003=CARTESIAN_POINT('Origin',(50.9313553995291,-35.0913553995288,-260.));
#276004=CARTESIAN_POINT('',(50.0313553995291,-35.0913553995292,910.));
#276005=CARTESIAN_POINT('Origin',(50.0313553995291,-35.0913553995292,910.));
#276006=CARTESIAN_POINT('',(50.0313553995291,-40.9413553995294,1282.35584962783));
#276007=CARTESIAN_POINT('',(50.0313553995291,-35.0913553995292,1282.35584962783));
#276008=CARTESIAN_POINT('',(50.0313553995291,-40.9413553995288,-260.));
#276009=CARTESIAN_POINT('',(50.0313553995291,-35.0913553995288,-260.));
#276010=CARTESIAN_POINT('',(50.0313553995291,-40.9413553995292,910.));
#276011=CARTESIAN_POINT('Origin',(49.1313553995291,-40.9413553995292,910.));
#276012=CARTESIAN_POINT('',(49.1313553995291,-41.8413553995294,1282.35584962783));
#276013=CARTESIAN_POINT('Origin',(49.1313553995291,-40.9413553995294,1282.35584962783));
#276014=CARTESIAN_POINT('',(49.1313553995291,-41.8413553995288,-260.));
#276015=CARTESIAN_POINT('Origin',(49.1313553995291,-40.9413553995288,-260.));
#276016=CARTESIAN_POINT('',(49.1313553995291,-41.8413553995292,910.));
#276017=CARTESIAN_POINT('Origin',(49.1313553995291,-41.8413553995292,910.));
#276018=CARTESIAN_POINT('',(45.3961281210043,-41.8413553995294,1282.35584962783));
#276019=CARTESIAN_POINT('',(49.1313553995291,-41.8413553995294,1282.35584962783));
#276020=CARTESIAN_POINT('',(45.3961281210043,-41.8413553995288,-260.));
#276021=CARTESIAN_POINT('',(49.1313553995291,-41.8413553995288,-260.));
#276022=CARTESIAN_POINT('',(45.3961281210043,-41.8413553995292,910.));
#276023=CARTESIAN_POINT('Origin',(45.3961281210043,-40.9413553995292,910.));
#276024=CARTESIAN_POINT('',(44.7597320179365,-41.5777515025973,1282.35584962783));
#276025=CARTESIAN_POINT('Origin',(45.3961281210043,-40.9413553995294,1282.35584962783));
#276026=CARTESIAN_POINT('',(44.7597320179365,-41.5777515025967,-260.));
#276027=CARTESIAN_POINT('Origin',(45.3961281210043,-40.9413553995288,-260.));
#276028=CARTESIAN_POINT('',(44.7597320179365,-41.5777515025971,910.));
#276029=CARTESIAN_POINT('Origin',(44.7597320179365,-41.5777515025971,910.));
#276030=CARTESIAN_POINT('',(38.0549592964612,-34.872978781122,1282.35584962783));
#276031=CARTESIAN_POINT('',(44.7597320179364,-41.5777515025972,1282.35584962783));
#276032=CARTESIAN_POINT('',(38.0549592964612,-34.8729787811214,-260.));
#276033=CARTESIAN_POINT('',(44.7597320179365,-41.5777515025967,-260.));
#276034=CARTESIAN_POINT('',(38.0549592964612,-34.8729787811219,910.));
#276035=CARTESIAN_POINT('Origin',(38.6913553995291,-34.236582678054,910.));
#276036=CARTESIAN_POINT('',(37.7913553995291,-34.2365826780541,1282.35584962783));
#276037=CARTESIAN_POINT('Origin',(38.6913553995291,-34.2365826780541,1282.35584962783));
#276038=CARTESIAN_POINT('',(37.7913553995291,-34.236582678054,-260.));
#276039=CARTESIAN_POINT('Origin',(38.6913553995291,-34.2365826780536,-260.));
#276040=CARTESIAN_POINT('',(37.7913553995291,-34.236582678054,910.));
#276041=CARTESIAN_POINT('Origin',(37.7913553995291,-34.236582678054,910.));
#276042=CARTESIAN_POINT('',(37.7913553995291,-34.236582678054,1282.35584962783));
#276043=CARTESIAN_POINT('',(37.7913553995291,-34.2365826780536,-260.));
#276044=CARTESIAN_POINT('Origin',(-28.5300780298402,-37.7913553995289,910.));
#276045=CARTESIAN_POINT('',(-28.5300780298403,-37.791355399529,1282.35584962783));
#276046=CARTESIAN_POINT('',(-27.0086446004718,-36.912955399529,1282.35584962783));
#276047=CARTESIAN_POINT('',(-28.5300780298402,-37.7913553995289,1282.35584962783));
#276048=CARTESIAN_POINT('',(-28.5300780298402,-37.7913553995288,-260.));
#276049=CARTESIAN_POINT('',(-28.5300780298402,-37.7913553995289,910.));
#276050=CARTESIAN_POINT('',(-27.0086446004717,-36.9129553995286,-260.));
#276051=CARTESIAN_POINT('',(-28.53007802984,-37.7913553995287,-260.));
#276052=CARTESIAN_POINT('',(-27.0086446004717,-36.9129553995289,910.));
#276053=CARTESIAN_POINT('Origin',(-25.4872111711032,-37.791355399529,910.));
#276054=CARTESIAN_POINT('',(-25.4872111711033,-37.791355399529,1282.35584962783));
#276055=CARTESIAN_POINT('',(-25.4872111711033,-37.791355399529,1282.35584962783));
#276056=CARTESIAN_POINT('',(-25.4872111711032,-37.7913553995287,-260.));
#276057=CARTESIAN_POINT('',(-25.487211171103,-37.7913553995287,-260.));
#276058=CARTESIAN_POINT('',(-25.4872111711032,-37.791355399529,910.));
#276059=CARTESIAN_POINT('Origin',(-19.763417321947,-37.791355399529,910.));
#276060=CARTESIAN_POINT('',(-19.763417321947,-37.7913553995291,1282.35584962783));
#276061=CARTESIAN_POINT('',(-19.763417321947,-37.7913553995291,1282.35584962783));
#276062=CARTESIAN_POINT('',(-19.7634173219468,-37.7913553995288,-260.));
#276063=CARTESIAN_POINT('',(-19.7634173219468,-37.7913553995288,-260.));
#276064=CARTESIAN_POINT('',(-19.763417321947,-37.791355399529,910.));
#276065=CARTESIAN_POINT('Origin',(-19.763417321947,-38.691355399529,910.));
#276066=CARTESIAN_POINT('',(-19.1270212188791,-38.0549592964612,1282.35584962783));
#276067=CARTESIAN_POINT('Origin',(-19.763417321947,-38.6913553995291,1282.35584962783));
#276068=CARTESIAN_POINT('',(-19.1270212188789,-38.0549592964609,-260.));
#276069=CARTESIAN_POINT('Origin',(-19.7634173219468,-38.6913553995288,-260.));
#276070=CARTESIAN_POINT('',(-19.1270212188791,-38.0549592964611,910.));
#276071=CARTESIAN_POINT('Origin',(-12.4222484974039,-44.7597320179364,910.));
#276072=CARTESIAN_POINT('',(-12.422248497404,-44.7597320179365,1282.35584962783));
#276073=CARTESIAN_POINT('',(-12.422248497404,-44.7597320179365,1282.35584962783));
#276074=CARTESIAN_POINT('',(-12.4222484974037,-44.7597320179362,-260.));
#276075=CARTESIAN_POINT('',(-12.4222484974037,-44.7597320179362,-260.));
#276076=CARTESIAN_POINT('',(-12.4222484974039,-44.7597320179364,910.));
#276077=CARTESIAN_POINT('Origin',(-13.0586446004718,-45.3961281210043,910.));
#276078=CARTESIAN_POINT('',(-12.1586446004719,-45.3961281210044,1282.35584962783));
#276079=CARTESIAN_POINT('Origin',(-13.0586446004719,-45.3961281210044,1282.35584962783));
#276080=CARTESIAN_POINT('',(-12.1586446004716,-45.3961281210041,-260.));
#276081=CARTESIAN_POINT('Origin',(-13.0586446004716,-45.3961281210041,-260.));
#276082=CARTESIAN_POINT('',(-12.1586446004718,-45.3961281210043,910.));
#276083=CARTESIAN_POINT('Origin',(-12.1586446004718,-49.1313553995291,910.));
#276084=CARTESIAN_POINT('',(-12.1586446004719,-49.1313553995291,1282.35584962783));
#276085=CARTESIAN_POINT('',(-12.1586446004719,-49.1313553995291,1282.35584962783));
#276086=CARTESIAN_POINT('',(-12.1586446004716,-49.1313553995289,-260.));
#276087=CARTESIAN_POINT('',(-12.1586446004716,-49.1313553995289,-260.));
#276088=CARTESIAN_POINT('',(-12.1586446004718,-49.1313553995291,910.));
#276089=CARTESIAN_POINT('Origin',(-13.0586446004718,-49.1313553995291,910.));
#276090=CARTESIAN_POINT('',(-13.0586446004719,-50.0313553995291,1282.35584962783));
#276091=CARTESIAN_POINT('Origin',(-13.0586446004719,-49.1313553995291,1282.35584962783));
#276092=CARTESIAN_POINT('',(-13.0586446004716,-50.0313553995288,-260.));
#276093=CARTESIAN_POINT('Origin',(-13.0586446004716,-49.1313553995288,-260.));
#276094=CARTESIAN_POINT('',(-13.0586446004718,-50.0313553995291,910.));
#276095=CARTESIAN_POINT('Origin',(-18.9086446004719,-50.031355399529,910.));
#276096=CARTESIAN_POINT('',(-18.9086446004719,-50.0313553995291,1282.35584962783));
#276097=CARTESIAN_POINT('',(-18.9086446004719,-50.0313553995291,1282.35584962783));
#276098=CARTESIAN_POINT('',(-18.9086446004716,-50.0313553995288,-260.));
#276099=CARTESIAN_POINT('',(-18.9086446004716,-50.0313553995288,-260.));
#276100=CARTESIAN_POINT('',(-18.9086446004719,-50.031355399529,910.));
#276101=CARTESIAN_POINT('Origin',(-18.9086446004719,-50.931355399529,910.));
#276102=CARTESIAN_POINT('',(-19.8086446004719,-50.9313553995291,1282.35584962783));
#276103=CARTESIAN_POINT('Origin',(-18.9086446004719,-50.9313553995291,1282.35584962783));
#276104=CARTESIAN_POINT('',(-19.8086446004716,-50.9313553995288,-260.));
#276105=CARTESIAN_POINT('Origin',(-18.9086446004716,-50.9313553995288,-260.));
#276106=CARTESIAN_POINT('',(-19.8086446004719,-50.931355399529,910.));
#276107=CARTESIAN_POINT('Origin',(-19.8086446004719,-53.001355399529,910.));
#276108=CARTESIAN_POINT('',(-19.8086446004719,-53.0013553995291,1282.35584962783));
#276109=CARTESIAN_POINT('',(-19.8086446004719,-53.001355399529,1282.35584962783));
#276110=CARTESIAN_POINT('',(-19.8086446004719,-53.0013553995288,-260.));
#276111=CARTESIAN_POINT('',(-19.8086446004717,-53.0013553995288,-260.));
#276112=CARTESIAN_POINT('',(-19.8086446004719,-53.001355399529,910.));
#276113=CARTESIAN_POINT('Origin',(-18.8186446004719,-53.001355399529,910.));
#276114=CARTESIAN_POINT('',(-18.8186446004719,-53.0013553995291,1282.35584962783));
#276115=CARTESIAN_POINT('',(-18.8186446004719,-53.0013553995291,1282.35584962783));
#276116=CARTESIAN_POINT('',(-18.8186446004717,-53.0013553995288,-260.));
#276117=CARTESIAN_POINT('',(-18.8186446004717,-53.0013553995288,-260.));
#276118=CARTESIAN_POINT('',(-18.8186446004719,-53.001355399529,910.));
#276119=CARTESIAN_POINT('Origin',(-18.8186446004719,-53.991355399529,910.));
#276120=CARTESIAN_POINT('',(-18.818644600472,-53.991355399529,1282.35584962783));
#276121=CARTESIAN_POINT('',(-18.8186446004717,-53.9913553995288,-260.));
#276122=CARTESIAN_POINT('Origin',(-54.0086446004715,-18.8013553995285,910.));
#276123=CARTESIAN_POINT('',(-53.0186446004715,-18.8013553995285,1282.35584962783));
#276124=CARTESIAN_POINT('',(-54.0086446004715,-18.8013553995285,1282.35584962783));
#276125=CARTESIAN_POINT('',(-53.0186446004712,-18.8013553995283,-260.));
#276126=CARTESIAN_POINT('',(-54.0086446004712,-18.8013553995282,-260.));
#276127=CARTESIAN_POINT('',(-53.0186446004714,-18.8013553995285,910.));
#276128=CARTESIAN_POINT('Origin',(-53.0186446004714,-18.8013553995285,910.));
#276129=CARTESIAN_POINT('',(-53.0186446004715,-19.7913553995285,1282.35584962783));
#276130=CARTESIAN_POINT('',(-53.0186446004715,-18.8013553995285,1282.35584962783));
#276131=CARTESIAN_POINT('',(-53.0186446004715,-19.7913553995283,-260.));
#276132=CARTESIAN_POINT('',(-53.0186446004712,-18.8013553995283,-260.));
#276133=CARTESIAN_POINT('',(-53.0186446004715,-19.7913553995285,910.));
#276134=CARTESIAN_POINT('Origin',(-53.0186446004715,-19.7913553995285,910.));
#276135=CARTESIAN_POINT('',(-50.9486446004715,-19.7913553995286,1282.35584962783));
#276136=CARTESIAN_POINT('',(-53.0186446004715,-19.7913553995285,1282.35584962783));
#276137=CARTESIAN_POINT('',(-50.9486446004712,-19.7913553995283,-260.));
#276138=CARTESIAN_POINT('',(-53.0186446004712,-19.7913553995283,-260.));
#276139=CARTESIAN_POINT('',(-50.9486446004715,-19.7913553995285,910.));
#276140=CARTESIAN_POINT('Origin',(-50.9486446004714,-18.8913553995285,910.));
#276141=CARTESIAN_POINT('',(-50.0486446004715,-18.8913553995286,1282.35584962783));
#276142=CARTESIAN_POINT('Origin',(-50.9486446004715,-18.8913553995286,1282.35584962783));
#276143=CARTESIAN_POINT('',(-50.0486446004712,-18.8913553995285,-260.));
#276144=CARTESIAN_POINT('Origin',(-50.9486446004712,-18.8913553995283,-260.));
#276145=CARTESIAN_POINT('',(-50.0486446004714,-18.8913553995285,910.));
#276146=CARTESIAN_POINT('Origin',(-50.0486446004714,-18.8913553995285,910.));
#276147=CARTESIAN_POINT('',(-50.0486446004714,-13.0413553995286,1282.35584962783));
#276148=CARTESIAN_POINT('',(-50.0486446004715,-18.8913553995285,1282.35584962783));
#276149=CARTESIAN_POINT('',(-50.0486446004711,-13.0413553995283,-260.));
#276150=CARTESIAN_POINT('',(-50.0486446004712,-18.8913553995283,-260.));
#276151=CARTESIAN_POINT('',(-50.0486446004713,-13.0413553995285,910.));
#276152=CARTESIAN_POINT('Origin',(-49.1486446004713,-13.0413553995285,910.));
#276153=CARTESIAN_POINT('',(-49.1486446004714,-12.1413553995286,1282.35584962783));
#276154=CARTESIAN_POINT('Origin',(-49.1486446004714,-13.0413553995286,1282.35584962783));
#276155=CARTESIAN_POINT('',(-49.1486446004713,-12.1413553995283,-260.));
#276156=CARTESIAN_POINT('Origin',(-49.1486446004711,-13.0413553995283,-260.));
#276157=CARTESIAN_POINT('',(-49.1486446004713,-12.1413553995285,910.));
#276158=CARTESIAN_POINT('Origin',(-49.1486446004713,-12.1413553995285,910.));
#276159=CARTESIAN_POINT('',(-45.4134173219466,-12.1413553995287,1282.35584962783));
#276160=CARTESIAN_POINT('',(-49.1486446004713,-12.1413553995286,1282.35584962783));
#276161=CARTESIAN_POINT('',(-45.4134173219464,-12.1413553995284,-260.));
#276162=CARTESIAN_POINT('',(-49.1486446004711,-12.1413553995283,-260.));
#276163=CARTESIAN_POINT('',(-45.4134173219466,-12.1413553995286,910.));
#276164=CARTESIAN_POINT('Origin',(-45.4134173219466,-13.0413553995286,910.));
#276165=CARTESIAN_POINT('',(-44.7770212188788,-12.4049592964608,1282.35584962783));
#276166=CARTESIAN_POINT('Origin',(-45.4134173219467,-13.0413553995287,1282.35584962783));
#276167=CARTESIAN_POINT('',(-44.7770212188785,-12.4049592964605,-260.));
#276168=CARTESIAN_POINT('Origin',(-45.4134173219464,-13.0413553995284,-260.));
#276169=CARTESIAN_POINT('',(-44.7770212188787,-12.4049592964607,910.));
#276170=CARTESIAN_POINT('Origin',(-44.7770212188787,-12.4049592964607,910.));
#276171=CARTESIAN_POINT('',(-38.0722484974036,-19.1097320179362,1282.35584962783));
#276172=CARTESIAN_POINT('',(-44.7770212188788,-12.4049592964608,1282.35584962783));
#276173=CARTESIAN_POINT('',(-38.0722484974034,-19.1097320179359,-260.));
#276174=CARTESIAN_POINT('',(-44.7770212188785,-12.4049592964605,-260.));
#276175=CARTESIAN_POINT('',(-38.0722484974036,-19.1097320179361,910.));
#276176=CARTESIAN_POINT('Origin',(-38.7086446004715,-19.746128121004,910.));
#276177=CARTESIAN_POINT('',(-37.8086446004715,-19.7461281210041,1282.35584962783));
#276178=CARTESIAN_POINT('Origin',(-38.7086446004715,-19.746128121004,1282.35584962783));
#276179=CARTESIAN_POINT('',(-37.8086446004713,-19.7461281210038,-260.));
#276180=CARTESIAN_POINT('Origin',(-38.7086446004712,-19.7461281210038,-260.));
#276181=CARTESIAN_POINT('',(-37.8086446004715,-19.746128121004,910.));
#276182=CARTESIAN_POINT('Origin',(-37.8086446004715,-19.746128121004,910.));
#276183=CARTESIAN_POINT('',(-37.8086446004716,-25.4699219701603,1282.35584962783));
#276184=CARTESIAN_POINT('',(-37.8086446004715,-19.746128121004,1282.35584962783));
#276185=CARTESIAN_POINT('',(-37.8086446004714,-25.46992197016,-260.));
#276186=CARTESIAN_POINT('',(-37.8086446004713,-19.7461281210038,-260.));
#276187=CARTESIAN_POINT('',(-37.8086446004716,-25.4699219701603,910.));
#276188=CARTESIAN_POINT('Origin',(-37.8086446004716,-25.4699219701603,910.));
#276189=CARTESIAN_POINT('',(-36.9302446004717,-26.9913553995289,1282.35584962783));
#276190=CARTESIAN_POINT('',(-37.8086446004717,-25.4699219701603,1282.35584962783));
#276191=CARTESIAN_POINT('',(-36.9302446004714,-26.9913553995286,-260.));
#276192=CARTESIAN_POINT('',(-37.8086446004714,-25.46992197016,-260.));
#276193=CARTESIAN_POINT('',(-36.9302446004716,-26.9913553995288,910.));
#276194=CARTESIAN_POINT('Origin',(-37.8086446004716,-28.5127888288973,910.));
#276195=CARTESIAN_POINT('',(-37.8086446004717,-28.5127888288974,1282.35584962783));
#276196=CARTESIAN_POINT('',(-37.8086446004716,-28.5127888288973,1282.35584962783));
#276197=CARTESIAN_POINT('',(-37.8086446004714,-28.5127888288971,-260.));
#276198=CARTESIAN_POINT('',(-37.8086446004714,-28.5127888288971,-260.));
#276199=CARTESIAN_POINT('',(-37.8086446004716,-28.5127888288973,910.));
#276200=CARTESIAN_POINT('Origin',(-37.8086446004717,-34.2365826780536,910.));
#276201=CARTESIAN_POINT('',(-37.8086446004717,-34.2365826780536,1282.35584962783));
#276202=CARTESIAN_POINT('',(-37.8086446004717,-34.2365826780536,1282.35584962783));
#276203=CARTESIAN_POINT('',(-37.8086446004715,-34.2365826780534,-260.));
#276204=CARTESIAN_POINT('',(-37.8086446004715,-34.2365826780534,-260.));
#276205=CARTESIAN_POINT('',(-37.8086446004717,-34.2365826780536,910.));
#276206=CARTESIAN_POINT('Origin',(-38.7086446004717,-34.2365826780536,910.));
#276207=CARTESIAN_POINT('',(-38.0722484974039,-34.8729787811215,1282.35584962783));
#276208=CARTESIAN_POINT('Origin',(-38.7086446004717,-34.2365826780536,1282.35584962783));
#276209=CARTESIAN_POINT('',(-38.0722484974036,-34.8729787811212,-260.));
#276210=CARTESIAN_POINT('Origin',(-38.7086446004715,-34.2365826780534,-260.));
#276211=CARTESIAN_POINT('',(-38.0722484974038,-34.8729787811215,910.));
#276212=CARTESIAN_POINT('Origin',(-44.7770212188791,-41.5777515025966,910.));
#276213=CARTESIAN_POINT('',(-44.7770212188792,-41.5777515025967,1282.35584962783));
#276214=CARTESIAN_POINT('',(-44.7770212188791,-41.5777515025966,1282.35584962783));
#276215=CARTESIAN_POINT('',(-44.7770212188789,-41.5777515025964,-260.));
#276216=CARTESIAN_POINT('',(-44.7770212188789,-41.5777515025964,-260.));
#276217=CARTESIAN_POINT('',(-44.7770212188791,-41.5777515025966,910.));
#276218=CARTESIAN_POINT('Origin',(-45.413417321947,-40.9413553995287,910.));
#276219=CARTESIAN_POINT('',(-45.4134173219471,-41.8413553995288,1282.35584962783));
#276220=CARTESIAN_POINT('Origin',(-45.4134173219471,-40.9413553995288,1282.35584962783));
#276221=CARTESIAN_POINT('',(-45.4134173219468,-41.8413553995285,-260.));
#276222=CARTESIAN_POINT('Origin',(-45.4134173219468,-40.9413553995285,-260.));
#276223=CARTESIAN_POINT('',(-45.413417321947,-41.8413553995287,910.));
#276224=CARTESIAN_POINT('Origin',(-49.1486446004717,-41.8413553995287,910.));
#276225=CARTESIAN_POINT('',(-49.1486446004718,-41.8413553995288,1282.35584962783));
#276226=CARTESIAN_POINT('',(-49.1486446004717,-41.8413553995288,1282.35584962783));
#276227=CARTESIAN_POINT('',(-49.1486446004715,-41.8413553995285,-260.));
#276228=CARTESIAN_POINT('',(-49.1486446004715,-41.8413553995285,-260.));
#276229=CARTESIAN_POINT('',(-49.1486446004717,-41.8413553995287,910.));
#276230=CARTESIAN_POINT('Origin',(-49.1486446004717,-40.9413553995287,910.));
#276231=CARTESIAN_POINT('',(-50.0486446004718,-40.9413553995288,1282.35584962783));
#276232=CARTESIAN_POINT('Origin',(-49.1486446004718,-40.9413553995288,1282.35584962783));
#276233=CARTESIAN_POINT('',(-50.0486446004715,-40.9413553995287,-260.));
#276234=CARTESIAN_POINT('Origin',(-49.1486446004715,-40.9413553995285,-260.));
#276235=CARTESIAN_POINT('',(-50.0486446004717,-40.9413553995287,910.));
#276236=CARTESIAN_POINT('Origin',(-50.0486446004717,-35.0913553995287,910.));
#276237=CARTESIAN_POINT('',(-50.0486446004717,-35.0913553995288,1282.35584962783));
#276238=CARTESIAN_POINT('',(-50.0486446004717,-35.0913553995287,1282.35584962783));
#276239=CARTESIAN_POINT('',(-50.0486446004715,-35.0913553995285,-260.));
#276240=CARTESIAN_POINT('',(-50.0486446004715,-35.0913553995285,-260.));
#276241=CARTESIAN_POINT('',(-50.0486446004717,-35.0913553995287,910.));
#276242=CARTESIAN_POINT('Origin',(-50.9486446004717,-35.0913553995287,910.));
#276243=CARTESIAN_POINT('',(-50.9486446004717,-34.1913553995288,1282.35584962783));
#276244=CARTESIAN_POINT('Origin',(-50.9486446004717,-35.0913553995288,1282.35584962783));
#276245=CARTESIAN_POINT('',(-50.9486446004714,-34.1913553995285,-260.));
#276246=CARTESIAN_POINT('Origin',(-50.9486446004715,-35.0913553995285,-260.));
#276247=CARTESIAN_POINT('',(-50.9486446004717,-34.1913553995287,910.));
#276248=CARTESIAN_POINT('Origin',(-53.0186446004717,-34.1913553995287,910.));
#276249=CARTESIAN_POINT('',(-53.0186446004717,-34.1913553995287,1282.35584962783));
#276250=CARTESIAN_POINT('',(-53.0186446004717,-34.1913553995287,1282.35584962783));
#276251=CARTESIAN_POINT('',(-53.0186446004715,-34.1913553995285,-260.));
#276252=CARTESIAN_POINT('',(-53.0186446004715,-34.1913553995285,-260.));
#276253=CARTESIAN_POINT('',(-53.0186446004717,-34.1913553995287,910.));
#276254=CARTESIAN_POINT('Origin',(-53.0186446004717,-35.1813553995287,910.));
#276255=CARTESIAN_POINT('',(-53.0186446004717,-35.1813553995287,1282.35584962783));
#276256=CARTESIAN_POINT('',(-53.0186446004717,-35.1813553995287,1282.35584962783));
#276257=CARTESIAN_POINT('',(-53.0186446004715,-35.1813553995284,-260.));
#276258=CARTESIAN_POINT('',(-53.0186446004715,-35.1813553995284,-260.));
#276259=CARTESIAN_POINT('',(-53.0186446004717,-35.1813553995287,910.));
#276260=CARTESIAN_POINT('Origin',(-54.0086446004717,-35.1813553995286,910.));
#276261=CARTESIAN_POINT('',(-54.0086446004717,-35.1813553995287,1282.35584962783));
#276262=CARTESIAN_POINT('',(-54.0086446004717,-35.1813553995287,1282.35584962783));
#276263=CARTESIAN_POINT('',(-54.0086446004715,-35.1813553995284,-260.));
#276264=CARTESIAN_POINT('',(-54.0086446004715,-35.1813553995284,-260.));
#276265=CARTESIAN_POINT('',(-54.0086446004717,-35.1813553995286,910.));
#276266=CARTESIAN_POINT('Origin',(-54.0086446004717,-35.1813553995286,910.));
#276267=CARTESIAN_POINT('',(-54.0086446004719,-50.3337553995287,1282.35584962783));
#276268=CARTESIAN_POINT('',(-54.0086446004717,-35.1813553995286,1282.35584962783));
#276269=CARTESIAN_POINT('',(-54.0086446004716,-50.3337553995284,-260.));
#276270=CARTESIAN_POINT('',(-54.0086446004715,-35.1813553995284,-260.));
#276271=CARTESIAN_POINT('',(-54.0086446004718,-50.3337553995286,910.));
#276272=CARTESIAN_POINT('Origin',(-50.3510446004718,-50.3337553995286,910.));
#276273=CARTESIAN_POINT('',(-50.3510446004719,-53.9913553995288,1282.35584962783));
#276274=CARTESIAN_POINT('Origin',(-50.3510446004719,-50.3337553995287,1282.35584962783));
#276275=CARTESIAN_POINT('',(-50.3510446004718,-53.9913553995285,-260.));
#276276=CARTESIAN_POINT('Origin',(-50.3510446004716,-50.3337553995284,-260.));
#276277=CARTESIAN_POINT('',(-50.3510446004718,-53.9913553995287,910.));
#276278=CARTESIAN_POINT('Origin',(-35.1986446004719,-53.9913553995289,910.));
#276279=CARTESIAN_POINT('',(-35.198644600472,-53.9913553995289,1282.35584962783));
#276280=CARTESIAN_POINT('',(-35.1986446004719,-53.9913553995289,1282.35584962783));
#276281=CARTESIAN_POINT('',(-35.1986446004717,-53.9913553995289,-260.));
#276282=CARTESIAN_POINT('',(-35.1986446004717,-53.9913553995286,-260.));
#276283=CARTESIAN_POINT('',(-35.1986446004719,-53.9913553995289,910.));
#276284=CARTESIAN_POINT('Origin',(-35.1986446004719,-53.9913553995289,910.));
#276285=CARTESIAN_POINT('',(-35.1986446004719,-53.0013553995289,1282.35584962783));
#276286=CARTESIAN_POINT('',(-35.198644600472,-53.9913553995289,1282.35584962783));
#276287=CARTESIAN_POINT('',(-35.1986446004719,-53.0013553995286,-260.));
#276288=CARTESIAN_POINT('',(-35.1986446004717,-53.9913553995286,-260.));
#276289=CARTESIAN_POINT('',(-35.1986446004719,-53.0013553995288,910.));
#276290=CARTESIAN_POINT('Origin',(-35.1986446004719,-53.0013553995288,910.));
#276291=CARTESIAN_POINT('',(-34.2086446004719,-53.0013553995289,1282.35584962783));
#276292=CARTESIAN_POINT('',(-35.1986446004719,-53.0013553995289,1282.35584962783));
#276293=CARTESIAN_POINT('',(-34.2086446004717,-53.0013553995288,-260.));
#276294=CARTESIAN_POINT('',(-35.1986446004717,-53.0013553995286,-260.));
#276295=CARTESIAN_POINT('',(-34.2086446004719,-53.0013553995288,910.));
#276296=CARTESIAN_POINT('Origin',(-34.2086446004719,-53.0013553995288,910.));
#276297=CARTESIAN_POINT('',(-34.2086446004719,-50.9313553995289,1282.35584962783));
#276298=CARTESIAN_POINT('',(-34.2086446004719,-53.0013553995288,1282.35584962783));
#276299=CARTESIAN_POINT('',(-34.2086446004716,-50.9313553995286,-260.));
#276300=CARTESIAN_POINT('',(-34.2086446004717,-53.0013553995286,-260.));
#276301=CARTESIAN_POINT('',(-34.2086446004718,-50.9313553995289,910.));
#276302=CARTESIAN_POINT('Origin',(-35.1086446004718,-50.9313553995288,910.));
#276303=CARTESIAN_POINT('',(-35.1086446004719,-50.0313553995289,1282.35584962783));
#276304=CARTESIAN_POINT('Origin',(-35.1086446004719,-50.9313553995289,1282.35584962783));
#276305=CARTESIAN_POINT('',(-35.1086446004716,-50.0313553995286,-260.));
#276306=CARTESIAN_POINT('Origin',(-35.1086446004716,-50.9313553995286,-260.));
#276307=CARTESIAN_POINT('',(-35.1086446004718,-50.0313553995288,910.));
#276308=CARTESIAN_POINT('Origin',(-35.1086446004718,-50.0313553995288,910.));
#276309=CARTESIAN_POINT('',(-40.9586446004719,-50.0313553995288,1282.35584962783));
#276310=CARTESIAN_POINT('',(-35.1086446004718,-50.0313553995289,1282.35584962783));
#276311=CARTESIAN_POINT('',(-40.9586446004716,-50.0313553995286,-260.));
#276312=CARTESIAN_POINT('',(-35.1086446004716,-50.0313553995286,-260.));
#276313=CARTESIAN_POINT('',(-40.9586446004718,-50.0313553995288,910.));
#276314=CARTESIAN_POINT('Origin',(-40.9586446004718,-49.1313553995288,910.));
#276315=CARTESIAN_POINT('',(-41.8586446004719,-49.1313553995288,1282.35584962783));
#276316=CARTESIAN_POINT('Origin',(-40.9586446004719,-49.1313553995288,1282.35584962783));
#276317=CARTESIAN_POINT('',(-41.8586446004716,-49.1313553995288,-260.));
#276318=CARTESIAN_POINT('Origin',(-40.9586446004716,-49.1313553995286,-260.));
#276319=CARTESIAN_POINT('',(-41.8586446004718,-49.1313553995288,910.));
#276320=CARTESIAN_POINT('Origin',(-41.8586446004718,-49.1313553995288,910.));
#276321=CARTESIAN_POINT('',(-41.8586446004719,-45.3961281210041,1282.35584962783));
#276322=CARTESIAN_POINT('',(-41.8586446004719,-49.1313553995288,1282.35584962783));
#276323=CARTESIAN_POINT('',(-41.8586446004716,-45.3961281210038,-260.));
#276324=CARTESIAN_POINT('',(-41.8586446004716,-49.1313553995285,-260.));
#276325=CARTESIAN_POINT('',(-41.8586446004718,-45.396128121004,910.));
#276326=CARTESIAN_POINT('Origin',(-40.9586446004718,-45.396128121004,910.));
#276327=CARTESIAN_POINT('',(-41.5950407035397,-44.7597320179362,1282.35584962783));
#276328=CARTESIAN_POINT('Origin',(-40.9586446004719,-45.3961281210041,1282.35584962783));
#276329=CARTESIAN_POINT('',(-41.5950407035397,-44.7597320179361,-260.));
#276330=CARTESIAN_POINT('Origin',(-40.9586446004716,-45.3961281210038,-260.));
#276331=CARTESIAN_POINT('',(-41.5950407035397,-44.7597320179361,910.));
#276332=CARTESIAN_POINT('Origin',(-41.5950407035397,-44.7597320179361,910.));
#276333=CARTESIAN_POINT('',(-34.8902679820644,-38.054959296461,1282.35584962783));
#276334=CARTESIAN_POINT('',(-41.5950407035397,-44.7597320179361,1282.35584962783));
#276335=CARTESIAN_POINT('',(-34.8902679820641,-38.0549592964607,-260.));
#276336=CARTESIAN_POINT('',(-41.5950407035395,-44.7597320179359,-260.));
#276337=CARTESIAN_POINT('',(-34.8902679820644,-38.054959296461,910.));
#276338=CARTESIAN_POINT('Origin',(-34.2538718789965,-38.6913553995289,910.));
#276339=CARTESIAN_POINT('',(-34.2538718789965,-37.7913553995289,1282.35584962783));
#276340=CARTESIAN_POINT('Origin',(-34.2538718789965,-38.6913553995289,1282.35584962783));
#276341=CARTESIAN_POINT('',(-34.2538718789965,-37.7913553995286,-260.));
#276342=CARTESIAN_POINT('Origin',(-34.2538718789963,-38.6913553995287,-260.));
#276343=CARTESIAN_POINT('',(-34.2538718789965,-37.7913553995289,910.));
#276344=CARTESIAN_POINT('Origin',(-34.2538718789965,-37.7913553995289,910.));
#276345=CARTESIAN_POINT('',(-34.2538718789965,-37.7913553995289,1282.35584962783));
#276346=CARTESIAN_POINT('',(-34.2538718789963,-37.7913553995286,-260.));
#276347=CARTESIAN_POINT('Origin',(-50.0486446004712,39.1586446004713,-260.0000216));
#276348=CARTESIAN_POINT('',(-50.8586446004712,38.3486446004714,1282.35584962783));
#276349=CARTESIAN_POINT('',(-50.0486446004712,39.1586446004713,1282.35584962783));
#276350=CARTESIAN_POINT('',(-50.8586446004712,38.3486446004714,-260.));
#276351=CARTESIAN_POINT('',(-50.8586446004712,38.3486446004714,-260.0000216));
#276352=CARTESIAN_POINT('',(-54.0762582397336,35.131030961209,-260.));
#276353=CARTESIAN_POINT('Origin',(-50.8586446004712,38.3486446004714,-260.0000216));
#276354=CARTESIAN_POINT('',(-50.8586446004712,38.3486446004714,1282.35584962783));
#276355=CARTESIAN_POINT('',(-35.4910309612088,22.9810309612089,-260.));
#276356=CARTESIAN_POINT('Origin',(-39.1586446004713,50.0486446004712,-260.0000216));
#276357=CARTESIAN_POINT('',(-38.3486446004713,50.8586446004712,1282.35584962783));
#276358=CARTESIAN_POINT('',(-39.1586446004713,50.0486446004712,1282.35584962783));
#276359=CARTESIAN_POINT('',(-38.3486446004713,50.8586446004712,-260.));
#276360=CARTESIAN_POINT('',(-54.0762582397337,35.1310309612087,-260.));
#276361=CARTESIAN_POINT('',(-38.3486446004713,50.8586446004712,-260.0000216));
#276362=CARTESIAN_POINT('Origin',(-38.3486446004713,50.8586446004712,-260.0000216));
#276363=CARTESIAN_POINT('',(-38.3486446004713,50.8586446004712,1282.35584962783));
#276364=CARTESIAN_POINT('',(-22.981030961209,35.4910309612087,-260.));
#276365=CARTESIAN_POINT('Origin',(0.,0.,-300.));
#276366=CARTESIAN_POINT('',(400.,-85.1426923911342,-300.));
#276367=CARTESIAN_POINT('',(400.,496.179570367622,-300.));
#276368=CARTESIAN_POINT('',(400.,0.,-300.));
#276369=CARTESIAN_POINT('',(-400.,-85.142692391134,-300.));
#276370=CARTESIAN_POINT('',(-1.03389319109141E-14,-85.1426923911341,-300.));
#276371=CARTESIAN_POINT('',(-400.,496.179570367622,-300.));
#276372=CARTESIAN_POINT('',(-400.,1.30395574000049E-13,-300.));
#276373=CARTESIAN_POINT('',(-266.14205645498,496.179570367622,-300.));
#276374=CARTESIAN_POINT('',(0.,496.179570367622,-300.));
#276375=CARTESIAN_POINT('',(-266.14205645498,85.1426923911342,-300.));
#276376=CARTESIAN_POINT('',(-266.14205645498,0.,-300.));
#276377=CARTESIAN_POINT('',(266.142056454979,85.1426923911341,-300.));
#276378=CARTESIAN_POINT('',(1.03389319109141E-14,85.1426923911341,-300.));
#276379=CARTESIAN_POINT('',(266.142056454979,496.179570367622,-300.));
#276380=CARTESIAN_POINT('',(266.142056454979,0.,-300.));
#276381=CARTESIAN_POINT('',(0.,496.179570367622,-300.));
#276382=CARTESIAN_POINT('Origin',(0.,496.179570367622,-300.));
#276383=CARTESIAN_POINT('',(400.,496.179570367622,-260.));
#276384=CARTESIAN_POINT('',(266.142056454979,496.179570367622,-260.));
#276385=CARTESIAN_POINT('',(0.,496.179570367622,-260.));
#276386=CARTESIAN_POINT('',(400.,496.179570367622,-300.));
#276387=CARTESIAN_POINT('',(266.142056454979,496.179570367622,-300.));
#276388=CARTESIAN_POINT('Origin',(266.142056454979,0.,-300.));
#276389=CARTESIAN_POINT('',(266.142056454979,85.1426923911341,-260.));
#276390=CARTESIAN_POINT('',(266.142056454979,0.,-260.));
#276391=CARTESIAN_POINT('',(266.142056454979,85.1426923911341,-300.));
#276392=CARTESIAN_POINT('Origin',(1.03389319109141E-14,85.1426923911341,
-300.));
#276393=CARTESIAN_POINT('',(-266.14205645498,85.1426923911342,-260.));
#276394=CARTESIAN_POINT('',(1.03389319109141E-14,85.1426923911341,-260.));
#276395=CARTESIAN_POINT('',(-266.14205645498,85.1426923911342,-300.));
#276396=CARTESIAN_POINT('Origin',(-266.14205645498,0.,-300.));
#276397=CARTESIAN_POINT('',(-266.14205645498,496.179570367622,-260.));
#276398=CARTESIAN_POINT('',(-266.14205645498,0.,-260.));
#276399=CARTESIAN_POINT('',(-266.14205645498,496.179570367622,-300.));
#276400=CARTESIAN_POINT('Origin',(0.,496.179570367622,-300.));
#276401=CARTESIAN_POINT('',(-400.,496.179570367622,-260.));
#276402=CARTESIAN_POINT('',(0.,496.179570367622,-260.));
#276403=CARTESIAN_POINT('',(-400.,496.179570367622,-300.));
#276404=CARTESIAN_POINT('Origin',(-400.,1.30395574000049E-13,-300.));
#276405=CARTESIAN_POINT('',(-400.,-85.142692391134,-260.));
#276406=CARTESIAN_POINT('',(-400.,1.30395574000049E-13,-260.));
#276407=CARTESIAN_POINT('',(-400.,-85.142692391134,-300.));
#276408=CARTESIAN_POINT('Origin',(-1.03389319109141E-14,-85.1426923911341,
-300.));
#276409=CARTESIAN_POINT('',(400.,-85.1426923911342,-260.));
#276410=CARTESIAN_POINT('',(-1.03389319109141E-14,-85.1426923911341,-260.));
#276411=CARTESIAN_POINT('',(400.,-85.1426923911342,-300.));
#276412=CARTESIAN_POINT('Origin',(400.,0.,-300.));
#276413=CARTESIAN_POINT('',(400.,0.,-260.));
#276414=CARTESIAN_POINT('Origin',(0.,0.,-260.));
#276415=CARTESIAN_POINT('Origin',(172.453871410095,236.609402635306,1282.35584962783));
#276416=CARTESIAN_POINT('',(172.453871410095,236.609402635306,1302.35584962783));
#276417=CARTESIAN_POINT('',(-172.453871410095,236.609402635306,1302.35584962783));
#276418=CARTESIAN_POINT('',(172.453871410095,236.609402635306,1302.35584962783));
#276419=CARTESIAN_POINT('',(172.453871410095,236.609402635306,1282.35584962783));
#276420=CARTESIAN_POINT('',(172.453871410095,236.609402635306,1282.35584962783));
#276421=CARTESIAN_POINT('',(-172.453871410095,236.609402635306,1282.35584962783));
#276422=CARTESIAN_POINT('',(172.453871410095,236.609402635306,1282.35584962783));
#276423=CARTESIAN_POINT('',(-172.453871410095,236.609402635306,1282.35584962783));
#276424=CARTESIAN_POINT('Origin',(-172.453871410095,236.609402635306,1282.35584962783));
#276425=CARTESIAN_POINT('',(-172.453871410095,-114.916974471838,1302.35584962783));
#276426=CARTESIAN_POINT('',(-172.453871410095,236.609402635306,1302.35584962783));
#276427=CARTESIAN_POINT('',(-172.453871410095,-114.916974471838,1282.35584962783));
#276428=CARTESIAN_POINT('',(-172.453871410095,236.609402635306,1282.35584962783));
#276429=CARTESIAN_POINT('',(-172.453871410095,-114.916974471838,1282.35584962783));
#276430=CARTESIAN_POINT('Origin',(-172.453871410095,-114.916974471838,1282.35584962783));
#276431=CARTESIAN_POINT('',(172.453871410095,-114.916974471838,1302.35584962783));
#276432=CARTESIAN_POINT('',(-172.453871410095,-114.916974471838,1302.35584962783));
#276433=CARTESIAN_POINT('',(172.453871410095,-114.916974471838,1282.35584962783));
#276434=CARTESIAN_POINT('',(-172.453871410095,-114.916974471838,1282.35584962783));
#276435=CARTESIAN_POINT('',(172.453871410095,-114.916974471838,1282.35584962783));
#276436=CARTESIAN_POINT('Origin',(172.453871410095,236.609402635306,1282.35584962783));
#276437=CARTESIAN_POINT('',(172.453871410095,236.609402635306,1302.35584962783));
#276438=CARTESIAN_POINT('',(172.453871410095,236.609402635306,1282.35584962783));
#276439=CARTESIAN_POINT('Origin',(0.,0.,1282.35584962783));
#276440=CARTESIAN_POINT('Origin',(-38.7086446004713,19.7634173219464,1302.35584962783));
#276453=UNCERTAINTY_MEASURE_WITH_UNIT(LENGTH_MEASURE(0.01),#276463,
'DISTANCE_ACCURACY_VALUE',
'Maximum model space distance between geometric entities at asserted c
onnectivities');
#276454=UNCERTAINTY_MEASURE_WITH_UNIT(LENGTH_MEASURE(0.01),#276463,
'DISTANCE_ACCURACY_VALUE',
'Maximum model space distance between geometric entities at asserted c
onnectivities');
#276461=(
GEOMETRIC_REPRESENTATION_CONTEXT(3)
GLOBAL_UNCERTAINTY_ASSIGNED_CONTEXT((#276453))
GLOBAL_UNIT_ASSIGNED_CONTEXT((#276463,#276465,#276466))
REPRESENTATION_CONTEXT('','3D')
);
#276462=(
GEOMETRIC_REPRESENTATION_CONTEXT(3)
GLOBAL_UNCERTAINTY_ASSIGNED_CONTEXT((#276454))
GLOBAL_UNIT_ASSIGNED_CONTEXT((#276463,#276465,#276466))
REPRESENTATION_CONTEXT('','3D')
);
#276463=(
LENGTH_UNIT()
NAMED_UNIT(*)
SI_UNIT(.MILLI.,.METRE.)
);
#276465=(
NAMED_UNIT(*)
PLANE_ANGLE_UNIT()
SI_UNIT($,.RADIAN.)
);
#276466=(
NAMED_UNIT(*)
SI_UNIT($,.STERADIAN.)
SOLID_ANGLE_UNIT()
);
#276473=SHAPE_DEFINITION_REPRESENTATION(#276480,#276493);
#276480=PRODUCT_DEFINITION_SHAPE('',$,#276501);
#276493=SHAPE_REPRESENTATION('',(#110986),#276461);
#276494=PRODUCT_DEFINITION_CONTEXT('part definition',#276517,'design');
#276501=PRODUCT_DEFINITION('support gantry arm_5537T808',
'support gantry arm',#276508,#276494);
#276508=PRODUCT_DEFINITION_FORMATION('',$,#276525);
#276517=APPLICATION_CONTEXT(
'Core Data for Automotive Mechanical Design Process');
#276518=PRODUCT_CONTEXT('part definition',#276517,'mechanical');
#276525=PRODUCT('support gantry arm_5537T808','support gantry arm',$,(#276518));
#276527=PRESENTATION_STYLE_ASSIGNMENT((#276532));
#276532=SURFACE_STYLE_USAGE(.BOTH.,#276537);
#276537=SURFACE_SIDE_STYLE('',(#276542));
#276542=SURFACE_STYLE_FILL_AREA(#276547);
#276547=FILL_AREA_STYLE('Opaque(97,158,199)',(#276552));
#276552=FILL_AREA_STYLE_COLOUR('Opaque(97,158,199)',#276557);
#276557=COLOUR_RGB('Opaque(97,158,199)',0.380392156862745,0.619607843137255,
0.780392156862745);
ENDSEC;
END-ISO-10303-21;
